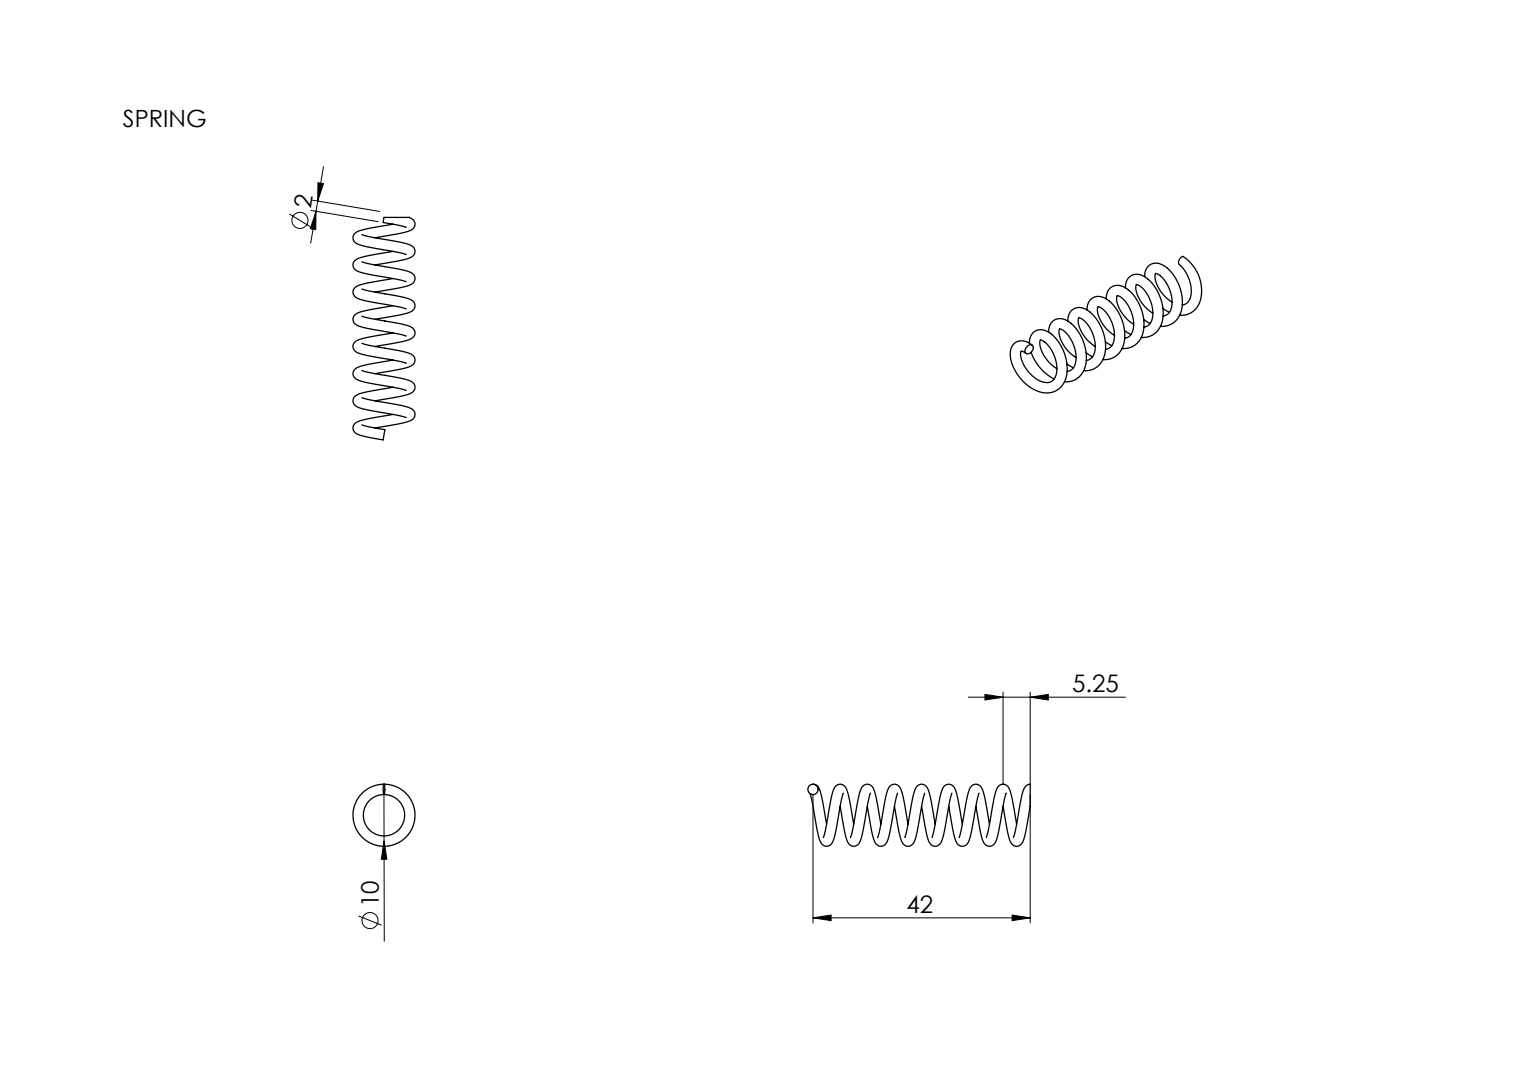
ISO-10303-21;
HEADER;
FILE_DESCRIPTION (('STEP AP214'),
    '1' );
FILE_NAME ('spring.step',
    '2026-10-08T14:41:38',
    ( '' ),
    ( '' ),
    'SwSTEP 2.0',
    'SolidWorks 2026',
    '' );
FILE_SCHEMA (( 'AUTOMOTIVE_DESIGN' ));
ENDSEC;

DATA;
#1=CARTESIAN_POINT ( 'NONE',  ( -12.68318583509882380, -26.07549068051207541, 23.95507249208304756 ) ) ;
#5=ORIENTED_EDGE ( 'NONE', *, *, #7068, .F. ) ;
#6=CARTESIAN_POINT ( 'NONE',  ( -14.83517299489738761, -20.99999999999997513, 4.263677507916960430 ) ) ;
#20=CARTESIAN_POINT ( 'NONE',  ( -16.17491895705301275, -18.95583473709189803, 14.54492750791695421 ) ) ;
#25=CARTESIAN_POINT ( 'NONE',  ( -17.64274437364858983, -19.75228648362910633, 21.54882249208304401 ) ) ;
#29=CARTESIAN_POINT ( 'NONE',  ( -17.35725562635140307, -28.41254052147349185, 40.79882249208304046 ) ) ;
#52=CARTESIAN_POINT ( 'NONE',  ( -10.75228648362910100, -26.64274437364854009, 6.013677507916958653 ) ) ;
#53=CARTESIAN_POINT ( 'NONE',  ( -19.41254052147348830, -26.35725562635142083, 18.26367750791695599 ) ) ;
#55=CARTESIAN_POINT ( 'NONE',  ( -13.49542703274174116, -28.95583473709188738, 3.392572492083040903 ) ) ;
#59=CARTESIAN_POINT ( 'NONE',  ( -13.82508104294698192, -29.04416526290806644, 1.419927507916958209 ) ) ;
#61=CARTESIAN_POINT ( 'NONE',  ( -15.16482700510259640, -28.99999999999998224, 1.638677507916958431 ) ) ;
#74=CARTESIAN_POINT ( 'NONE',  ( -7.999999999999996447, -23.83517299489733432, 23.29882249208304046 ) ) ;
#79=CARTESIAN_POINT ( 'NONE',  ( -15.63902057219076269, -20.95583473709189448, 9.294927507916961318 ) ) ;
#81=CARTESIAN_POINT ( 'NONE',  ( -21.14459132904239169, -20.64274437364858628, 5.361322492083039570 ) ) ;
#90=CARTESIAN_POINT ( 'NONE',  ( -15.00000000000001066, -19.99999999999997868, -4.814824860968089633E-32 ) ) ;
#98=CARTESIAN_POINT ( 'NONE',  ( -9.754982604823348780, -18.99630608921234654, 15.41992750791695777 ) ) ;
#103=CARTESIAN_POINT ( 'NONE',  ( -14.83517299489736985, -26.99999999999998579, 24.61132249208304756 ) ) ;
#107=CARTESIAN_POINT ( 'NONE',  ( -11.99999999999999289, -24.16482700510258752, 16.07617750791696309 ) ) ;
#119=PLANE ( 'NONE',  #7046 ) ;
#120=CARTESIAN_POINT ( 'NONE',  ( -19.95583473709191580, -22.49542703274176603, 13.66992750791695599 ) ) ;
#123=CARTESIAN_POINT ( 'NONE',  ( -16.50457296725825174, -19.04416526290807354, 16.51757249208304046 ) ) ;
#126=CARTESIAN_POINT ( 'NONE',  ( -14.83517299489736985, -26.99999999999998579, 19.36132249208304046 ) ) ;
#129=CARTESIAN_POINT ( 'NONE',  ( -11.21456601361727046, -19.57682413056721416, 1.010946030696228434E-16 ) ) ;
#144=CARTESIAN_POINT ( 'NONE',  ( -17.35725562635144215, -19.58745947852648683, 19.57617750791695954 ) ) ;
#146=CARTESIAN_POINT ( 'NONE',  ( -17.35725562635144215, -19.58745947852648683, 9.076177507916957765 ) ) ;
#149=CARTESIAN_POINT ( 'NONE',  ( -20.24501739517669563, -18.99630608921239627, 42.33007249208303335 ) ) ;
#151=CARTESIAN_POINT ( 'NONE',  ( -10.58745947852649927, -21.64274437364853654, -0.1113224920830418047 ) ) ;
#153=CARTESIAN_POINT ( 'NONE',  ( -12.35725562635143682, -19.75228648362908501, 20.45117750791695954 ) ) ;
#170=CARTESIAN_POINT ( 'NONE',  ( -22.04416526290809486, -22.28918265808477628, 15.64257249208304223 ) ) ;
#175=CARTESIAN_POINT ( 'NONE',  ( -18.04416526290808420, -24.63902057219074493, 18.48242750791695954 ) ) ;
#177=CARTESIAN_POINT ( 'NONE',  ( -7.999999999999996447, -23.83517299489733432, 7.548822492083037794 ) ) ;
#198=CARTESIAN_POINT ( 'NONE',  ( -20.97976432393977575, -20.35725562635143504, 13.88867750791695599 ) ) ;
#202=CARTESIAN_POINT ( 'NONE',  ( -13.64274437364857739, -21.31951028609534760, 11.92382249208304401 ) ) ;
#206=CARTESIAN_POINT ( 'NONE',  ( -15.96867458239597326, -26.95583473709190159, 17.60742750791696309 ) ) ;
#222=CARTESIAN_POINT ( 'NONE',  ( -10.04416526290807710, -25.50457296725819489, 21.54492750791695599 ) ) ;
#226=CARTESIAN_POINT ( 'NONE',  ( -19.95583473709190514, -25.50457296725822687, 15.20507249208304046 ) ) ;
#228=CARTESIAN_POINT ( 'NONE',  ( -17.07549068051208963, -26.31681416490115311, 25.26757249208305112 ) ) ;
#235=( BOUNDED_CURVE ( )  B_SPLINE_CURVE ( 2, ( #4277, #17906, #10238, #11607, #11805, #16129, #13075, #8674, #61, #14656, #4180, #7208, #16424, #14762, #1334, #10042, #1227, #16223, #2599, #7501, #2989, #1531, #2897, #2794, #14856, #14957, #8970, #6044, #13479, #16039, #8872, #13181, #1431, #8580, #19173, #17497, #1133, #19368, #4075, #5744, #11704, #5939, #14561, #7112, #8771, #7304, #13271, #5844, #17801, #4375, #10334, #11910, #16330, #7406, #18202, #8002, #16628, #18399, #15345, #16823, #3194, #18000, #9264, #6339, #12200, #9460, #9170, #1636, #352, #13969, #13671, #4779, #250, #10531, #6235, #18299, #7607, #12304, #1822, #4965, #10729, #542, #12001, #16524, #4867, #7801, #13772, #4574, #15251, #3386, #10827, #16725, #6140, #9355, #153, #1924, #7907, #15154, #3087, #9070, #13872, #10922, #3294, #16922, #447, #1723, #6432, #3485, #12399, #7704, #15446, #2013, #15057, #13572, #12101, #18097, #4670, #10626, #2113, #12596, #918, #14165, #17022, #6900, #17387, #6629, #11203, #15918, #2390, #3579, #9551, #5251, #14345, #2299, #5064, #17112, #8376, #3772, #12683, #18872, #12873, #18494, #17302, #3676, #3864, #15543, #8198, #8469, #8097, #5437, #3961, #18587, #14066, #8283, #9921, #14253, #638, #825, #11393, #17207, #9830, #2481, #734, #14445, #6528, #15823, #18686, #12493, #11115, #11020, #5154, #11304, #9646, #15633, #2205, #6808, #6713, #9745, #15737, #5341, #12773, #18769, #2674, #1205, #8657, #18960, #14638, #7289, #16022 ),
 .UNSPECIFIED., .F., .F. ) 
 B_SPLINE_CURVE_WITH_KNOTS ( ( 3, 2, 2, 2, 2, 2, 2, 2, 2, 2, 2, 2, 2, 2, 2, 2, 2, 2, 2, 2, 2, 2, 2, 2, 2, 2, 2, 2, 2, 2, 2, 2, 2, 2, 2, 2, 2, 2, 2, 2, 2, 2, 2, 2, 2, 2, 2, 2, 2, 2, 2, 2, 2, 2, 2, 2, 2, 2, 2, 2, 2, 2, 2, 2, 2, 2, 2, 2, 2, 2, 2, 2, 2, 2, 2, 2, 2, 2, 2, 2, 2, 2, 2, 2, 2, 2, 2, 2, 2, 2, 2, 2, 2, 2, 3 ),
 ( 0.02351720863160803449, 0.03125000000000000000, 0.04166666666666666435, 0.05208333333333333565, 0.06250000000000000000, 0.07291666666666665741, 0.08333333333333332871, 0.09375000000000000000, 0.1041666666666666574, 0.1145833333333333148, 0.1250000000000000000, 0.1354166666666666574, 0.1458333333333333426, 0.1562500000000000000, 0.1666666666666666574, 0.1770833333333333426, 0.1875000000000000000, 0.1979166666666666574, 0.2083333333333333426, 0.2187500000000000000, 0.2291666666666666574, 0.2395833333333333426, 0.2500000000000000000, 0.2604166666666666852, 0.2708333333333333148, 0.2812500000000000000, 0.2916666666666666852, 0.3020833333333333148, 0.3125000000000000000, 0.3229166666666666852, 0.3333333333333333148, 0.3437500000000000000, 0.3541666666666666852, 0.3645833333333333148, 0.3750000000000000000, 0.3854166666666666852, 0.3958333333333333148, 0.4062500000000000000, 0.4166666666666666852, 0.4270833333333333148, 0.4375000000000000000, 0.4479166666666666852, 0.4583333333333333148, 0.4687500000000000000, 0.4791666666666666852, 0.4895833333333333148, 0.5000000000000000000, 0.5104166666666666297, 0.5208333333333333703, 0.5312500000000000000, 0.5416666666666666297, 0.5520833333333333703, 0.5625000000000000000, 0.5729166666666666297, 0.5833333333333333703, 0.5937500000000000000, 0.6041666666666666297, 0.6145833333333333703, 0.6250000000000000000, 0.6354166666666666297, 0.6458333333333333703, 0.6562500000000000000, 0.6666666666666666297, 0.6770833333333333703, 0.6875000000000000000, 0.6979166666666666297, 0.7083333333333333703, 0.7187500000000000000, 0.7291666666666666297, 0.7395833333333333703, 0.7500000000000000000, 0.7604166666666666297, 0.7708333333333333703, 0.7812500000000000000, 0.7916666666666666297, 0.8020833333333333703, 0.8125000000000000000, 0.8229166666666666297, 0.8333333333333333703, 0.8437500000000000000, 0.8541666666666666297, 0.8645833333333333703, 0.8750000000000000000, 0.8854166666666666297, 0.8958333333333333703, 0.9062500000000000000, 0.9166666666666666297, 0.9270833333333333703, 0.9375000000000000000, 0.9479166666666666297, 0.9583333333333333703, 0.9687500000000000000, 0.9791666666666666297, 0.9895833333333333703, 1.000000000000000000 ),
 .UNSPECIFIED. ) 
 CURVE ( )  GEOMETRIC_REPRESENTATION_ITEM ( )  RATIONAL_B_SPLINE_CURVE ( ( 0.9869654386326103257, 0.9747051062697298374, 1.000000000000000000, 0.9659258262890683122, 1.000000000000000000, 0.9659258262890683122, 1.000000000000000000, 0.9659258262890683122, 1.000000000000000000, 0.9659258262890683122, 1.000000000000000000, 0.9659258262890683122, 1.000000000000000000, 0.9659258262890683122, 1.000000000000000000, 0.9659258262890683122, 1.000000000000000000, 0.9659258262890683122, 1.000000000000000000, 0.9659258262890683122, 1.000000000000000000, 0.9659258262890683122, 1.000000000000000000, 0.9659258262890683122, 1.000000000000000000, 0.9659258262890683122, 1.000000000000000000, 0.9659258262890683122, 1.000000000000000000, 0.9659258262890683122, 1.000000000000000000, 0.9659258262890683122, 1.000000000000000000, 0.9659258262890683122, 1.000000000000000000, 0.9659258262890683122, 1.000000000000000000, 0.9659258262890683122, 1.000000000000000000, 0.9659258262890683122, 1.000000000000000000, 0.9659258262890683122, 1.000000000000000000, 0.9659258262890683122, 1.000000000000000000, 0.9659258262890683122, 1.000000000000000000, 0.9659258262890683122, 1.000000000000000000, 0.9659258262890683122, 1.000000000000000000, 0.9659258262890683122, 1.000000000000000000, 0.9659258262890683122, 1.000000000000000000, 0.9659258262890683122, 1.000000000000000000, 0.9659258262890683122, 1.000000000000000000, 0.9659258262890683122, 1.000000000000000000, 0.9659258262890683122, 1.000000000000000000, 0.9659258262890683122, 1.000000000000000000, 0.9659258262890683122, 1.000000000000000000, 0.9659258262890683122, 1.000000000000000000, 0.9659258262890683122, 1.000000000000000000, 0.9659258262890683122, 1.000000000000000000, 0.9659258262890683122, 1.000000000000000000, 0.9659258262890683122, 1.000000000000000000, 0.9659258262890683122, 1.000000000000000000, 0.9659258262890683122, 1.000000000000000000, 0.9659258262890683122, 1.000000000000000000, 0.9659258262890683122, 1.000000000000000000, 0.9659258262890683122, 1.000000000000000000, 0.9659258262890683122, 1.000000000000000000, 0.9659258262890683122, 1.000000000000000000, 0.9659258262890683122, 1.000000000000000000, 0.9659258262890683122, 1.000000000000000000, 0.9659258262890683122, 1.000000000000000000, 0.9659258262890683122, 1.000000000000000000, 0.9659258262890683122, 1.000000000000000000, 0.9659258262890683122, 1.000000000000000000, 0.9659258262890683122, 1.000000000000000000, 0.9659258262890683122, 1.000000000000000000, 0.9659258262890683122, 1.000000000000000000, 0.9659258262890683122, 1.000000000000000000, 0.9659258262890683122, 1.000000000000000000, 0.9659258262890683122, 1.000000000000000000, 0.9659258262890683122, 1.000000000000000000, 0.9659258262890683122, 1.000000000000000000, 0.9659258262890683122, 1.000000000000000000, 0.9659258262890683122, 1.000000000000000000, 0.9659258262890683122, 1.000000000000000000, 0.9659258262890683122, 1.000000000000000000, 0.9659258262890683122, 1.000000000000000000, 0.9659258262890683122, 1.000000000000000000, 0.9659258262890683122, 1.000000000000000000, 0.9659258262890683122, 1.000000000000000000, 0.9659258262890683122, 1.000000000000000000, 0.9659258262890683122, 1.000000000000000000, 0.9659258262890683122, 1.000000000000000000, 0.9659258262890683122, 1.000000000000000000, 0.9659258262890683122, 1.000000000000000000, 0.9659258262890683122, 1.000000000000000000, 0.9659258262890683122, 1.000000000000000000, 0.9659258262890683122, 1.000000000000000000, 0.9659258262890683122, 1.000000000000000000, 0.9659258262890683122, 1.000000000000000000, 0.9659258262890683122, 1.000000000000000000, 0.9659258262890683122, 1.000000000000000000, 0.9659258262890683122, 1.000000000000000000, 0.9659258262890683122, 1.000000000000000000, 0.9659258262890683122, 1.000000000000000000, 0.9659258262890683122, 1.000000000000000000, 0.9659258262890683122, 1.000000000000000000, 0.9659258262890683122, 1.000000000000000000, 0.9659258262890683122, 1.000000000000000000, 0.9659258262890683122, 1.000000000000000000, 0.9659258262890683122, 1.000000000000000000, 0.9659258262890683122, 1.000000000000000000, 0.9659258262890683122, 1.000000000000000000, 0.9659258262890683122, 1.000000000000000000, 0.9659258262890683122, 1.000000000000000000, 0.9659258262890683122, 1.000000000000000000, 0.9659258262890683122, 1.000000000000000000 ) ) 
 REPRESENTATION_ITEM ( '' )  );
#244=CARTESIAN_POINT ( 'NONE',  ( -13.82508104294698192, -29.04416526290806644, 11.91992750791695421 ) ) ;
#246=CARTESIAN_POINT ( 'NONE',  ( -20.04416526290809131, -22.82508104294699791, 20.89257249208303691 ) ) ;
#248=CARTESIAN_POINT ( 'NONE',  ( -10.75228648362910100, -26.64274437364854009, 11.26367750791695777 ) ) ;
#250=CARTESIAN_POINT ( 'NONE',  ( -10.58745947852649927, -21.64274437364853654, 15.63867750791695777 ) ) ;
#263=CARTESIAN_POINT ( 'NONE',  ( -14.83517299489734853, -30.99999999999998224, 19.36132249208304046 ) ) ;
#264=CARTESIAN_POINT ( 'NONE',  ( -9.955834737091903364, -25.17491895705295235, 7.767572492083041347 ) ) ;
#266=CARTESIAN_POINT ( 'NONE',  ( -14.83517299489738761, -20.99999999999997513, 14.76367750791695954 ) ) ;
#268=CARTESIAN_POINT ( 'NONE',  ( -7.999999999999996447, -23.83517299489733432, 18.04882249208304046 ) ) ;
#288=CARTESIAN_POINT ( 'NONE',  ( -11.64274437364854187, -30.14459132904234195, 16.95117750791695954 ) ) ;
#293=CARTESIAN_POINT ( 'NONE',  ( -14.83517299489736985, -26.99999999999998579, 14.11132249208304223 ) ) ;
#294=CARTESIAN_POINT ( 'NONE',  ( -16.71081734191527346, -16.95583473709190159, 9.294927507916959541 ) ) ;
#298=CARTESIAN_POINT ( 'NONE',  ( -16.35725562635142794, -21.31951028609535470, 14.32617750791695777 ) ) ;
#321=CARTESIAN_POINT ( 'NONE',  ( -13.82508104294698192, -29.04416526290806644, 11.91992750791695421 ) ) ;
#325=CARTESIAN_POINT ( 'NONE',  ( -19.41254052147350961, -21.64274437364857562, 21.11132249208304401 ) ) ;
#328=CARTESIAN_POINT ( 'NONE',  ( -15.63902057219073605, -27.04416526290807710, 19.58007249208304046 ) ) ;
#337=CARTESIAN_POINT ( 'NONE',  ( -15.00000000000001421, -18.99999999999997868, 42.00000000000000000 ) ) ;
#346=CARTESIAN_POINT ( 'NONE',  ( -13.82508104294698192, -29.04416526290806644, 17.16992750791694888 ) ) ;
#348=CARTESIAN_POINT ( 'NONE',  ( -11.21908421996106320, -27.53959229564982181, 23.95507249208304401 ) ) ;
#350=CARTESIAN_POINT ( 'NONE',  ( -17.64274437364855430, -28.24771351637087236, 23.07617750791695954 ) ) ;
#352=CARTESIAN_POINT ( 'NONE',  ( -14.83517299489739649, -18.99999999999997868, 14.76367750791695777 ) ) ;
#365=CARTESIAN_POINT ( 'NONE',  ( -9.020235676060250896, -20.35725562635137820, 38.61132249208304046 ) ) ;
#367=CARTESIAN_POINT ( 'NONE',  ( -12.64274437364858628, -19.58745947852646552, 6.673822492083040459 ) ) ;
#369=CARTESIAN_POINT ( 'NONE',  ( -16.64274437364856496, -26.51566270880199738, 23.07617750791695954 ) ) ;
#371=CARTESIAN_POINT ( 'NONE',  ( -21.95583473709189803, -26.04047135212049469, 15.20507249208304046 ) ) ;
#392=CARTESIAN_POINT ( 'NONE',  ( -8.855408670957631401, -20.64274437364852943, 26.13867750791696309 ) ) ;
#396=CARTESIAN_POINT ( 'NONE',  ( -14.03132541760400009, -26.95583473709189448, 13.89257249208304401 ) ) ;
#397=CARTESIAN_POINT ( 'NONE',  ( -8.044165262908075320, -26.04047135212042718, 11.04492750791695777 ) ) ;
#402=CARTESIAN_POINT ( 'NONE',  ( -12.04416526290807887, -24.96867458239596260, 11.04492750791696132 ) ) ;
#416=CARTESIAN_POINT ( 'NONE',  ( -19.99999999999999645, -23.83517299489738051, 13.45117750791695777 ) ) ;
#422=CARTESIAN_POINT ( 'NONE',  ( -10.75228648362912232, -21.35725562635138530, 22.86132249208304401 ) ) ;
#424=CARTESIAN_POINT ( 'NONE',  ( -11.95583473709190514, -24.63902057219072361, 18.26757249208304401 ) ) ;
#441=CARTESIAN_POINT ( 'NONE',  ( -10.58745947852649927, -21.64274437364853654, 20.88867750791695954 ) ) ;
#443=CARTESIAN_POINT ( 'NONE',  ( -17.35725562635140307, -28.41254052147349185, 19.79882249208304046 ) ) ;
#445=CARTESIAN_POINT ( 'NONE',  ( -18.53959229564986799, -20.21908421996107563, 14.10742750791695777 ) ) ;
#447=CARTESIAN_POINT ( 'NONE',  ( -15.16482700510259640, -28.99999999999998224, 22.63867750791695954 ) ) ;
#449=CARTESIAN_POINT ( 'NONE',  ( -18.78091578003892792, -20.46040770435013556, 31.83007249208304046 ) ) ;
#460=CARTESIAN_POINT ( 'NONE',  ( -11.35725562635139418, -29.97976432393972601, 29.42382249208304046 ) ) ;
#461=CARTESIAN_POINT ( 'NONE',  ( -18.53959229564983247, -27.78091578003891016, 9.517572492083040459 ) ) ;
#463=CARTESIAN_POINT ( 'NONE',  ( -16.64274437364856496, -26.51566270880199738, 33.57617750791696665 ) ) ;
#465=CARTESIAN_POINT ( 'NONE',  ( -12.95952864787948755, -30.95583473709188382, 24.39257249208303691 ) ) ;
#483=CARTESIAN_POINT ( 'NONE',  ( -8.044165262908075320, -26.04047135212042718, 32.04492750791695954 ) ) ;
#488=CARTESIAN_POINT ( 'NONE',  ( -15.63902057219073605, -27.04416526290807710, 24.83007249208304046 ) ) ;
#489=CARTESIAN_POINT ( 'NONE',  ( -13.28918265808472299, -31.04416526290805933, 17.16992750791696309 ) ) ;
#493=CARTESIAN_POINT ( 'NONE',  ( -14.03132541760401786, -21.04416526290806289, 20.23242750791696309 ) ) ;
#511=CARTESIAN_POINT ( 'NONE',  ( -10.75228648362910100, -26.64274437364854009, 27.01367750791695954 ) ) ;
#514=CARTESIAN_POINT ( 'NONE',  ( -19.99999999999999645, -24.16482700510261949, 31.17382249208304046 ) ) ;
#517=CARTESIAN_POINT ( 'NONE',  ( -11.95583473709190514, -24.63902057219072361, 23.51757249208304401 ) ) ;
#518=( BOUNDED_SURFACE ( )  B_SPLINE_SURFACE ( 3, 2, ( 
 ( #10197, #8455, #1007, #8641, #5511, #1394, #8550, #16095, #7170, #18945, #11476, #16192, #7369, #4038, #13143, #17663, #4241, #14624, #5610, #1301, #10003, #13339, #19237, #13041, #2466, #2757, #16287, #17570, #11770, #14826, #4148, #16007, #19338, #10099, #2567, #14524, #10294, #11867, #9911, #1095, #14431, #14723, #17765, #17867, #7276, #13241, #5804, #2861, #15904, #18066, #15222, #7670, #9231, #7571, #4441, #6403, #13542, #16590, #18166, #321, #14925, #4838, #6304, #4741, #17965, #4641, #416, #120, #12368, #9326, #6104, #20, #1790, #1597, #16393, #18270, #10399, #12068, #12274, #13738, #3158, #10594, #3259, #9138, #13436, #15021, #10791, #3361, #7773, #16790, #2957, #12167, #6009, #15122, #8933, #7467, #13843, #16695, #7876, #1690, #15313, #13637, #1498, #222, #11971, #6207, #4539, #10699, #1891, #10495, #16492, #3056, #9032, #17174, #603, #18655, #16887, #9427, #17082, #13938, #9800, #16993, #5131, #9616, #15422, #1986, #5220, #15794, #511, #15602, #14133, #8160, #11084, #8071, #9709, #12461, #2360, #8257, #15509, #10892, #6688, #5306, #14032, #794, #3834, #6596, #6498, #8343, #2082, #18459, #5029, #12744, #14315, #18366, #10989, #3453, #3552, #6779, #882, #2171, #3736, #708, #7970, #12566, #18563, #15702, #12654, #2271, #3644, #4935, #6861, #11174, #14225, #18740, #11266, #9520, #17267, #14502, #1275, #14698, #19022, #1074, #1373, #14604, #5587, #13022, #17447, #16264, #7254, #4017, #18923, #5690, #2634 ),
 ( #13221, #4123, #17544, #5781, #7053, #11650, #8528, #9979, #11549, #2836, #14406, #10079, #16073, #8819, #14805, #12835, #19118, #8620, #5405, #17353, #8710, #19213, #1171, #11743, #2446, #7149, #15983, #17640, #17740, #13119, #18833, #4216, #8430, #10171, #4315, #10271, #16170, #983, #11360, #2739, #3924, #9892, #15885, #6959, #12929, #5492, #11455, #2545, #16763, #6185, #18136, #3130, #16371, #16564, #7645, #16668, #14993, #3032, #1570, #10762, #1671, #9109, #15099, #13612, #12044, #15287, #17841, #9009, #198, #7544, #7748, #13519, #7342, #3233, #16467, #98, #6080, #4415, #4714, #4814, #10668, #12142, #288, #19313, #15194, #3335, #1765, #10377, #9206, #18239, #7443, #5982, #13410, #10570, #13712, #6274, #18043, #4616, #12244, #9303, #13313, #11841, #5880, #2935, #8910, #14899, #1474, #6085, #11951, #17943, #4515, #10472, #9584, #16964, #10866, #12437, #17143, #764, #679, #9679, #13811, #15577, #16861, #14003, #392, #4908, #11234, #14103, #5275, #2047, #6745, #15481, #3807, #8042, #7847, #5102, #15391, #10960, #2241, #18534, #1959, #3706, #15672, #6662, #3526, #2144, #6375, #12338, #575, #3423, #12716, #483, #6564, #12533, #18336, #9396, #8131, #18713, #7945, #11056, #17052, #3615, #12627, #9492, #18622, #13905, #17239, #11148, #18433, #6470, #5187, #8232, #14197, #9773, #1860, #5002, #3895, #13194, #18900, #17328, #15860, #10143, #11716, #15768, #9862, #14287, #2419, #17613, #17710, #18995, #1146, #11518, #5378 ),
 ( #2331, #4291, #14476, #5463, #2608, #12991, #8314, #9950, #17422, #4190, #16142, #2515, #3992, #855, #17511, #11426, #8499, #10052, #11622, #6834, #2712, #8685, #16048, #8402, #15950, #12803, #1047, #18803, #1243, #7024, #11336, #13089, #12903, #14375, #14668, #951, #5560, #7223, #5659, #4090, #8592, #14573, #6933, #7123, #19089, #19187, #5754, #6154, #1346, #10641, #12116, #4586, #4389, #10445, #6247, #5953, #18216, #15169, #13386, #5856, #7621, #7419, #2808, #4683, #16235, #11924, #18110, #170, #3002, #19381, #9085, #17918, #19284, #1442, #16644, #9183, #15073, #3209, #8786, #18013, #11817, #8982, #14777, #13283, #263, #3102, #13685, #16437, #1737, #4491, #12214, #14969, #7317, #13492, #10347, #1542, #7720, #7517, #16345, #10248, #17812, #1648, #74, #10545, #2909, #8883, #6054, #14870, #12016, #16535, #13585, #15457, #1834, #7815, #11033, #2470, #6353, #2026, #554, #13982, #16936, #13884, #15555, #18312, #8460, #14078, #1937, #16738, #12506, #11127, #460, #6642, #9657, #6445, #12316, #14435, #7920, #4880, #10840, #18599, #1010, #4792, #16835, #3307, #3400, #12606, #6985, #8016, #9562, #6541, #13785, #18410, #4977, #2125, #18509, #8109, #12412, #10741, #12951, #3501, #10935, #17033, #5076, #9276, #9471, #3591, #5166, #17123, #651, #3687, #15647, #15265, #365, #9367, #15361, #17667, #8646, #5809, #16195, #5517, #13148, #1192, #7373, #1398, #5717, #7174, #7470, #1305, #2664, #11676, #13244, #14829, #10007 ),
 ( #8936, #17768, #10298, #14727, #8553, #8735, #19241, #8844, #19145, #14628, #4244, #2960, #11776, #7279, #4342, #16292, #10204, #18949, #16012, #2762, #2864, #13347, #19341, #5907, #11479, #11872, #17871, #4444, #10402, #2571, #16396, #14931, #1503, #17467, #4042, #14528, #1098, #7081, #13044, #19043, #5614, #11577, #17574, #4153, #10103, #16099, #6308, #12279, #7674, #4747, #9234, #10796, #16698, #17968, #16891, #16793, #4841, #12372, #7575, #18370, #9141, #1602, #9432, #3365, #1795, #226, #13640, #18071, #3457, #7880, #4644, #123, #18274, #3263, #7776, #6406, #6210, #3163, #12171, #15425, #13846, #10702, #18171, #4940, #15126, #9329, #1693, #10598, #15225, #1989, #15026, #13741, #325, #13440, #25, #6012, #15316, #1894, #11974, #4542, #422, #13545, #10498, #10897, #16498, #3060, #9038, #16595, #6108, #12071, #18566, #14036, #797, #17177, #2275, #886, #8164, #17085, #6691, #3927, #2363, #18658, #12658, #6866, #9620, #6782, #3649, #5134, #5223, #17358, #9524, #15606, #711, #9895, #11363, #15888, #14229, #3740, #514, #12464, #3838, #8346, #11179, #14318, #16996, #9713, #11088, #12748, #12838, #15706, #7975, #18745, #3555, #5309, #18838, #5408, #8261, #15514, #13941, #17271, #11270, #6503, #9804, #18464, #2085, #5033, #10994, #8074, #606, #15798, #6602, #12570, #2174, #14137, #2743, #11747, #10083, #17548, #16076, #5885, #16174, #4221, #10176, #8715, #7153, #10382, #12932, #4128, #14702, #2640, #2841, #8623, #2450 ),
 ( #19317, #5787, #1280, #14809, #14411, #10276, #11846, #16269, #5495, #4319, #13318, #2550, #1078, #8532, #5695, #7258, #13225, #14607, #13122, #17645, #19217, #11654, #6963, #17846, #17745, #8824, #1377, #15987, #7348, #8433, #4420, #11552, #1174, #19122, #18927, #987, #11458, #17450, #4021, #9982, #14506, #7056, #13025, #19025, #5591, #18244, #7851, #16471, #14998, #3036, #202, #9209, #15201, #10574, #7650, #12146, #13716, #6189, #1478, #396, #293, #7751, #15292, #10478, #1865, #12050, #4519, #12342, #6278, #4718, #3135, #16569, #1575, #6378, #10765, #7549, #9013, #1769, #18141, #10673, #9307, #9114, #6084, #15104, #18341, #16768, #13616, #1674, #13817, #18048, #12248, #4621, #13524, #16674, #4911, #17947, #3237, #4818, #16375, #2939, #8915, #3339, #14903, #7447, #13415, #1, #5987, #11956, #103, #488, #12631, #2053, #17148, #5279, #6666, #18809, #9685, #6474, #8236, #3812, #15772, #14109, #12441, #859, #768, #15677, #10870, #2247, #14292, #18437, #3428, #6838, #5006, #12809, #14202, #6752, #18627, #10964, #684, #11152, #12720, #18538, #6572, #5106, #16865, #5194, #3711, #18717, #11239, #15581, #9400, #1962, #12538, #17243, #11060, #9779, #17056, #2335, #8321, #16969, #15395, #7948, #13909, #3529, #9496, #15485, #8046, #14008, #579, #3621, #9589, #2148, #8136, #1151, #14382, #14580, #5664, #14674, #12999, #1052, #19000, #8793, #19094, #7128, #13094, #11628, #10057, #13288, #15864, #7029, #17618, #5565, #5759 ),
 ( #2424, #16149, #2814, #8691, #4195, #17718, #17333, #13198, #14782, #19192, #8407, #7229, #16241, #5468, #3997, #11433, #8596, #10147, #2718, #11523, #16052, #1249, #11721, #4295, #9869, #1351, #10252, #7323, #5383, #18904, #11341, #17517, #12908, #3900, #956, #6938, #4097, #2612, #9955, #17426, #15957, #2522, #8503, #14481, #9089, #13590, #12218, #79, #8987, #18018, #15268, #13690, #10551, #4593, #18219, #1548, #18116, #14974, #16442, #16540, #9282, #1450, #7523, #12022, #1837, #3311, #7821, #6161, #15078, #11821, #4395, #15175, #266, #3108, #6252, #8888, #1652, #10450, #12121, #4796, #7626, #19291, #4688, #14876, #16649, #10745, #6059, #13497, #5861, #175, #3010, #10646, #3214, #1742, #10355, #16742, #7727, #9187, #13390, #17817, #16349, #2914, #7423, #19386, #5959, #11930, #17923, #4495, #6357, #8213, #369, #9474, #2221, #3689, #6545, #3505, #12609, #15460, #3403, #4982, #9659, #12695, #18603, #14181, #12320, #2127, #9372, #12512, #18316, #16841, #3790, #6644, #17221, #13987, #18699, #8020, #15750, #557, #4884, #17036, #7924, #2029, #746, #11037, #13887, #15651, #6728, #5168, #18513, #14082, #10846, #15367, #5080, #1940, #5261, #12418, #3593, #9564, #463, #6449, #657, #11215, #18415, #15559, #8111, #11129, #17127, #9757, #2312, #10939, #13789, #16942, #5448, #838, #16034, #14650, #3976, #10126, #13174, #9933, #15839, #5739, #11407, #9843, #8385, #2692, #4270, #8296, #2403, #6819, #14358, #16123, #10232 ),
 ( #12786, #18783, #4175, #8668, #7008, #1220, #17313, #10036, #18886, #14554, #7202, #4068, #16216, #7106, #3876, #19168, #15930, #13069, #2496, #17402, #12976, #17692, #933, #8483, #1033, #14268, #11699, #5359, #1125, #2593, #11319, #6914, #12887, #14460, #18975, #5545, #11501, #8575, #17491, #19067, #5640, #11601, #17598, #17992, #5836, #16518, #146, #12093, #14952, #11800, #10620, #9062, #4566, #9162, #10523, #4663, #17794, #8765, #16621, #4367, #3188, #3081, #15050, #7494, #19267, #1525, #6037, #1628, #5930, #13370, #11901, #2787, #11994, #7598, #13565, #6131, #8962, #14755, #10327, #17899, #18091, #10422, #1329, #16417, #7299, #13266, #13470, #16324, #53, #19362, #2891, #8866, #14851, #1424, #7399, #2982, #4471, #4336, #14719, #3942, #2755, #11766, #1002, #18942, #6978, #4146, #13140, #19139, #14520, #11569, #16090, #17660, #10097, #5421, #10292, #4237, #11670, #19234, #14428, #5803, #16005, #8452, #16285, #10195, #8639, #7073, #1093, #5508, #2858, #1299, #11473, #12944, #5712, #2658, #14622, #13239, #13039, #10000, #19037, #8838, #7274, #17567, #5608, #900, #17763, #4035, #15900, #16190, #17462, #12854, #6881, #18856, #11377, #1187, #7168, #8729, #17369, #9908, #2464, #2565, #8546, #16588, #9030, #15219, #15017, #3358, #10694, #4536, #7569, #16490, #11865, #6205, #12271, #18163, #3154, #7770, #7367, #3256, #18265, #9227, #17865, #16691, #6301, #14923, #13433, #1496, #18064, #7667, #13635, #1594, #6101, #10592, #12164 ) ),
 .UNSPECIFIED., .T., .F., .F. ) 
 B_SPLINE_SURFACE_WITH_KNOTS ( ( 4, 3, 4 ),
 ( 3, 2, 2, 2, 2, 2, 2, 2, 2, 2, 2, 2, 2, 2, 2, 2, 2, 2, 2, 2, 2, 2, 2, 2, 2, 2, 2, 2, 2, 2, 2, 2, 2, 2, 2, 2, 2, 2, 2, 2, 2, 2, 2, 2, 2, 2, 2, 2, 2, 2, 2, 2, 2, 2, 2, 2, 2, 2, 2, 2, 2, 2, 2, 2, 2, 2, 2, 2, 2, 2, 2, 2, 2, 2, 2, 2, 2, 2, 2, 2, 2, 2, 2, 2, 2, 2, 2, 2, 2, 2, 2, 2, 2, 2, 2, 2, 3 ),
 ( 0.000000000000000000, 0.5000000000000000000, 1.000000000000000000 ),
 ( 0.000000000000000000, 0.01041666666666666609, 0.02083333333333333218, 0.03125000000000000000, 0.04166666666666666435, 0.05208333333333333565, 0.06250000000000000000, 0.07291666666666667129, 0.08333333333333332871, 0.09375000000000000000, 0.1041666666666666713, 0.1145833333333333287, 0.1250000000000000000, 0.1354166666666666574, 0.1458333333333333426, 0.1562500000000000000, 0.1666666666666666574, 0.1770833333333333426, 0.1875000000000000000, 0.1979166666666666574, 0.2083333333333333426, 0.2187500000000000000, 0.2291666666666666574, 0.2395833333333333426, 0.2500000000000000000, 0.2604166666666666852, 0.2708333333333333148, 0.2812500000000000000, 0.2916666666666666852, 0.3020833333333333148, 0.3125000000000000000, 0.3229166666666666852, 0.3333333333333333148, 0.3437500000000000000, 0.3541666666666666852, 0.3645833333333333148, 0.3750000000000000000, 0.3854166666666666852, 0.3958333333333333148, 0.4062500000000000000, 0.4166666666666666852, 0.4270833333333333148, 0.4375000000000000000, 0.4479166666666666852, 0.4583333333333333148, 0.4687500000000000000, 0.4791666666666666852, 0.4895833333333333148, 0.5000000000000000000, 0.5104166666666666297, 0.5208333333333333703, 0.5312500000000000000, 0.5416666666666666297, 0.5520833333333333703, 0.5625000000000000000, 0.5729166666666666297, 0.5833333333333333703, 0.5937500000000000000, 0.6041666666666666297, 0.6145833333333333703, 0.6250000000000000000, 0.6354166666666666297, 0.6458333333333333703, 0.6562500000000000000, 0.6666666666666666297, 0.6770833333333333703, 0.6875000000000000000, 0.6979166666666666297, 0.7083333333333333703, 0.7187500000000000000, 0.7291666666666666297, 0.7395833333333333703, 0.7500000000000000000, 0.7604166666666666297, 0.7708333333333333703, 0.7812500000000000000, 0.7916666666666666297, 0.8020833333333333703, 0.8125000000000000000, 0.8229166666666666297, 0.8333333333333333703, 0.8437500000000000000, 0.8541666666666666297, 0.8645833333333333703, 0.8750000000000000000, 0.8854166666666666297, 0.8958333333333333703, 0.9062500000000000000, 0.9166666666666666297, 0.9270833333333333703, 0.9375000000000000000, 0.9479166666666666297, 0.9583333333333333703, 0.9687500000000000000, 0.9791666666666666297, 0.9895833333333333703, 1.000000000000000000 ),
 .UNSPECIFIED. ) 
 GEOMETRIC_REPRESENTATION_ITEM ( )  RATIONAL_B_SPLINE_SURFACE ( (
 ( 1.000000000000000000, 0.9659258262890683122, 1.000000000000000000, 0.9659258262890683122, 1.000000000000000000, 0.9659258262890683122, 1.000000000000000000, 0.9659258262890683122, 1.000000000000000000, 0.9659258262890683122, 1.000000000000000000, 0.9659258262890683122, 1.000000000000000000, 0.9659258262890683122, 1.000000000000000000, 0.9659258262890683122, 1.000000000000000000, 0.9659258262890683122, 1.000000000000000000, 0.9659258262890683122, 1.000000000000000000, 0.9659258262890683122, 1.000000000000000000, 0.9659258262890683122, 1.000000000000000000, 0.9659258262890683122, 1.000000000000000000, 0.9659258262890683122, 1.000000000000000000, 0.9659258262890683122, 1.000000000000000000, 0.9659258262890683122, 1.000000000000000000, 0.9659258262890683122, 1.000000000000000000, 0.9659258262890683122, 1.000000000000000000, 0.9659258262890683122, 1.000000000000000000, 0.9659258262890683122, 1.000000000000000000, 0.9659258262890683122, 1.000000000000000000, 0.9659258262890683122, 1.000000000000000000, 0.9659258262890683122, 1.000000000000000000, 0.9659258262890683122, 1.000000000000000000, 0.9659258262890683122, 1.000000000000000000, 0.9659258262890683122, 1.000000000000000000, 0.9659258262890683122, 1.000000000000000000, 0.9659258262890683122, 1.000000000000000000, 0.9659258262890683122, 1.000000000000000000, 0.9659258262890683122, 1.000000000000000000, 0.9659258262890683122, 1.000000000000000000, 0.9659258262890683122, 1.000000000000000000, 0.9659258262890683122, 1.000000000000000000, 0.9659258262890683122, 1.000000000000000000, 0.9659258262890683122, 1.000000000000000000, 0.9659258262890683122, 1.000000000000000000, 0.9659258262890683122, 1.000000000000000000, 0.9659258262890683122, 1.000000000000000000, 0.9659258262890683122, 1.000000000000000000, 0.9659258262890683122, 1.000000000000000000, 0.9659258262890683122, 1.000000000000000000, 0.9659258262890683122, 1.000000000000000000, 0.9659258262890683122, 1.000000000000000000, 0.9659258262890683122, 1.000000000000000000, 0.9659258262890683122, 1.000000000000000000, 0.9659258262890683122, 1.000000000000000000, 0.9659258262890683122, 1.000000000000000000, 0.9659258262890683122, 1.000000000000000000, 0.9659258262890683122, 1.000000000000000000, 0.9659258262890683122, 1.000000000000000000, 0.9659258262890683122, 1.000000000000000000, 0.9659258262890683122, 1.000000000000000000, 0.9659258262890683122, 1.000000000000000000, 0.9659258262890683122, 1.000000000000000000, 0.9659258262890683122, 1.000000000000000000, 0.9659258262890683122, 1.000000000000000000, 0.9659258262890683122, 1.000000000000000000, 0.9659258262890683122, 1.000000000000000000, 0.9659258262890683122, 1.000000000000000000, 0.9659258262890683122, 1.000000000000000000, 0.9659258262890683122, 1.000000000000000000, 0.9659258262890683122, 1.000000000000000000, 0.9659258262890683122, 1.000000000000000000, 0.9659258262890683122, 1.000000000000000000, 0.9659258262890683122, 1.000000000000000000, 0.9659258262890683122, 1.000000000000000000, 0.9659258262890683122, 1.000000000000000000, 0.9659258262890683122, 1.000000000000000000, 0.9659258262890683122, 1.000000000000000000, 0.9659258262890683122, 1.000000000000000000, 0.9659258262890683122, 1.000000000000000000, 0.9659258262890683122, 1.000000000000000000, 0.9659258262890683122, 1.000000000000000000, 0.9659258262890683122, 1.000000000000000000, 0.9659258262890683122, 1.000000000000000000, 0.9659258262890683122, 1.000000000000000000, 0.9659258262890683122, 1.000000000000000000, 0.9659258262890683122, 1.000000000000000000, 0.9659258262890683122, 1.000000000000000000, 0.9659258262890683122, 1.000000000000000000, 0.9659258262890683122, 1.000000000000000000, 0.9659258262890683122, 1.000000000000000000, 0.9659258262890683122, 1.000000000000000000, 0.9659258262890683122, 1.000000000000000000, 0.9659258262890683122, 1.000000000000000000, 0.9659258262890683122, 1.000000000000000000, 0.9659258262890683122, 1.000000000000000000, 0.9659258262890683122, 1.000000000000000000, 0.9659258262890683122, 1.000000000000000000, 0.9659258262890683122, 1.000000000000000000, 0.9659258262890683122, 1.000000000000000000, 0.9659258262890683122, 1.000000000000000000, 0.9659258262890683122, 1.000000000000000000, 0.9659258262890683122, 1.000000000000000000, 0.9659258262890683122, 1.000000000000000000, 0.9659258262890683122, 1.000000000000000000),
 ( 0.3333333333333333703, 0.3219752754296894559, 0.3333333333333333703, 0.3219752754296894559, 0.3333333333333333703, 0.3219752754296894559, 0.3333333333333333703, 0.3219752754296894559, 0.3333333333333333703, 0.3219752754296894559, 0.3333333333333333703, 0.3219752754296894559, 0.3333333333333333703, 0.3219752754296894559, 0.3333333333333333703, 0.3219752754296894559, 0.3333333333333333703, 0.3219752754296894559, 0.3333333333333333703, 0.3219752754296894559, 0.3333333333333333703, 0.3219752754296894559, 0.3333333333333333703, 0.3219752754296894559, 0.3333333333333333703, 0.3219752754296894559, 0.3333333333333333703, 0.3219752754296894559, 0.3333333333333333703, 0.3219752754296894559, 0.3333333333333333703, 0.3219752754296894559, 0.3333333333333333703, 0.3219752754296894559, 0.3333333333333333703, 0.3219752754296894559, 0.3333333333333333703, 0.3219752754296894559, 0.3333333333333333703, 0.3219752754296894559, 0.3333333333333333703, 0.3219752754296894559, 0.3333333333333333703, 0.3219752754296894559, 0.3333333333333333703, 0.3219752754296894559, 0.3333333333333333703, 0.3219752754296894559, 0.3333333333333333703, 0.3219752754296894559, 0.3333333333333333703, 0.3219752754296894559, 0.3333333333333333703, 0.3219752754296894559, 0.3333333333333333703, 0.3219752754296894559, 0.3333333333333333703, 0.3219752754296894559, 0.3333333333333333703, 0.3219752754296894559, 0.3333333333333333703, 0.3219752754296894559, 0.3333333333333333703, 0.3219752754296894559, 0.3333333333333333703, 0.3219752754296894559, 0.3333333333333333703, 0.3219752754296894559, 0.3333333333333333703, 0.3219752754296894559, 0.3333333333333333703, 0.3219752754296894559, 0.3333333333333333703, 0.3219752754296894559, 0.3333333333333333703, 0.3219752754296894559, 0.3333333333333333703, 0.3219752754296894559, 0.3333333333333333703, 0.3219752754296894559, 0.3333333333333333703, 0.3219752754296894559, 0.3333333333333333703, 0.3219752754296894559, 0.3333333333333333703, 0.3219752754296894559, 0.3333333333333333703, 0.3219752754296894559, 0.3333333333333333703, 0.3219752754296894559, 0.3333333333333333703, 0.3219752754296894559, 0.3333333333333333703, 0.3219752754296894559, 0.3333333333333333703, 0.3219752754296894559, 0.3333333333333333703, 0.3219752754296894559, 0.3333333333333333703, 0.3219752754296894559, 0.3333333333333333703, 0.3219752754296894559, 0.3333333333333333703, 0.3219752754296894559, 0.3333333333333333703, 0.3219752754296894559, 0.3333333333333333703, 0.3219752754296894559, 0.3333333333333333703, 0.3219752754296894559, 0.3333333333333333703, 0.3219752754296894559, 0.3333333333333333703, 0.3219752754296894559, 0.3333333333333333703, 0.3219752754296894559, 0.3333333333333333703, 0.3219752754296894559, 0.3333333333333333703, 0.3219752754296894559, 0.3333333333333333703, 0.3219752754296894559, 0.3333333333333333703, 0.3219752754296894559, 0.3333333333333333703, 0.3219752754296894559, 0.3333333333333333703, 0.3219752754296894559, 0.3333333333333333703, 0.3219752754296894559, 0.3333333333333333703, 0.3219752754296894559, 0.3333333333333333703, 0.3219752754296894559, 0.3333333333333333703, 0.3219752754296894559, 0.3333333333333333703, 0.3219752754296894559, 0.3333333333333333703, 0.3219752754296894559, 0.3333333333333333703, 0.3219752754296894559, 0.3333333333333333703, 0.3219752754296894559, 0.3333333333333333703, 0.3219752754296894559, 0.3333333333333333703, 0.3219752754296894559, 0.3333333333333333703, 0.3219752754296894559, 0.3333333333333333703, 0.3219752754296894559, 0.3333333333333333703, 0.3219752754296894559, 0.3333333333333333703, 0.3219752754296894559, 0.3333333333333333703, 0.3219752754296894559, 0.3333333333333333703, 0.3219752754296894559, 0.3333333333333333703, 0.3219752754296894559, 0.3333333333333333703, 0.3219752754296894559, 0.3333333333333333703, 0.3219752754296894559, 0.3333333333333333703, 0.3219752754296894559, 0.3333333333333333703, 0.3219752754296894559, 0.3333333333333333703, 0.3219752754296894559, 0.3333333333333333703, 0.3219752754296894559, 0.3333333333333333703, 0.3219752754296894559, 0.3333333333333333703, 0.3219752754296894559, 0.3333333333333333703, 0.3219752754296894559, 0.3333333333333333703, 0.3219752754296894559, 0.3333333333333333703, 0.3219752754296894559, 0.3333333333333333703, 0.3219752754296894559, 0.3333333333333333703, 0.3219752754296894559, 0.3333333333333333703, 0.3219752754296894559, 0.3333333333333333703, 0.3219752754296894559, 0.3333333333333333703),
 ( 0.3333333333333333703, 0.3219752754296894559, 0.3333333333333333703, 0.3219752754296894559, 0.3333333333333333703, 0.3219752754296894559, 0.3333333333333333703, 0.3219752754296894559, 0.3333333333333333703, 0.3219752754296894559, 0.3333333333333333703, 0.3219752754296894559, 0.3333333333333333703, 0.3219752754296894559, 0.3333333333333333703, 0.3219752754296894559, 0.3333333333333333703, 0.3219752754296894559, 0.3333333333333333703, 0.3219752754296894559, 0.3333333333333333703, 0.3219752754296894559, 0.3333333333333333703, 0.3219752754296894559, 0.3333333333333333703, 0.3219752754296894559, 0.3333333333333333703, 0.3219752754296894559, 0.3333333333333333703, 0.3219752754296894559, 0.3333333333333333703, 0.3219752754296894559, 0.3333333333333333703, 0.3219752754296894559, 0.3333333333333333703, 0.3219752754296894559, 0.3333333333333333703, 0.3219752754296894559, 0.3333333333333333703, 0.3219752754296894559, 0.3333333333333333703, 0.3219752754296894559, 0.3333333333333333703, 0.3219752754296894559, 0.3333333333333333703, 0.3219752754296894559, 0.3333333333333333703, 0.3219752754296894559, 0.3333333333333333703, 0.3219752754296894559, 0.3333333333333333703, 0.3219752754296894559, 0.3333333333333333703, 0.3219752754296894559, 0.3333333333333333703, 0.3219752754296894559, 0.3333333333333333703, 0.3219752754296894559, 0.3333333333333333703, 0.3219752754296894559, 0.3333333333333333703, 0.3219752754296894559, 0.3333333333333333703, 0.3219752754296894559, 0.3333333333333333703, 0.3219752754296894559, 0.3333333333333333703, 0.3219752754296894559, 0.3333333333333333703, 0.3219752754296894559, 0.3333333333333333703, 0.3219752754296894559, 0.3333333333333333703, 0.3219752754296894559, 0.3333333333333333703, 0.3219752754296894559, 0.3333333333333333703, 0.3219752754296894559, 0.3333333333333333703, 0.3219752754296894559, 0.3333333333333333703, 0.3219752754296894559, 0.3333333333333333703, 0.3219752754296894559, 0.3333333333333333703, 0.3219752754296894559, 0.3333333333333333703, 0.3219752754296894559, 0.3333333333333333703, 0.3219752754296894559, 0.3333333333333333703, 0.3219752754296894559, 0.3333333333333333703, 0.3219752754296894559, 0.3333333333333333703, 0.3219752754296894559, 0.3333333333333333703, 0.3219752754296894559, 0.3333333333333333703, 0.3219752754296894559, 0.3333333333333333703, 0.3219752754296894559, 0.3333333333333333703, 0.3219752754296894559, 0.3333333333333333703, 0.3219752754296894559, 0.3333333333333333703, 0.3219752754296894559, 0.3333333333333333703, 0.3219752754296894559, 0.3333333333333333703, 0.3219752754296894559, 0.3333333333333333703, 0.3219752754296894559, 0.3333333333333333703, 0.3219752754296894559, 0.3333333333333333703, 0.3219752754296894559, 0.3333333333333333703, 0.3219752754296894559, 0.3333333333333333703, 0.3219752754296894559, 0.3333333333333333703, 0.3219752754296894559, 0.3333333333333333703, 0.3219752754296894559, 0.3333333333333333703, 0.3219752754296894559, 0.3333333333333333703, 0.3219752754296894559, 0.3333333333333333703, 0.3219752754296894559, 0.3333333333333333703, 0.3219752754296894559, 0.3333333333333333703, 0.3219752754296894559, 0.3333333333333333703, 0.3219752754296894559, 0.3333333333333333703, 0.3219752754296894559, 0.3333333333333333703, 0.3219752754296894559, 0.3333333333333333703, 0.3219752754296894559, 0.3333333333333333703, 0.3219752754296894559, 0.3333333333333333703, 0.3219752754296894559, 0.3333333333333333703, 0.3219752754296894559, 0.3333333333333333703, 0.3219752754296894559, 0.3333333333333333703, 0.3219752754296894559, 0.3333333333333333703, 0.3219752754296894559, 0.3333333333333333703, 0.3219752754296894559, 0.3333333333333333703, 0.3219752754296894559, 0.3333333333333333703, 0.3219752754296894559, 0.3333333333333333703, 0.3219752754296894559, 0.3333333333333333703, 0.3219752754296894559, 0.3333333333333333703, 0.3219752754296894559, 0.3333333333333333703, 0.3219752754296894559, 0.3333333333333333703, 0.3219752754296894559, 0.3333333333333333703, 0.3219752754296894559, 0.3333333333333333703, 0.3219752754296894559, 0.3333333333333333703, 0.3219752754296894559, 0.3333333333333333703, 0.3219752754296894559, 0.3333333333333333703, 0.3219752754296894559, 0.3333333333333333703, 0.3219752754296894559, 0.3333333333333333703, 0.3219752754296894559, 0.3333333333333333703, 0.3219752754296894559, 0.3333333333333333703, 0.3219752754296894559, 0.3333333333333333703, 0.3219752754296894559, 0.3333333333333333703),
 ( 1.000000000000000000, 0.9659258262890683122, 1.000000000000000000, 0.9659258262890683122, 1.000000000000000000, 0.9659258262890683122, 1.000000000000000000, 0.9659258262890683122, 1.000000000000000000, 0.9659258262890683122, 1.000000000000000000, 0.9659258262890683122, 1.000000000000000000, 0.9659258262890683122, 1.000000000000000000, 0.9659258262890683122, 1.000000000000000000, 0.9659258262890683122, 1.000000000000000000, 0.9659258262890683122, 1.000000000000000000, 0.9659258262890683122, 1.000000000000000000, 0.9659258262890683122, 1.000000000000000000, 0.9659258262890683122, 1.000000000000000000, 0.9659258262890683122, 1.000000000000000000, 0.9659258262890683122, 1.000000000000000000, 0.9659258262890683122, 1.000000000000000000, 0.9659258262890683122, 1.000000000000000000, 0.9659258262890683122, 1.000000000000000000, 0.9659258262890683122, 1.000000000000000000, 0.9659258262890683122, 1.000000000000000000, 0.9659258262890683122, 1.000000000000000000, 0.9659258262890683122, 1.000000000000000000, 0.9659258262890683122, 1.000000000000000000, 0.9659258262890683122, 1.000000000000000000, 0.9659258262890683122, 1.000000000000000000, 0.9659258262890683122, 1.000000000000000000, 0.9659258262890683122, 1.000000000000000000, 0.9659258262890683122, 1.000000000000000000, 0.9659258262890683122, 1.000000000000000000, 0.9659258262890683122, 1.000000000000000000, 0.9659258262890683122, 1.000000000000000000, 0.9659258262890683122, 1.000000000000000000, 0.9659258262890683122, 1.000000000000000000, 0.9659258262890683122, 1.000000000000000000, 0.9659258262890683122, 1.000000000000000000, 0.9659258262890683122, 1.000000000000000000, 0.9659258262890683122, 1.000000000000000000, 0.9659258262890683122, 1.000000000000000000, 0.9659258262890683122, 1.000000000000000000, 0.9659258262890683122, 1.000000000000000000, 0.9659258262890683122, 1.000000000000000000, 0.9659258262890683122, 1.000000000000000000, 0.9659258262890683122, 1.000000000000000000, 0.9659258262890683122, 1.000000000000000000, 0.9659258262890683122, 1.000000000000000000, 0.9659258262890683122, 1.000000000000000000, 0.9659258262890683122, 1.000000000000000000, 0.9659258262890683122, 1.000000000000000000, 0.9659258262890683122, 1.000000000000000000, 0.9659258262890683122, 1.000000000000000000, 0.9659258262890683122, 1.000000000000000000, 0.9659258262890683122, 1.000000000000000000, 0.9659258262890683122, 1.000000000000000000, 0.9659258262890683122, 1.000000000000000000, 0.9659258262890683122, 1.000000000000000000, 0.9659258262890683122, 1.000000000000000000, 0.9659258262890683122, 1.000000000000000000, 0.9659258262890683122, 1.000000000000000000, 0.9659258262890683122, 1.000000000000000000, 0.9659258262890683122, 1.000000000000000000, 0.9659258262890683122, 1.000000000000000000, 0.9659258262890683122, 1.000000000000000000, 0.9659258262890683122, 1.000000000000000000, 0.9659258262890683122, 1.000000000000000000, 0.9659258262890683122, 1.000000000000000000, 0.9659258262890683122, 1.000000000000000000, 0.9659258262890683122, 1.000000000000000000, 0.9659258262890683122, 1.000000000000000000, 0.9659258262890683122, 1.000000000000000000, 0.9659258262890683122, 1.000000000000000000, 0.9659258262890683122, 1.000000000000000000, 0.9659258262890683122, 1.000000000000000000, 0.9659258262890683122, 1.000000000000000000, 0.9659258262890683122, 1.000000000000000000, 0.9659258262890683122, 1.000000000000000000, 0.9659258262890683122, 1.000000000000000000, 0.9659258262890683122, 1.000000000000000000, 0.9659258262890683122, 1.000000000000000000, 0.9659258262890683122, 1.000000000000000000, 0.9659258262890683122, 1.000000000000000000, 0.9659258262890683122, 1.000000000000000000, 0.9659258262890683122, 1.000000000000000000, 0.9659258262890683122, 1.000000000000000000, 0.9659258262890683122, 1.000000000000000000, 0.9659258262890683122, 1.000000000000000000, 0.9659258262890683122, 1.000000000000000000, 0.9659258262890683122, 1.000000000000000000, 0.9659258262890683122, 1.000000000000000000, 0.9659258262890683122, 1.000000000000000000, 0.9659258262890683122, 1.000000000000000000, 0.9659258262890683122, 1.000000000000000000, 0.9659258262890683122, 1.000000000000000000, 0.9659258262890683122, 1.000000000000000000, 0.9659258262890683122, 1.000000000000000000, 0.9659258262890683122, 1.000000000000000000, 0.9659258262890683122, 1.000000000000000000),
 ( 0.3333333333333333703, 0.3219752754296894559, 0.3333333333333333703, 0.3219752754296894559, 0.3333333333333333703, 0.3219752754296894559, 0.3333333333333333703, 0.3219752754296894559, 0.3333333333333333703, 0.3219752754296894559, 0.3333333333333333703, 0.3219752754296894559, 0.3333333333333333703, 0.3219752754296894559, 0.3333333333333333703, 0.3219752754296894559, 0.3333333333333333703, 0.3219752754296894559, 0.3333333333333333703, 0.3219752754296894559, 0.3333333333333333703, 0.3219752754296894559, 0.3333333333333333703, 0.3219752754296894559, 0.3333333333333333703, 0.3219752754296894559, 0.3333333333333333703, 0.3219752754296894559, 0.3333333333333333703, 0.3219752754296894559, 0.3333333333333333703, 0.3219752754296894559, 0.3333333333333333703, 0.3219752754296894559, 0.3333333333333333703, 0.3219752754296894559, 0.3333333333333333703, 0.3219752754296894559, 0.3333333333333333703, 0.3219752754296894559, 0.3333333333333333703, 0.3219752754296894559, 0.3333333333333333703, 0.3219752754296894559, 0.3333333333333333703, 0.3219752754296894559, 0.3333333333333333703, 0.3219752754296894559, 0.3333333333333333703, 0.3219752754296894559, 0.3333333333333333703, 0.3219752754296894559, 0.3333333333333333703, 0.3219752754296894559, 0.3333333333333333703, 0.3219752754296894559, 0.3333333333333333703, 0.3219752754296894559, 0.3333333333333333703, 0.3219752754296894559, 0.3333333333333333703, 0.3219752754296894559, 0.3333333333333333703, 0.3219752754296894559, 0.3333333333333333703, 0.3219752754296894559, 0.3333333333333333703, 0.3219752754296894559, 0.3333333333333333703, 0.3219752754296894559, 0.3333333333333333703, 0.3219752754296894559, 0.3333333333333333703, 0.3219752754296894559, 0.3333333333333333703, 0.3219752754296894559, 0.3333333333333333703, 0.3219752754296894559, 0.3333333333333333703, 0.3219752754296894559, 0.3333333333333333703, 0.3219752754296894559, 0.3333333333333333703, 0.3219752754296894559, 0.3333333333333333703, 0.3219752754296894559, 0.3333333333333333703, 0.3219752754296894559, 0.3333333333333333703, 0.3219752754296894559, 0.3333333333333333703, 0.3219752754296894559, 0.3333333333333333703, 0.3219752754296894559, 0.3333333333333333703, 0.3219752754296894559, 0.3333333333333333703, 0.3219752754296894559, 0.3333333333333333703, 0.3219752754296894559, 0.3333333333333333703, 0.3219752754296894559, 0.3333333333333333703, 0.3219752754296894559, 0.3333333333333333703, 0.3219752754296894559, 0.3333333333333333703, 0.3219752754296894559, 0.3333333333333333703, 0.3219752754296894559, 0.3333333333333333703, 0.3219752754296894559, 0.3333333333333333703, 0.3219752754296894559, 0.3333333333333333703, 0.3219752754296894559, 0.3333333333333333703, 0.3219752754296894559, 0.3333333333333333703, 0.3219752754296894559, 0.3333333333333333703, 0.3219752754296894559, 0.3333333333333333703, 0.3219752754296894559, 0.3333333333333333703, 0.3219752754296894559, 0.3333333333333333703, 0.3219752754296894559, 0.3333333333333333703, 0.3219752754296894559, 0.3333333333333333703, 0.3219752754296894559, 0.3333333333333333703, 0.3219752754296894559, 0.3333333333333333703, 0.3219752754296894559, 0.3333333333333333703, 0.3219752754296894559, 0.3333333333333333703, 0.3219752754296894559, 0.3333333333333333703, 0.3219752754296894559, 0.3333333333333333703, 0.3219752754296894559, 0.3333333333333333703, 0.3219752754296894559, 0.3333333333333333703, 0.3219752754296894559, 0.3333333333333333703, 0.3219752754296894559, 0.3333333333333333703, 0.3219752754296894559, 0.3333333333333333703, 0.3219752754296894559, 0.3333333333333333703, 0.3219752754296894559, 0.3333333333333333703, 0.3219752754296894559, 0.3333333333333333703, 0.3219752754296894559, 0.3333333333333333703, 0.3219752754296894559, 0.3333333333333333703, 0.3219752754296894559, 0.3333333333333333703, 0.3219752754296894559, 0.3333333333333333703, 0.3219752754296894559, 0.3333333333333333703, 0.3219752754296894559, 0.3333333333333333703, 0.3219752754296894559, 0.3333333333333333703, 0.3219752754296894559, 0.3333333333333333703, 0.3219752754296894559, 0.3333333333333333703, 0.3219752754296894559, 0.3333333333333333703, 0.3219752754296894559, 0.3333333333333333703, 0.3219752754296894559, 0.3333333333333333703, 0.3219752754296894559, 0.3333333333333333703, 0.3219752754296894559, 0.3333333333333333703, 0.3219752754296894559, 0.3333333333333333703, 0.3219752754296894559, 0.3333333333333333703, 0.3219752754296894559, 0.3333333333333333703),
 ( 0.3333333333333333703, 0.3219752754296894559, 0.3333333333333333703, 0.3219752754296894559, 0.3333333333333333703, 0.3219752754296894559, 0.3333333333333333703, 0.3219752754296894559, 0.3333333333333333703, 0.3219752754296894559, 0.3333333333333333703, 0.3219752754296894559, 0.3333333333333333703, 0.3219752754296894559, 0.3333333333333333703, 0.3219752754296894559, 0.3333333333333333703, 0.3219752754296894559, 0.3333333333333333703, 0.3219752754296894559, 0.3333333333333333703, 0.3219752754296894559, 0.3333333333333333703, 0.3219752754296894559, 0.3333333333333333703, 0.3219752754296894559, 0.3333333333333333703, 0.3219752754296894559, 0.3333333333333333703, 0.3219752754296894559, 0.3333333333333333703, 0.3219752754296894559, 0.3333333333333333703, 0.3219752754296894559, 0.3333333333333333703, 0.3219752754296894559, 0.3333333333333333703, 0.3219752754296894559, 0.3333333333333333703, 0.3219752754296894559, 0.3333333333333333703, 0.3219752754296894559, 0.3333333333333333703, 0.3219752754296894559, 0.3333333333333333703, 0.3219752754296894559, 0.3333333333333333703, 0.3219752754296894559, 0.3333333333333333703, 0.3219752754296894559, 0.3333333333333333703, 0.3219752754296894559, 0.3333333333333333703, 0.3219752754296894559, 0.3333333333333333703, 0.3219752754296894559, 0.3333333333333333703, 0.3219752754296894559, 0.3333333333333333703, 0.3219752754296894559, 0.3333333333333333703, 0.3219752754296894559, 0.3333333333333333703, 0.3219752754296894559, 0.3333333333333333703, 0.3219752754296894559, 0.3333333333333333703, 0.3219752754296894559, 0.3333333333333333703, 0.3219752754296894559, 0.3333333333333333703, 0.3219752754296894559, 0.3333333333333333703, 0.3219752754296894559, 0.3333333333333333703, 0.3219752754296894559, 0.3333333333333333703, 0.3219752754296894559, 0.3333333333333333703, 0.3219752754296894559, 0.3333333333333333703, 0.3219752754296894559, 0.3333333333333333703, 0.3219752754296894559, 0.3333333333333333703, 0.3219752754296894559, 0.3333333333333333703, 0.3219752754296894559, 0.3333333333333333703, 0.3219752754296894559, 0.3333333333333333703, 0.3219752754296894559, 0.3333333333333333703, 0.3219752754296894559, 0.3333333333333333703, 0.3219752754296894559, 0.3333333333333333703, 0.3219752754296894559, 0.3333333333333333703, 0.3219752754296894559, 0.3333333333333333703, 0.3219752754296894559, 0.3333333333333333703, 0.3219752754296894559, 0.3333333333333333703, 0.3219752754296894559, 0.3333333333333333703, 0.3219752754296894559, 0.3333333333333333703, 0.3219752754296894559, 0.3333333333333333703, 0.3219752754296894559, 0.3333333333333333703, 0.3219752754296894559, 0.3333333333333333703, 0.3219752754296894559, 0.3333333333333333703, 0.3219752754296894559, 0.3333333333333333703, 0.3219752754296894559, 0.3333333333333333703, 0.3219752754296894559, 0.3333333333333333703, 0.3219752754296894559, 0.3333333333333333703, 0.3219752754296894559, 0.3333333333333333703, 0.3219752754296894559, 0.3333333333333333703, 0.3219752754296894559, 0.3333333333333333703, 0.3219752754296894559, 0.3333333333333333703, 0.3219752754296894559, 0.3333333333333333703, 0.3219752754296894559, 0.3333333333333333703, 0.3219752754296894559, 0.3333333333333333703, 0.3219752754296894559, 0.3333333333333333703, 0.3219752754296894559, 0.3333333333333333703, 0.3219752754296894559, 0.3333333333333333703, 0.3219752754296894559, 0.3333333333333333703, 0.3219752754296894559, 0.3333333333333333703, 0.3219752754296894559, 0.3333333333333333703, 0.3219752754296894559, 0.3333333333333333703, 0.3219752754296894559, 0.3333333333333333703, 0.3219752754296894559, 0.3333333333333333703, 0.3219752754296894559, 0.3333333333333333703, 0.3219752754296894559, 0.3333333333333333703, 0.3219752754296894559, 0.3333333333333333703, 0.3219752754296894559, 0.3333333333333333703, 0.3219752754296894559, 0.3333333333333333703, 0.3219752754296894559, 0.3333333333333333703, 0.3219752754296894559, 0.3333333333333333703, 0.3219752754296894559, 0.3333333333333333703, 0.3219752754296894559, 0.3333333333333333703, 0.3219752754296894559, 0.3333333333333333703, 0.3219752754296894559, 0.3333333333333333703, 0.3219752754296894559, 0.3333333333333333703, 0.3219752754296894559, 0.3333333333333333703, 0.3219752754296894559, 0.3333333333333333703, 0.3219752754296894559, 0.3333333333333333703, 0.3219752754296894559, 0.3333333333333333703, 0.3219752754296894559, 0.3333333333333333703, 0.3219752754296894559, 0.3333333333333333703),
 ( 1.000000000000000000, 0.9659258262890683122, 1.000000000000000000, 0.9659258262890683122, 1.000000000000000000, 0.9659258262890683122, 1.000000000000000000, 0.9659258262890683122, 1.000000000000000000, 0.9659258262890683122, 1.000000000000000000, 0.9659258262890683122, 1.000000000000000000, 0.9659258262890683122, 1.000000000000000000, 0.9659258262890683122, 1.000000000000000000, 0.9659258262890683122, 1.000000000000000000, 0.9659258262890683122, 1.000000000000000000, 0.9659258262890683122, 1.000000000000000000, 0.9659258262890683122, 1.000000000000000000, 0.9659258262890683122, 1.000000000000000000, 0.9659258262890683122, 1.000000000000000000, 0.9659258262890683122, 1.000000000000000000, 0.9659258262890683122, 1.000000000000000000, 0.9659258262890683122, 1.000000000000000000, 0.9659258262890683122, 1.000000000000000000, 0.9659258262890683122, 1.000000000000000000, 0.9659258262890683122, 1.000000000000000000, 0.9659258262890683122, 1.000000000000000000, 0.9659258262890683122, 1.000000000000000000, 0.9659258262890683122, 1.000000000000000000, 0.9659258262890683122, 1.000000000000000000, 0.9659258262890683122, 1.000000000000000000, 0.9659258262890683122, 1.000000000000000000, 0.9659258262890683122, 1.000000000000000000, 0.9659258262890683122, 1.000000000000000000, 0.9659258262890683122, 1.000000000000000000, 0.9659258262890683122, 1.000000000000000000, 0.9659258262890683122, 1.000000000000000000, 0.9659258262890683122, 1.000000000000000000, 0.9659258262890683122, 1.000000000000000000, 0.9659258262890683122, 1.000000000000000000, 0.9659258262890683122, 1.000000000000000000, 0.9659258262890683122, 1.000000000000000000, 0.9659258262890683122, 1.000000000000000000, 0.9659258262890683122, 1.000000000000000000, 0.9659258262890683122, 1.000000000000000000, 0.9659258262890683122, 1.000000000000000000, 0.9659258262890683122, 1.000000000000000000, 0.9659258262890683122, 1.000000000000000000, 0.9659258262890683122, 1.000000000000000000, 0.9659258262890683122, 1.000000000000000000, 0.9659258262890683122, 1.000000000000000000, 0.9659258262890683122, 1.000000000000000000, 0.9659258262890683122, 1.000000000000000000, 0.9659258262890683122, 1.000000000000000000, 0.9659258262890683122, 1.000000000000000000, 0.9659258262890683122, 1.000000000000000000, 0.9659258262890683122, 1.000000000000000000, 0.9659258262890683122, 1.000000000000000000, 0.9659258262890683122, 1.000000000000000000, 0.9659258262890683122, 1.000000000000000000, 0.9659258262890683122, 1.000000000000000000, 0.9659258262890683122, 1.000000000000000000, 0.9659258262890683122, 1.000000000000000000, 0.9659258262890683122, 1.000000000000000000, 0.9659258262890683122, 1.000000000000000000, 0.9659258262890683122, 1.000000000000000000, 0.9659258262890683122, 1.000000000000000000, 0.9659258262890683122, 1.000000000000000000, 0.9659258262890683122, 1.000000000000000000, 0.9659258262890683122, 1.000000000000000000, 0.9659258262890683122, 1.000000000000000000, 0.9659258262890683122, 1.000000000000000000, 0.9659258262890683122, 1.000000000000000000, 0.9659258262890683122, 1.000000000000000000, 0.9659258262890683122, 1.000000000000000000, 0.9659258262890683122, 1.000000000000000000, 0.9659258262890683122, 1.000000000000000000, 0.9659258262890683122, 1.000000000000000000, 0.9659258262890683122, 1.000000000000000000, 0.9659258262890683122, 1.000000000000000000, 0.9659258262890683122, 1.000000000000000000, 0.9659258262890683122, 1.000000000000000000, 0.9659258262890683122, 1.000000000000000000, 0.9659258262890683122, 1.000000000000000000, 0.9659258262890683122, 1.000000000000000000, 0.9659258262890683122, 1.000000000000000000, 0.9659258262890683122, 1.000000000000000000, 0.9659258262890683122, 1.000000000000000000, 0.9659258262890683122, 1.000000000000000000, 0.9659258262890683122, 1.000000000000000000, 0.9659258262890683122, 1.000000000000000000, 0.9659258262890683122, 1.000000000000000000, 0.9659258262890683122, 1.000000000000000000, 0.9659258262890683122, 1.000000000000000000, 0.9659258262890683122, 1.000000000000000000, 0.9659258262890683122, 1.000000000000000000, 0.9659258262890683122, 1.000000000000000000, 0.9659258262890683122, 1.000000000000000000, 0.9659258262890683122, 1.000000000000000000, 0.9659258262890683122, 1.000000000000000000, 0.9659258262890683122, 1.000000000000000000, 0.9659258262890683122, 1.000000000000000000) ) ) 
 REPRESENTATION_ITEM ( '' )  SURFACE ( )  );
#536=CARTESIAN_POINT ( 'NONE',  ( -19.99999999999999645, -23.83517299489738051, 18.70117750791695954 ) ) ;
#538=CARTESIAN_POINT ( 'NONE',  ( -13.82508104294702100, -18.95583473709188382, 22.20507249208304401 ) ) ;
#540=CARTESIAN_POINT ( 'NONE',  ( -14.83517299489739649, -18.99999999999997868, 20.01367750791695954 ) ) ;
#542=CARTESIAN_POINT ( 'NONE',  ( -16.50457296725820555, -28.95583473709189803, 17.60742750791695599 ) ) ;
#544=CARTESIAN_POINT ( 'NONE',  ( -13.82508104294702100, -18.95583473709188382, 27.45507249208304046 ) ) ;
#554=CARTESIAN_POINT ( 'NONE',  ( -18.64274437364860049, -18.02023567606023491, 26.79882249208304401 ) ) ;
#555=CARTESIAN_POINT ( 'NONE',  ( -19.41254052147350961, -21.64274437364857562, 15.86132249208304223 ) ) ;
#557=CARTESIAN_POINT ( 'NONE',  ( -18.04416526290808420, -24.63902057219074493, 28.98242750791696309 ) ) ;
#559=CARTESIAN_POINT ( 'NONE',  ( -21.99999999999999289, -24.16482700510262305, 20.67382249208304046 ) ) ;
#575=CARTESIAN_POINT ( 'NONE',  ( -8.855408670957631401, -20.64274437364852943, 31.38867750791695599 ) ) ;
#579=CARTESIAN_POINT ( 'NONE',  ( -15.16482700510262482, -20.99999999999997513, 37.73632249208304756 ) ) ;
#580=CARTESIAN_POINT ( 'NONE',  ( -9.754982604823348780, -18.99630608921234654, 20.66992750791695954 ) ) ;
#586=CARTESIAN_POINT ( 'NONE',  ( -14.36097942780923731, -27.04416526290806999, 27.66992750791696665 ) ) ;
#603=CARTESIAN_POINT ( 'NONE',  ( -19.99999999999999645, -23.83517299489738051, 23.95117750791695954 ) ) ;
#606=CARTESIAN_POINT ( 'NONE',  ( -15.16482700510263371, -18.99999999999997868, 37.73632249208303335 ) ) ;
#608=CARTESIAN_POINT ( 'NONE',  ( -12.48433729119799196, -22.35725562635139596, 33.36132249208304756 ) ) ;
#629=CARTESIAN_POINT ( 'NONE',  ( -14.83517299489739649, -18.99999999999997868, 35.76367750791695954 ) ) ;
#633=CARTESIAN_POINT ( 'NONE',  ( -9.955834737091903364, -25.17491895705294880, 23.51757249208304401 ) ) ;
#636=CARTESIAN_POINT ( 'NONE',  ( -12.35725562635143682, -19.75228648362908501, 15.20117750791695777 ) ) ;
#638=CARTESIAN_POINT ( 'NONE',  ( -19.41254052147348830, -26.35725562635142083, 34.01367750791696665 ) ) ;
#640=CARTESIAN_POINT ( 'NONE',  ( -10.75228648362912232, -21.35725562635138530, 22.86132249208304401 ) ) ;
#651=CARTESIAN_POINT ( 'NONE',  ( -15.16482700510264436, -16.99999999999997868, 37.73632249208302625 ) ) ;
#657=CARTESIAN_POINT ( 'NONE',  ( -17.68048971390461688, -25.35725562635141372, 34.01367750791696665 ) ) ;
#660=CARTESIAN_POINT ( 'NONE',  ( -18.64274437364860049, -18.02023567606023491, 21.54882249208304046 ) ) ;
#679=CARTESIAN_POINT ( 'NONE',  ( -18.35725562635144925, -17.85540867095761186, 24.82617750791695599 ) ) ;
#684=CARTESIAN_POINT ( 'NONE',  ( -17.99999999999999645, -24.16482700510260173, 31.17382249208304046 ) ) ;
#685=CARTESIAN_POINT ( 'NONE',  ( -18.35725562635144925, -17.85540867095761186, 19.57617750791695954 ) ) ;
#690=CARTESIAN_POINT ( 'NONE',  ( -16.64274437364856496, -26.51566270880199738, 28.32617750791696665 ) ) ;
#708=CARTESIAN_POINT ( 'NONE',  ( -20.04416526290808065, -25.17491895705300209, 34.23242750791695954 ) ) ;
#711=CARTESIAN_POINT ( 'NONE',  ( -14.83517299489735741, -28.99999999999998224, 29.86132249208304401 ) ) ;
#713=CARTESIAN_POINT ( 'NONE',  ( -17.31681416490117087, -21.92450931948788551, 26.58007249208304756 ) ) ;
#727=CARTESIAN_POINT ( 'NONE',  ( -18.53959229564986799, -20.21908421996107563, 29.85742750791695599 ) ) ;
#729=CARTESIAN_POINT ( 'NONE',  ( -17.64274437364858983, -19.75228648362910633, 26.79882249208304401 ) ) ;
#731=CARTESIAN_POINT ( 'NONE',  ( -10.04416526290807710, -25.50457296725819489, 26.79492750791695954 ) ) ;
#734=CARTESIAN_POINT ( 'NONE',  ( -17.35725562635144215, -19.58745947852648683, 35.32617750791695954 ) ) ;
#736=CARTESIAN_POINT ( 'NONE',  ( -12.35725562635140307, -28.24771351637085459, 24.17382249208304046 ) ) ;
#746=CARTESIAN_POINT ( 'NONE',  ( -16.35725562635142794, -21.31951028609535470, 30.07617750791696309 ) ) ;
#748=CARTESIAN_POINT ( 'NONE',  ( -9.996306089212408708, -18.75498260482328661, 38.39257249208304756 ) ) ;
#764=CARTESIAN_POINT ( 'NONE',  ( -20.00369391078762860, -18.75498260482333279, 24.60742750791696309 ) ) ;
#768=CARTESIAN_POINT ( 'NONE',  ( -12.48433729119799196, -22.35725562635139596, 28.11132249208304401 ) ) ;
#769=CARTESIAN_POINT ( 'NONE',  ( -9.020235676060220698, -27.64274437364852588, 16.51367750791695954 ) ) ;
#775=CARTESIAN_POINT ( 'NONE',  ( -13.64274437364856141, -26.68048971390460622, 32.70117750791696665 ) ) ;
#794=CARTESIAN_POINT ( 'NONE',  ( -16.17491895705301275, -18.95583473709189803, 30.29492750791695244 ) ) ;
#797=CARTESIAN_POINT ( 'NONE',  ( -19.24771351637086880, -26.64274437364857206, 25.48632249208304401 ) ) ;
#799=CARTESIAN_POINT ( 'NONE',  ( -17.95583473709190869, -24.96867458239598037, 36.20507249208304756 ) ) ;
#817=CARTESIAN_POINT ( 'NONE',  ( -18.53959229564986799, -20.21908421996107563, 35.10742750791694533 ) ) ;
#819=CARTESIAN_POINT ( 'NONE',  ( -16.17491895705296656, -29.04416526290807710, 30.08007249208304401 ) ) ;
#822=CARTESIAN_POINT ( 'NONE',  ( -16.17491895705301275, -18.95583473709189803, 35.54492750791695954 ) ) ;
#825=CARTESIAN_POINT ( 'NONE',  ( -20.04416526290808065, -25.17491895705300209, 34.23242750791696665 ) ) ;
#827=CARTESIAN_POINT ( 'NONE',  ( -20.04416526290809131, -22.82508104294700502, 31.39257249208304046 ) ) ;
#838=CARTESIAN_POINT ( 'NONE',  ( -11.95583473709191047, -23.36097942780921954, 36.85742750791697375 ) ) ;
#840=CARTESIAN_POINT ( 'NONE',  ( -18.64274437364860049, -18.02023567606023491, 26.79882249208304401 ) ) ;
#855=CARTESIAN_POINT ( 'NONE',  ( -16.71081734191520596, -31.04416526290808065, 3.830072492083039126 ) ) ;
#859=CARTESIAN_POINT ( 'NONE',  ( -12.92450931948790149, -21.68318583509881137, 27.89257249208304401 ) ) ;
#860=CARTESIAN_POINT ( 'NONE',  ( -8.855408670957631401, -20.64274437364852943, 26.13867750791696309 ) ) ;
#882=CARTESIAN_POINT ( 'NONE',  ( -17.64274437364855430, -28.24771351637087236, 33.57617750791696665 ) ) ;
#886=CARTESIAN_POINT ( 'NONE',  ( -20.04416526290809131, -22.82508104294699791, 26.14257249208303691 ) ) ;
#891=CARTESIAN_POINT ( 'NONE',  ( -17.51566270880199738, -25.64274437364856496, 35.98632249208304756 ) ) ;
#900=CARTESIAN_POINT ( 'NONE',  ( -16.17491895705301275, -18.95583473709189803, 30.29492750791695244 ) ) ;
#910=CARTESIAN_POINT ( 'NONE',  ( -20.04416526290808065, -25.17491895705300209, 28.98242750791695244 ) ) ;
#912=CARTESIAN_POINT ( 'NONE',  ( -10.58745947852648328, -26.35725562635138530, 28.98632249208304401 ) ) ;
#915=CARTESIAN_POINT ( 'NONE',  ( -13.49542703274178379, -19.04416526290806289, 30.73242750791695599 ) ) ;
#918=CARTESIAN_POINT ( 'NONE',  ( -10.58745947852649927, -21.64274437364853654, 26.13867750791695599 ) ) ;
#933=CARTESIAN_POINT ( 'NONE',  ( -17.35725562635144215, -19.58745947852648683, 3.826177507916958209 ) ) ;
#935=CARTESIAN_POINT ( 'NONE',  ( -9.754982604823302594, -29.00369391078756465, 34.45507249208304046 ) ) ;
#951=CARTESIAN_POINT ( 'NONE',  ( -12.95952864787948755, -30.95583473709188382, 8.642572492083038682 ) ) ;
#953=ORIENTED_EDGE ( 'NONE', *, *, #2641, .T. ) ;
#956=CARTESIAN_POINT ( 'NONE',  ( -13.64274437364856141, -26.68048971390460622, 6.451177507916961318 ) ) ;
#959=CARTESIAN_POINT ( 'NONE',  ( -7.999999999999996447, -24.16482700510256976, 31.82617750791695954 ) ) ;
#975=EDGE_CURVE ( 'NONE', #12569, #15887, #9043, .T. ) ;
#983=CARTESIAN_POINT ( 'NONE',  ( -17.04047135212043784, -30.95583473709190159, 7.107427507916957765 ) ) ;
#987=CARTESIAN_POINT ( 'NONE',  ( -14.03132541760400009, -26.95583473709189448, 8.642572492083042235 ) ) ;
#991=CARTESIAN_POINT ( 'NONE',  ( -18.04416526290808775, -23.36097942780924441, 36.64257249208304756 ) ) ;
#1002=CARTESIAN_POINT ( 'NONE',  ( -9.999999999999994671, -24.16482700510257686, 21.32617750791695599 ) ) ;
#1007=CARTESIAN_POINT ( 'NONE',  ( -12.35725562635143682, -19.75228648362908501, -0.5488224920830419018 ) ) ;
#1010=CARTESIAN_POINT ( 'NONE',  ( -21.14459132904239169, -20.64274437364858628, 31.61132249208303691 ) ) ;
#1011=CARTESIAN_POINT ( 'NONE',  ( -12.64274437364855252, -28.41254052147347053, 37.95117750791695954 ) ) ;
#1013=CARTESIAN_POINT ( 'NONE',  ( -9.955834737091903364, -25.17491895705294880, 39.26757249208304046 ) ) ;
#1018=CARTESIAN_POINT ( 'NONE',  ( -13.49542703274178379, -19.04416526290806289, 35.98242750791696665 ) ) ;
#1022=CARTESIAN_POINT ( 'NONE',  ( -13.49542703274174116, -28.95583473709188738, 34.89257249208303335 ) ) ;
#1033=CARTESIAN_POINT ( 'NONE',  ( -14.83517299489739649, -18.99999999999997868, 4.263677507916958653 ) ) ;
#1035=CARTESIAN_POINT ( 'NONE',  ( -17.04047135212050890, -17.04416526290807710, 37.51757249208304046 ) ) ;
#1047=CARTESIAN_POINT ( 'NONE',  ( -11.64274437364859693, -17.85540867095757989, 6.673822492083038682 ) ) ;
#1052=CARTESIAN_POINT ( 'NONE',  ( -14.03132541760400009, -26.95583473709189448, 40.14257249208306177 ) ) ;
#1053=CARTESIAN_POINT ( 'NONE',  ( -18.35725562635144925, -17.85540867095761186, 24.82617750791695599 ) ) ;
#1074=CARTESIAN_POINT ( 'NONE',  ( -16.50457296725820555, -28.95583473709189448, 38.60742750791694533 ) ) ;
#1078=CARTESIAN_POINT ( 'NONE',  ( -14.83517299489736985, -26.99999999999998579, 3.611322492083043123 ) ) ;
#1081=CARTESIAN_POINT ( 'NONE',  ( -15.63902057219076269, -20.95583473709189448, 9.294927507916961318 ) ) ;
#1093=CARTESIAN_POINT ( 'NONE',  ( -9.999999999999994671, -24.16482700510257686, 26.57617750791695954 ) ) ;
#1095=CARTESIAN_POINT ( 'NONE',  ( -18.78091578003889950, -27.53959229564985378, 7.544927507916956877 ) ) ;
#1098=CARTESIAN_POINT ( 'NONE',  ( -14.83517299489735741, -28.99999999999998224, 8.861322492083040459 ) ) ;
#1100=CARTESIAN_POINT ( 'NONE',  ( -11.35725562635144925, -18.02023567606020293, -0.5488224920830435671 ) ) ;
#1103=CARTESIAN_POINT ( 'NONE',  ( -19.95583473709190514, -25.50457296725822687, 36.20507249208303335 ) ) ;
#1108=CARTESIAN_POINT ( 'NONE',  ( -11.21908421996108629, -20.46040770435011069, 31.16992750791695599 ) ) ;
#1114=CARTESIAN_POINT ( 'NONE',  ( -19.95583473709190514, -25.50457296725823042, 41.45507249208304046 ) ) ;
#1124=CARTESIAN_POINT ( 'NONE',  ( -12.35725562635143682, -19.75228648362908501, 4.701177507916957765 ) ) ;
#1125=CARTESIAN_POINT ( 'NONE',  ( -10.58745947852649927, -21.64274437364853654, 5.138677507916957765 ) ) ;
#1127=CARTESIAN_POINT ( 'NONE',  ( -20.97976432393974022, -27.64274437364858628, 35.98632249208303335 ) ) ;
#1132=CARTESIAN_POINT ( 'NONE',  ( -17.95583473709191580, -23.03132541760400898, 34.66992750791696665 ) ) ;
#1133=CARTESIAN_POINT ( 'NONE',  ( -19.41254052147348830, -26.35725562635142083, 7.763677507916958653 ) ) ;
#1142=CIRCLE ( 'NONE', #15856, 0.9999999999999974465 ) ;
#1146=CARTESIAN_POINT ( 'NONE',  ( -18.35725562635144925, -17.85540867095761186, 40.57617750791695244 ) ) ;
#1147=ORIENTED_EDGE ( 'NONE', *, *, #4748, .T. ) ;
#1151=CARTESIAN_POINT ( 'NONE',  ( -12.04416526290808420, -23.03132541760398766, 38.83007249208304756 ) ) ;
#1152=CARTESIAN_POINT ( 'NONE',  ( -7.955834737091916686, -22.28918265808470522, 36.85742750791695244 ) ) ;
#1158=VERTEX_POINT ( 'NONE', #1514 ) ;
#1171=CARTESIAN_POINT ( 'NONE',  ( -18.35725562635144925, -17.85540867095761186, 3.826177507916956433 ) ) ;
#1174=CARTESIAN_POINT ( 'NONE',  ( -12.31951028609536536, -25.35725562635139596, 7.986322492083044011 ) ) ;
#1177=CARTESIAN_POINT ( 'NONE',  ( -12.48433729119798130, -25.64274437364855075, 0.7636775079169598746 ) ) ;
#1187=CARTESIAN_POINT ( 'NONE',  ( -11.46040770435012668, -27.78091578003887463, 32.48242750791695954 ) ) ;
#1192=CARTESIAN_POINT ( 'NONE',  ( -16.71081734191520596, -31.04416526290808065, 40.58007249208304756 ) ) ;
#1193=CARTESIAN_POINT ( 'NONE',  ( -20.97976432393977575, -20.35725562635143504, 3.388677507916956877 ) ) ;
#1197=CARTESIAN_POINT ( 'NONE',  ( -11.99999999999999289, -23.83517299489735564, 2.298822492083042235 ) ) ;
#1205=CARTESIAN_POINT ( 'NONE',  ( -19.95583473709191225, -22.49542703274176603, 39.91992750791695954 ) ) ;
#1207=CARTESIAN_POINT ( 'NONE',  ( -13.82508104294702100, -18.95583473709188382, 32.70507249208304046 ) ) ;
#1219=CARTESIAN_POINT ( 'NONE',  ( -11.46040770435012668, -27.78091578003887463, 0.9824275079169582092 ) ) ;
#1220=CARTESIAN_POINT ( 'NONE',  ( -9.955834737091912245, -22.82508104294696594, 0.1074275079169582509 ) ) ;
#1222=CARTESIAN_POINT ( 'NONE',  ( -17.64274437364858983, -19.75228648362910633, 11.04882249208304046 ) ) ;
#1226=CARTESIAN_POINT ( 'NONE',  ( -15.96867458239597326, -26.95583473709190159, 28.10742750791695954 ) ) ;
#1227=CARTESIAN_POINT ( 'NONE',  ( -19.24771351637089367, -21.35725562635142438, 3.388677507916958653 ) ) ;
#1243=CARTESIAN_POINT ( 'NONE',  ( -9.020235676060250896, -20.35725562635137820, 7.111322492083040459 ) ) ;
#1245=( NAMED_UNIT ( * ) SI_UNIT ( $, .STERADIAN. ) SOLID_ANGLE_UNIT ( ) );
#1249=CARTESIAN_POINT ( 'NONE',  ( -17.07549068051210739, -21.68318583509881847, 3.607427507916959097 ) ) ;
#1251=CARTESIAN_POINT ( 'NONE',  ( -18.64274437364860049, -18.02023567606023491, 11.04882249208303868 ) ) ;
#1275=CARTESIAN_POINT ( 'NONE',  ( -12.64274437364855252, -28.41254052147347053, 37.95117750791695954 ) ) ;
#1280=CARTESIAN_POINT ( 'NONE',  ( -13.64274437364857739, -21.31951028609534760, 1.423822492083042901 ) ) ;
#1284=CARTESIAN_POINT ( 'NONE',  ( -14.83517299489736985, -26.99999999999998579, 40.36132249208304756 ) ) ;
#1299=CARTESIAN_POINT ( 'NONE',  ( -11.46040770435012668, -27.78091578003887463, 27.23242750791694888 ) ) ;
#1301=CARTESIAN_POINT ( 'NONE',  ( -19.95583473709191580, -22.49542703274176603, 3.169927507916957321 ) ) ;
#1305=CARTESIAN_POINT ( 'NONE',  ( -22.04416526290809486, -22.28918265808477628, 41.89257249208304046 ) ) ;
#1307=CARTESIAN_POINT ( 'NONE',  ( -14.83517299489740715, -16.99999999999997868, -0.9863224920830435671 ) ) ;
#1309=CARTESIAN_POINT ( 'NONE',  ( -16.35725562635141372, -26.68048971390461332, 4.048822492083043123 ) ) ;
#1315=CARTESIAN_POINT ( 'NONE',  ( -17.64274437364855430, -28.24771351637087236, 38.82617750791695954 ) ) ;
#1319=CARTESIAN_POINT ( 'NONE',  ( -16.17491895705296656, -29.04416526290807354, 40.58007249208304046 ) ) ;
#1328=CARTESIAN_POINT ( 'NONE',  ( -10.04416526290807710, -25.50457296725819489, 0.5449275079169579872 ) ) ;
#1329=CARTESIAN_POINT ( 'NONE',  ( -12.64274437364855252, -28.41254052147347053, 16.95117750791695954 ) ) ;
#1331=CARTESIAN_POINT ( 'NONE',  ( -14.83517299489735741, -28.99999999999998224, 3.611322492083041347 ) ) ;
#1333=CARTESIAN_POINT ( 'NONE',  ( -11.46040770435012668, -27.78091578003887463, 0.9824275079169582092 ) ) ;
#1334=CARTESIAN_POINT ( 'NONE',  ( -19.99999999999999645, -23.83517299489738051, 2.951177507916958209 ) ) ;
#1346=CARTESIAN_POINT ( 'NONE',  ( -15.16482700510264436, -16.99999999999997868, 11.48632249208304046 ) ) ;
#1351=CARTESIAN_POINT ( 'NONE',  ( -14.03132541760401786, -21.04416526290806289, 4.482427507916961318 ) ) ;
#1353=CARTESIAN_POINT ( 'NONE',  ( -9.020235676060250896, -20.35725562635137820, 7.111322492083040459 ) ) ;
#1364=CARTESIAN_POINT ( 'NONE',  ( -10.52874183968111765, -22.23000804518926543, 4.401948939463559618E-14 ) ) ;
#1373=CARTESIAN_POINT ( 'NONE',  ( -17.64274437364855430, -28.24771351637087236, 38.82617750791695954 ) ) ;
#1377=CARTESIAN_POINT ( 'NONE',  ( -13.64274437364857739, -21.31951028609534760, 6.673822492083044011 ) ) ;
#1381=CARTESIAN_POINT ( 'NONE',  ( -16.35725562635141372, -26.68048971390461332, 40.79882249208304756 ) ) ;
#1393=AXIS2_PLACEMENT_3D ( 'NONE', #337, #13652, #7987 ) ;
#1394=CARTESIAN_POINT ( 'NONE',  ( -9.955834737091912245, -22.82508104294696594, 0.1074275079169582509 ) ) ;
#1397=PRODUCT_DEFINITION_CONTEXT ( 'detailed design', #10429, 'design' ) ;
#1398=CARTESIAN_POINT ( 'NONE',  ( -20.00369391078757886, -29.24501739517668142, 41.01757249208304046 ) ) ;
#1399=CARTESIAN_POINT ( 'NONE',  ( -19.41254052147348830, -26.35725562635142083, 39.26367750791695954 ) ) ;
#1402=CARTESIAN_POINT ( 'NONE',  ( -15.16482700510262482, -20.99999999999997513, 0.9863224920830429010 ) ) ;
#1416=SURFACE_SIDE_STYLE ('',( #7294 ) ) ;
#1422=CARTESIAN_POINT ( 'NONE',  ( -12.64274437364855252, -28.41254052147347053, 6.451177507916959541 ) ) ;
#1424=CARTESIAN_POINT ( 'NONE',  ( -18.53959229564986799, -20.21908421996107563, 19.35742750791695599 ) ) ;
#1426=CARTESIAN_POINT ( 'NONE',  ( -12.35725562635140307, -28.24771351637085459, 3.173822492083041347 ) ) ;
#1428=CARTESIAN_POINT ( 'NONE',  ( -15.63902057219076269, -20.95583473709189448, 40.79492750791695244 ) ) ;
#1431=CARTESIAN_POINT ( 'NONE',  ( -15.16482700510259640, -28.99999999999998224, 6.888677507916957765 ) ) ;
#1442=CARTESIAN_POINT ( 'NONE',  ( -13.28918265808478694, -16.95583473709189093, 16.95507249208304046 ) ) ;
#1444=SURFACE_STYLE_USAGE ( .BOTH. , #14872 ) ;
#1448=ORIENTED_EDGE ( 'NONE', *, *, #11863, .T. ) ;
#1450=CARTESIAN_POINT ( 'NONE',  ( -15.96867458239597326, -26.95583473709190159, 12.35742750791696132 ) ) ;
#1452=CARTESIAN_POINT ( 'NONE',  ( -9.020235676060250896, -20.35725562635137820, 1.861322492083039126 ) ) ;
#1474=CARTESIAN_POINT ( 'NONE',  ( -11.64274437364854187, -30.14459132904234195, 22.20117750791695599 ) ) ;
#1478=CARTESIAN_POINT ( 'NONE',  ( -13.35725562635141195, -26.51566270880198672, 13.67382249208304401 ) ) ;
#1484=CARTESIAN_POINT ( 'NONE',  ( -17.95583473709191580, -23.03132541760400898, 8.419927507916959541 ) ) ;
#1496=CARTESIAN_POINT ( 'NONE',  ( -20.04416526290808065, -25.17491895705300209, 39.48242750791695244 ) ) ;
#1498=CARTESIAN_POINT ( 'NONE',  ( -9.999999999999994671, -24.16482700510257686, 21.32617750791695599 ) ) ;
#1503=CARTESIAN_POINT ( 'NONE',  ( -10.58745947852648328, -26.35725562635138530, 7.986322492083041347 ) ) ;
#1506=CARTESIAN_POINT ( 'NONE',  ( -17.51566270880199738, -25.64274437364856496, 9.736322492083042235 ) ) ;
#1509=CARTESIAN_POINT ( 'NONE',  ( -12.94483980383665589, -18.39989183304783538, -8.139499971890162088E-17 ) ) ;
#1514=CARTESIAN_POINT ( 'NONE',  ( -15.00000000000001066, -19.99999999999997868, -4.814824860968089633E-32 ) ) ;
#1524=CARTESIAN_POINT ( 'NONE',  ( -16.50457296725820555, -28.95583473709189448, 7.107427507916955989 ) ) ;
#1525=CARTESIAN_POINT ( 'NONE',  ( -20.04416526290808065, -25.17491895705300209, 13.23242750791695777 ) ) ;
#1527=CARTESIAN_POINT ( 'NONE',  ( -9.955834737091903364, -25.17491895705294880, 7.767572492083041347 ) ) ;
#1529=CARTESIAN_POINT ( 'NONE',  ( -17.99999999999999645, -23.83517299489736985, 39.70117750791695954 ) ) ;
#1531=CARTESIAN_POINT ( 'NONE',  ( -13.49542703274178201, -19.04416526290806289, 4.482427507916958653 ) ) ;
#1542=CARTESIAN_POINT ( 'NONE',  ( -17.04047135212050890, -17.04416526290807710, 21.76757249208304401 ) ) ;
#1544=FILL_AREA_STYLE ('',( #13284 ) ) ;
#1548=CARTESIAN_POINT ( 'NONE',  ( -12.04416526290807887, -24.96867458239596260, 11.04492750791696132 ) ) ;
#1549=CARTESIAN_POINT ( 'NONE',  ( -8.855408670957602979, -27.35725562635137820, 2.736322492083039126 ) ) ;
#1570=CARTESIAN_POINT ( 'NONE',  ( -11.64274437364854187, -30.14459132904234195, 11.70117750791695777 ) ) ;
#1571=PLANE ( 'NONE',  #8360 ) ;
#1575=CARTESIAN_POINT ( 'NONE',  ( -15.16482700510262482, -20.99999999999997513, 16.73632249208304046 ) ) ;
#1581=CARTESIAN_POINT ( 'NONE',  ( -14.36097942780923731, -27.04416526290806999, 22.41992750791696309 ) ) ;
#1594=CARTESIAN_POINT ( 'NONE',  ( -18.53959229564986799, -20.21908421996107563, 40.35742750791696665 ) ) ;
#1597=CARTESIAN_POINT ( 'NONE',  ( -13.49542703274178379, -19.04416526290806289, 14.98242750791695777 ) ) ;
#1602=CARTESIAN_POINT ( 'NONE',  ( -16.17491895705296656, -29.04416526290807710, 14.33007249208304046 ) ) ;
#1605=CARTESIAN_POINT ( 'NONE',  ( -12.04416526290808420, -23.03132541760398766, 23.08007249208304401 ) ) ;
#1627=CARTESIAN_POINT ( 'NONE',  ( -15.16482700510259640, -28.99999999999998224, 22.63867750791695954 ) ) ;
#1628=CARTESIAN_POINT ( 'NONE',  ( -19.95583473709191580, -22.49542703274176603, 13.66992750791695599 ) ) ;
#1630=CARTESIAN_POINT ( 'NONE',  ( -10.75228648362912232, -21.35725562635138530, 1.861322492083040903 ) ) ;
#1633=CARTESIAN_POINT ( 'NONE',  ( -10.04416526290807710, -25.50457296725819489, 5.794927507916955989 ) ) ;
#1636=CARTESIAN_POINT ( 'NONE',  ( -16.17491895705301275, -18.95583473709189448, 14.54492750791695599 ) ) ;
#1648=CARTESIAN_POINT ( 'NONE',  ( -8.044165262908093084, -21.95952864787946979, 23.08007249208303691 ) ) ;
#1652=CARTESIAN_POINT ( 'NONE',  ( -12.31951028609537602, -22.64274437364854364, 15.63867750791696309 ) ) ;
#1654=CARTESIAN_POINT ( 'NONE',  ( -21.99999999999999289, -24.16482700510262305, 4.923822492083038682 ) ) ;
#1671=CARTESIAN_POINT ( 'NONE',  ( -15.16482700510258574, -30.99999999999998224, 12.13867750791695421 ) ) ;
#1674=CARTESIAN_POINT ( 'NONE',  ( -17.07549068051208963, -26.31681416490115311, 20.01757249208304401 ) ) ;
#1678=CARTESIAN_POINT ( 'NONE',  ( -14.36097942780923731, -27.04416526290806999, 17.16992750791696309 ) ) ;
#1681=CARTESIAN_POINT ( 'NONE',  ( -15.00000000000001954, -17.99999999999997868, -4.814824860968089633E-32 ) ) ;
#1690=CARTESIAN_POINT ( 'NONE',  ( -11.21908421996108629, -20.46040770435011069, 20.66992750791695244 ) ) ;
#1693=CARTESIAN_POINT ( 'NONE',  ( -17.35725562635140307, -28.41254052147349185, 19.79882249208304046 ) ) ;
#1695=CARTESIAN_POINT ( 'NONE',  ( -17.07549068051208963, -26.31681416490115311, 20.01757249208304401 ) ) ;
#1713=CARTESIAN_POINT ( 'NONE',  ( -19.24771351637089367, -21.35725562635142438, 24.38867750791695954 ) ) ;
#1718=CARTESIAN_POINT ( 'NONE',  ( -12.64274437364858628, -19.58745947852646552, 22.42382249208304401 ) ) ;
#1721=CARTESIAN_POINT ( 'NONE',  ( -19.24771351637089367, -21.35725562635142438, 3.388677507916958653 ) ) ;
#1723=CARTESIAN_POINT ( 'NONE',  ( -16.50457296725820555, -28.95583473709189803, 22.85742750791695954 ) ) ;
#1737=CARTESIAN_POINT ( 'NONE',  ( -20.97976432393974022, -27.64274437364858628, 20.23632249208303691 ) ) ;
#1739=CARTESIAN_POINT ( 'NONE',  ( -9.999999999999994671, -23.83517299489734143, 18.04882249208304401 ) ) ;
#1742=CARTESIAN_POINT ( 'NONE',  ( -17.07549068051210739, -21.68318583509881847, 19.35742750791695954 ) ) ;
#1744=CARTESIAN_POINT ( 'NONE',  ( -22.04416526290809486, -22.28918265808477628, 26.14257249208303691 ) ) ;
#1765=CARTESIAN_POINT ( 'NONE',  ( -18.64274437364853654, -29.97976432393976509, 17.82617750791695954 ) ) ;
#1769=CARTESIAN_POINT ( 'NONE',  ( -12.04416526290808420, -23.03132541760398766, 17.83007249208304046 ) ) ;
#1770=CARTESIAN_POINT ( 'NONE',  ( -9.996306089212364299, -29.24501739517662813, 0.9824275079169565439 ) ) ;
#1774=CARTESIAN_POINT ( 'NONE',  ( -16.64274437364856496, -26.51566270880199738, 23.07617750791695954 ) ) ;
#1790=CARTESIAN_POINT ( 'NONE',  ( -14.83517299489739649, -18.99999999999997868, 14.76367750791695777 ) ) ;
#1791=AXIS2_PLACEMENT_3D ( 'NONE', #13713, #4815, #7646 ) ;
#1795=CARTESIAN_POINT ( 'NONE',  ( -19.24771351637086880, -26.64274437364857206, 14.98632249208304046 ) ) ;
#1796=CARTESIAN_POINT ( 'NONE',  ( -12.92450931948790149, -21.68318583509881137, 17.39257249208304046 ) ) ;
#1814=CARTESIAN_POINT ( 'NONE',  ( -12.64274437364855252, -28.41254052147347053, 11.70117750791695777 ) ) ;
#1817=CARTESIAN_POINT ( 'NONE',  ( -11.46040770435014977, -20.21908421996103655, 17.39257249208304401 ) ) ;
#1819=CARTESIAN_POINT ( 'NONE',  ( -15.16482700510259640, -28.99999999999998224, 22.63867750791695954 ) ) ;
#1822=CARTESIAN_POINT ( 'NONE',  ( -12.64274437364855252, -28.41254052147347053, 16.95117750791695954 ) ) ;
#1834=CARTESIAN_POINT ( 'NONE',  ( -20.97976432393974022, -27.64274437364858628, 25.48632249208304401 ) ) ;
#1835=CARTESIAN_POINT ( 'NONE',  ( -14.83517299489735741, -28.99999999999998224, 14.11132249208304046 ) ) ;
#1837=CARTESIAN_POINT ( 'NONE',  ( -17.68048971390461688, -25.35725562635141372, 13.01367750791696132 ) ) ;
#1839=CARTESIAN_POINT ( 'NONE',  ( -16.71081734191520596, -31.04416526290808065, 14.33007249208304046 ) ) ;
#1860=CARTESIAN_POINT ( 'NONE',  ( -7.999999999999996447, -24.16482700510256976, 37.07617750791694533 ) ) ;
#1865=CARTESIAN_POINT ( 'NONE',  ( -17.51566270880199738, -25.64274437364856496, 14.98632249208304046 ) ) ;
#1866=CARTESIAN_POINT ( 'NONE',  ( -20.97976432393977575, -20.35725562635143504, 19.13867750791695954 ) ) ;
#1870=CARTESIAN_POINT ( 'NONE',  ( -11.95583473709191047, -23.36097942780921954, 21.10742750791696309 ) ) ;
#1891=CARTESIAN_POINT ( 'NONE',  ( -15.16482700510259640, -28.99999999999998224, 22.63867750791695954 ) ) ;
#1894=CARTESIAN_POINT ( 'NONE',  ( -13.82508104294702100, -18.95583473709188382, 22.20507249208304401 ) ) ;
#1896=CARTESIAN_POINT ( 'NONE',  ( -17.95583473709190869, -24.96867458239598037, 15.20507249208304579 ) ) ;
#1915=CARTESIAN_POINT ( 'NONE',  ( -11.21908421996108629, -20.46040770435011069, 20.66992750791695244 ) ) ;
#1917=CARTESIAN_POINT ( 'NONE',  ( -18.53959229564982536, -27.78091578003890660, 14.76757249208303691 ) ) ;
#1922=CARTESIAN_POINT ( 'NONE',  ( -19.95583473709191580, -22.49542703274176603, 13.66992750791695599 ) ) ;
#1924=CARTESIAN_POINT ( 'NONE',  ( -11.21908421996108984, -20.46040770435011069, 20.66992750791695599 ) ) ;
#1937=CARTESIAN_POINT ( 'NONE',  ( -7.999999999999996447, -23.83517299489733432, 28.54882249208303691 ) ) ;
#1938=CARTESIAN_POINT ( 'NONE',  ( -12.35725562635140307, -28.24771351637085459, 13.67382249208304223 ) ) ;
#1940=CARTESIAN_POINT ( 'NONE',  ( -12.92450931948788906, -26.31681416490114245, 32.48242750791695954 ) ) ;
#1943=CARTESIAN_POINT ( 'NONE',  ( -14.83517299489734853, -30.99999999999998224, 19.36132249208304046 ) ) ;
#1959=CARTESIAN_POINT ( 'NONE',  ( -20.97976432393977575, -20.35725562635143504, 29.63867750791695954 ) ) ;
#1962=CARTESIAN_POINT ( 'NONE',  ( -11.95583473709190514, -24.63902057219072361, 34.01757249208304046 ) ) ;
#1963=CARTESIAN_POINT ( 'NONE',  ( -8.855408670957631401, -20.64274437364852943, 15.63867750791696132 ) ) ;
#1970=CARTESIAN_POINT ( 'NONE',  ( -17.95583473709191580, -23.03132541760400898, 13.66992750791696309 ) ) ;
#1986=CARTESIAN_POINT ( 'NONE',  ( -9.955834737091912245, -22.82508104294696594, 26.35742750791695954 ) ) ;
#1989=CARTESIAN_POINT ( 'NONE',  ( -19.95583473709190514, -25.50457296725822687, 20.45507249208304401 ) ) ;
#1991=CARTESIAN_POINT ( 'NONE',  ( -12.92450931948790149, -21.68318583509881137, 22.64257249208304401 ) ) ;
#2005=CARTESIAN_POINT ( 'NONE',  ( -9.999999999999994671, -24.16482700510257686, 16.07617750791695954 ) ) ;
#2007=CARTESIAN_POINT ( 'NONE',  ( -9.955834737091903364, -25.17491895705294880, 13.01757249208304223 ) ) ;
#2011=CARTESIAN_POINT ( 'NONE',  ( -12.64274437364855252, -28.41254052147347053, 11.70117750791695777 ) ) ;
#2013=CARTESIAN_POINT ( 'NONE',  ( -19.95583473709191225, -22.49542703274176603, 24.16992750791695599 ) ) ;
#2015=CARTESIAN_POINT ( 'NONE',  ( -9.955834737091903364, -25.17491895705295235, 28.76757249208304401 ) ) ;
#2026=CARTESIAN_POINT ( 'NONE',  ( -20.24501739517669563, -18.99630608921239627, 26.58007249208304046 ) ) ;
#2027=CARTESIAN_POINT ( 'NONE',  ( -19.99999999999999645, -24.16482700510261949, 15.42382249208304046 ) ) ;
#2029=CARTESIAN_POINT ( 'NONE',  ( -17.07549068051210739, -21.68318583509881847, 29.85742750791696309 ) ) ;
#2031=CARTESIAN_POINT ( 'NONE',  ( -11.64274437364859693, -17.85540867095757989, 17.17382249208304046 ) ) ;
#2047=CARTESIAN_POINT ( 'NONE',  ( -9.996306089212364299, -29.24501739517662813, 27.23242750791696309 ) ) ;
#2053=CARTESIAN_POINT ( 'NONE',  ( -17.07549068051208963, -26.31681416490115311, 25.26757249208305112 ) ) ;
#2056=CARTESIAN_POINT ( 'NONE',  ( -9.754982604823348780, -18.99630608921234654, 15.41992750791695777 ) ) ;
#2061=CARTESIAN_POINT ( 'NONE',  ( -17.68048971390461688, -25.35725562635141372, 34.01367750791696665 ) ) ;
#2072=DIRECTION ( 'NONE',  ( 0.000000000000000000, 0.000000000000000000, -1.000000000000000000 ) ) ;
#2082=CARTESIAN_POINT ( 'NONE',  ( -10.58745947852649927, -21.64274437364853654, 31.38867750791696309 ) ) ;
#2085=CARTESIAN_POINT ( 'NONE',  ( -19.41254052147350961, -21.64274437364857562, 36.86132249208304046 ) ) ;
#2089=CARTESIAN_POINT ( 'NONE',  ( -12.31951028609536536, -25.35725562635139596, 39.48632249208304756 ) ) ;
#2107=CARTESIAN_POINT ( 'NONE',  ( -13.82508104294698192, -29.04416526290806644, 27.66992750791695244 ) ) ;
#2109=CARTESIAN_POINT ( 'NONE',  ( -10.04416526290808953, -22.49542703274172695, 12.58007249208304046 ) ) ;
#2111=CARTESIAN_POINT ( 'NONE',  ( -10.58745947852649927, -21.64274437364853654, 10.38867750791695777 ) ) ;
#2113=CARTESIAN_POINT ( 'NONE',  ( -12.35725562635143682, -19.75228648362908501, 25.70117750791695599 ) ) ;
#2115=CARTESIAN_POINT ( 'NONE',  ( -11.46040770435015332, -20.21908421996104011, 27.89257249208303691 ) ) ;
#2125=CARTESIAN_POINT ( 'NONE',  ( -9.754982604823302594, -29.00369391078756465, 34.45507249208304046 ) ) ;
#2126=CARTESIAN_POINT ( 'NONE',  ( -10.04416526290808598, -22.49542703274172695, 12.58007249208304046 ) ) ;
#2127=CARTESIAN_POINT ( 'NONE',  ( -11.95583473709191047, -23.36097942780921954, 26.35742750791696309 ) ) ;
#2129=CARTESIAN_POINT ( 'NONE',  ( -9.754982604823302594, -29.00369391078756465, 23.95507249208304046 ) ) ;
#2144=CARTESIAN_POINT ( 'NONE',  ( -12.95952864787955150, -17.04416526290805933, 30.73242750791696309 ) ) ;
#2148=CARTESIAN_POINT ( 'NONE',  ( -12.92450931948790149, -21.68318583509881137, 38.39257249208304756 ) ) ;
#2149=CARTESIAN_POINT ( 'NONE',  ( -21.99999999999999289, -23.83517299489739116, 18.70117750791695599 ) ) ;
#2155=CARTESIAN_POINT ( 'NONE',  ( -15.63902057219076269, -20.95583473709189448, 25.04492750791696309 ) ) ;
#2171=CARTESIAN_POINT ( 'NONE',  ( -18.78091578003889950, -27.53959229564985378, 33.79492750791696665 ) ) ;
#2174=CARTESIAN_POINT ( 'NONE',  ( -10.75228648362912232, -21.35725562635138530, 38.61132249208304046 ) ) ;
#2177=CARTESIAN_POINT ( 'NONE',  ( -14.03132541760400009, -26.95583473709189448, 29.64257249208304401 ) ) ;
#2194=CARTESIAN_POINT ( 'NONE',  ( -16.50457296725820555, -28.95583473709189448, 33.35742750791695954 ) ) ;
#2197=CARTESIAN_POINT ( 'NONE',  ( -18.78091578003892081, -20.46040770435013556, 37.08007249208304046 ) ) ;
#2202=CARTESIAN_POINT ( 'NONE',  ( -9.999999999999994671, -24.16482700510257686, 37.07617750791695954 ) ) ;
#2205=CARTESIAN_POINT ( 'NONE',  ( -12.64274437364855252, -28.41254052147347053, 37.95117750791695954 ) ) ;
#2208=CARTESIAN_POINT ( 'NONE',  ( -16.17491895705296656, -29.04416526290807354, 19.58007249208303691 ) ) ;
#2221=CARTESIAN_POINT ( 'NONE',  ( -17.68048971390461688, -25.35725562635141372, 23.51367750791696309 ) ) ;
#2224=CARTESIAN_POINT ( 'NONE',  ( -11.35725562635139418, -29.97976432393972601, 29.42382249208304046 ) ) ;
#2241=CARTESIAN_POINT ( 'NONE',  ( -21.99999999999999289, -23.83517299489739116, 29.20117750791695244 ) ) ;
#2247=CARTESIAN_POINT ( 'NONE',  ( -11.95583473709190514, -24.63902057219072361, 28.76757249208304401 ) ) ;
#2248=CARTESIAN_POINT ( 'NONE',  ( -17.04047135212043784, -30.95583473709190159, 17.60742750791695954 ) ) ;
#2254=CARTESIAN_POINT ( 'NONE',  ( -17.95583473709191580, -23.03132541760400898, 29.41992750791696665 ) ) ;
#2271=CARTESIAN_POINT ( 'NONE',  ( -16.17491895705301275, -18.95583473709189803, 35.54492750791695954 ) ) ;
#2275=CARTESIAN_POINT ( 'NONE',  ( -19.99999999999999645, -24.16482700510261949, 25.92382249208304401 ) ) ;
#2277=CARTESIAN_POINT ( 'NONE',  ( -15.63902057219073605, -27.04416526290807710, 30.08007249208304401 ) ) ;
#2290=CARTESIAN_POINT ( 'NONE',  ( -9.955834737091912245, -22.82508104294696594, 31.60742750791695954 ) ) ;
#2294=CARTESIAN_POINT ( 'NONE',  ( -16.17491895705296656, -29.04416526290807710, 35.33007249208301914 ) ) ;
#2296=CARTESIAN_POINT ( 'NONE',  ( -12.35725562635143682, -19.75228648362908501, 30.95117750791695954 ) ) ;
#2299=CARTESIAN_POINT ( 'NONE',  ( -20.04416526290808065, -25.17491895705300209, 28.98242750791695599 ) ) ;
#2301=CARTESIAN_POINT ( 'NONE',  ( -17.35725562635140307, -28.41254052147349185, 30.29882249208304401 ) ) ;
#2312=CARTESIAN_POINT ( 'NONE',  ( -14.83517299489738761, -20.99999999999997513, 35.76367750791695954 ) ) ;
#2313=APPLICATION_CONTEXT ( 'automotive_design' ) ;
#2315=CARTESIAN_POINT ( 'NONE',  ( -9.754982604823302594, -29.00369391078756465, 39.70507249208304046 ) ) ;
#2331=CARTESIAN_POINT ( 'NONE',  ( -15.16482700510264436, -16.99999999999997868, 0.9863224920830391262 ) ) ;
#2335=CARTESIAN_POINT ( 'NONE',  ( -15.63902057219073605, -27.04416526290807710, 35.33007249208304046 ) ) ;
#2337=CARTESIAN_POINT ( 'NONE',  ( -14.83517299489740715, -16.99999999999997868, 25.26367750791695954 ) ) ;
#2360=CARTESIAN_POINT ( 'NONE',  ( -19.41254052147348830, -26.35725562635142083, 28.76367750791695954 ) ) ;
#2363=CARTESIAN_POINT ( 'NONE',  ( -15.16482700510263371, -18.99999999999997868, 27.23632249208304046 ) ) ;
#2366=CARTESIAN_POINT ( 'NONE',  ( -17.31681416490117087, -21.92450931948788551, 31.83007249208304046 ) ) ;
#2383=CARTESIAN_POINT ( 'NONE',  ( -11.21908421996108629, -20.46040770435011069, 36.41992750791695954 ) ) ;
#2385=CARTESIAN_POINT ( 'NONE',  ( -19.95583473709190514, -25.50457296725822687, 30.95507249208303691 ) ) ;
#2387=CARTESIAN_POINT ( 'NONE',  ( -18.53959229564986799, -20.21908421996107563, 24.60742750791695954 ) ) ;
#2390=CARTESIAN_POINT ( 'NONE',  ( -15.16482700510259640, -28.99999999999998224, 27.88867750791695954 ) ) ;
#2392=CARTESIAN_POINT ( 'NONE',  ( -19.41254052147350961, -21.64274437364857562, 31.61132249208303691 ) ) ;
#2403=CARTESIAN_POINT ( 'NONE',  ( -17.51566270880201159, -22.35725562635141728, 40.13867750791696665 ) ) ;
#2405=CARTESIAN_POINT ( 'NONE',  ( -17.04047135212050890, -17.04416526290807710, 32.26757249208304046 ) ) ;
#2419=CARTESIAN_POINT ( 'NONE',  ( -21.99999999999999289, -23.83517299489739116, 39.70117750791695954 ) ) ;
#2424=CARTESIAN_POINT ( 'NONE',  ( -14.83517299489738761, -20.99999999999997513, -0.9863224920830401254 ) ) ;
#2425=CARTESIAN_POINT ( 'NONE',  ( -15.16482700510258574, -30.99999999999998224, 27.88867750791695954 ) ) ;
#2446=CARTESIAN_POINT ( 'NONE',  ( -14.83517299489740715, -16.99999999999997868, 4.263677507916957765 ) ) ;
#2450=CARTESIAN_POINT ( 'NONE',  ( -15.16482700510263371, -18.99999999999997868, 42.98632249208304046 ) ) ;
#2455=CARTESIAN_POINT ( 'NONE',  ( -18.04416526290808775, -23.36097942780924441, 26.14257249208303691 ) ) ;
#2464=CARTESIAN_POINT ( 'NONE',  ( -17.64274437364855430, -28.24771351637087236, 33.57617750791696665 ) ) ;
#2466=CARTESIAN_POINT ( 'NONE',  ( -14.83517299489739649, -18.99999999999997868, 4.263677507916958653 ) ) ;
#2470=CARTESIAN_POINT ( 'NONE',  ( -22.04416526290809486, -22.28918265808477628, 26.14257249208303691 ) ) ;
#2471=CARTESIAN_POINT ( 'NONE',  ( -9.999999999999994671, -24.16482700510257686, 37.07617750791695954 ) ) ;
#2475=CARTESIAN_POINT ( 'NONE',  ( -11.46040770435014977, -20.21908421996103655, 38.39257249208301914 ) ) ;
#2478=CARTESIAN_POINT ( 'NONE',  ( -9.955834737091912245, -22.82508104294696594, 26.35742750791695954 ) ) ;
#2481=CARTESIAN_POINT ( 'NONE',  ( -18.53959229564986799, -20.21908421996107563, 35.10742750791695244 ) ) ;
#2483=CARTESIAN_POINT ( 'NONE',  ( -10.75228648362912232, -21.35725562635138530, 38.61132249208304046 ) ) ;
#2496=CARTESIAN_POINT ( 'NONE',  ( -19.99999999999999645, -23.83517299489738051, 2.951177507916958209 ) ) ;
#2498=CARTESIAN_POINT ( 'NONE',  ( -8.855408670957602979, -27.35725562635137820, 34.23632249208304046 ) ) ;
#2515=CARTESIAN_POINT ( 'NONE',  ( -12.95952864787948755, -30.95583473709188382, 3.392572492083039570 ) ) ;
#2522=CARTESIAN_POINT ( 'NONE',  ( -18.04416526290808420, -24.63902057219074493, 7.982427507916962206 ) ) ;
#2523=CARTESIAN_POINT ( 'NONE',  ( -20.97976432393977575, -20.35725562635143504, 34.88867750791695954 ) ) ;
#2545=CARTESIAN_POINT ( 'NONE',  ( -16.71081734191527346, -16.95583473709190159, 9.294927507916959541 ) ) ;
#2550=CARTESIAN_POINT ( 'NONE',  ( -14.03132541760400009, -26.95583473709189448, 3.392572492083043567 ) ) ;
#2554=CARTESIAN_POINT ( 'NONE',  ( -17.51566270880201159, -22.35725562635141728, 3.388677507916959986 ) ) ;
#2565=CARTESIAN_POINT ( 'NONE',  ( -18.78091578003889950, -27.53959229564985378, 33.79492750791696665 ) ) ;
#2567=CARTESIAN_POINT ( 'NONE',  ( -12.64274437364855252, -28.41254052147347053, 6.451177507916959541 ) ) ;
#2571=CARTESIAN_POINT ( 'NONE',  ( -10.04416526290808953, -22.49542703274172695, 7.330072492083041347 ) ) ;
#2572=CARTESIAN_POINT ( 'NONE',  ( -20.97976432393977575, -20.35725562635143504, 8.638677507916955989 ) ) ;
#2575=CARTESIAN_POINT ( 'NONE',  ( -20.04416526290809131, -22.82508104294699791, 36.64257249208304046 ) ) ;
#2579=CARTESIAN_POINT ( 'NONE',  ( -13.82508104294698192, -29.04416526290806644, 32.91992750791695954 ) ) ;
#2583=CARTESIAN_POINT ( 'NONE',  ( -13.82508104294702100, -18.95583473709188382, 37.95507249208304046 ) ) ;
#2593=CARTESIAN_POINT ( 'NONE',  ( -9.955834737091912245, -22.82508104294696594, 5.357427507916956877 ) ) ;
#2596=CARTESIAN_POINT ( 'NONE',  ( -9.020235676060250896, -20.35725562635137820, 33.36132249208304046 ) ) ;
#2598=CARTESIAN_POINT ( 'NONE',  ( -15.96867458239597326, -26.95583473709190159, 33.35742750791695954 ) ) ;
#2599=CARTESIAN_POINT ( 'NONE',  ( -17.35725562635144215, -19.58745947852648683, 3.826177507916958209 ) ) ;
#2608=CARTESIAN_POINT ( 'NONE',  ( -9.020235676060250896, -20.35725562635137820, 1.861322492083039126 ) ) ;
#2612=CARTESIAN_POINT ( 'NONE',  ( -15.96867458239597326, -26.95583473709190159, 7.107427507916960430 ) ) ;
#2613=CARTESIAN_POINT ( 'NONE',  ( -21.14459132904236327, -27.35725562635143149, 28.76367750791696309 ) ) ;
#2634=CARTESIAN_POINT ( 'NONE',  ( -14.83517299489739649, -18.99999999999997868, 41.01367750791696665 ) ) ;
#2640=CARTESIAN_POINT ( 'NONE',  ( -18.78091578003892081, -20.46040770435013556, 42.33007249208301914 ) ) ;
#2641=EDGE_CURVE ( 'NONE', #13312, #18550, #10633, .T. ) ;
#2644=CARTESIAN_POINT ( 'NONE',  ( -17.51566270880201159, -22.35725562635141728, 8.638677507916959541 ) ) ;
#2658=CARTESIAN_POINT ( 'NONE',  ( -16.50457296725820555, -28.95583473709189448, 28.10742750791695954 ) ) ;
#2664=CARTESIAN_POINT ( 'NONE',  ( -21.14459132904239169, -20.64274437364858628, 42.11132249208304046 ) ) ;
#2666=CARTESIAN_POINT ( 'NONE',  ( -17.64274437364855430, -28.24771351637087236, 38.82617750791695954 ) ) ;
#2669=CARTESIAN_POINT ( 'NONE',  ( -13.64274437364857739, -21.31951028609534760, 1.423822492083042901 ) ) ;
#2674=CARTESIAN_POINT ( 'NONE',  ( -19.99999999999999645, -23.83517299489738051, 39.70117750791695954 ) ) ;
#2676=CARTESIAN_POINT ( 'NONE',  ( -11.21908421996106142, -27.53959229564982181, 34.45507249208304046 ) ) ;
#2691=CARTESIAN_POINT ( 'NONE',  ( -16.17491895705301275, -18.95583473709189803, 9.294927507916954212 ) ) ;
#2692=CARTESIAN_POINT ( 'NONE',  ( -18.04416526290808420, -24.63902057219074493, 39.48242750791696665 ) ) ;
#2694=CARTESIAN_POINT ( 'NONE',  ( -15.16482700510263371, -18.99999999999997868, 6.236322492083041347 ) ) ;
#2699=CARTESIAN_POINT ( 'NONE',  ( -12.31951028609537602, -22.64274437364854364, 31.38867750791696309 ) ) ;
#2712=CARTESIAN_POINT ( 'NONE',  ( -21.14459132904239169, -20.64274437364858628, 5.361322492083039570 ) ) ;
#2713=( LENGTH_UNIT ( ) NAMED_UNIT ( * ) SI_UNIT ( .MILLI., .METRE. ) );
#2715=CARTESIAN_POINT ( 'NONE',  ( -11.46040770435015332, -20.21908421996104011, 1.642572492083041125 ) ) ;
#2718=CARTESIAN_POINT ( 'NONE',  ( -17.99999999999999645, -23.83517299489736985, 2.951177507916960430 ) ) ;
#2719=CARTESIAN_POINT ( 'NONE',  ( -9.996306089212364299, -29.24501739517662813, 37.73242750791695244 ) ) ;
#2725=( GEOMETRIC_REPRESENTATION_CONTEXT ( 3 ) GLOBAL_UNCERTAINTY_ASSIGNED_CONTEXT ( ( #5516 ) ) GLOBAL_UNIT_ASSIGNED_CONTEXT ( ( #2713, #5857, #7224 ) ) REPRESENTATION_CONTEXT ( 'NONE', 'WORKASPACE' ) );
#2739=CARTESIAN_POINT ( 'NONE',  ( -20.24501739517664234, -29.00369391078761439, 7.544927507916956877 ) ) ;
#2743=CARTESIAN_POINT ( 'NONE',  ( -9.999999999999994671, -23.83517299489734143, 39.04882249208304046 ) ) ;
#2746=CARTESIAN_POINT ( 'NONE',  ( -12.68318583509884157, -21.92450931948787485, -0.3300724920830400699 ) ) ;
#2755=CARTESIAN_POINT ( 'NONE',  ( -10.58745947852649927, -21.64274437364853654, 20.88867750791695954 ) ) ;
#2757=CARTESIAN_POINT ( 'NONE',  ( -13.49542703274178379, -19.04416526290806289, 4.482427507916957765 ) ) ;
#2762=CARTESIAN_POINT ( 'NONE',  ( -20.04416526290809131, -22.82508104294699791, 5.142572492083038682 ) ) ;
#2763=CARTESIAN_POINT ( 'NONE',  ( -11.35725562635144925, -18.02023567606020293, 9.951177507916955989 ) ) ;
#2765=CARTESIAN_POINT ( 'NONE',  ( -18.53959229564982536, -27.78091578003890660, 41.01757249208304046 ) ) ;
#2775=CARTESIAN_POINT ( 'NONE',  ( -14.83517299489735741, -28.99999999999998224, 40.36132249208304046 ) ) ;
#2785=CARTESIAN_POINT ( 'NONE',  ( -11.21908421996108629, -20.46040770435011069, -0.3300724920830416798 ) ) ;
#2787=CARTESIAN_POINT ( 'NONE',  ( -16.17491895705301275, -18.95583473709189803, 14.54492750791695421 ) ) ;
#2790=CARTESIAN_POINT ( 'NONE',  ( -13.82508104294702100, -18.95583473709188382, 11.70507249208303868 ) ) ;
#2793=CARTESIAN_POINT ( 'NONE',  ( -11.21908421996108629, -20.46040770435011069, 4.919927507916955989 ) ) ;
#2794=CARTESIAN_POINT ( 'NONE',  ( -11.21908421996108984, -20.46040770435011069, 4.919927507916956877 ) ) ;
#2808=CARTESIAN_POINT ( 'NONE',  ( -18.35725562635138886, -30.14459132904237393, 14.54882249208303868 ) ) ;
#2814=CARTESIAN_POINT ( 'NONE',  ( -13.35725562635142794, -21.48433729119796709, -0.5488224920830401254 ) ) ;
#2815=CARTESIAN_POINT ( 'NONE',  ( -13.28918265808478694, -16.95583473709189093, 6.455072492083038682 ) ) ;
#2836=CARTESIAN_POINT ( 'NONE',  ( -9.996306089212364299, -29.24501739517662813, 0.9824275079169565439 ) ) ;
#2841=CARTESIAN_POINT ( 'NONE',  ( -17.64274437364858983, -19.75228648362910633, 42.54882249208304046 ) ) ;
#2846=CARTESIAN_POINT ( 'NONE',  ( -13.35725562635142794, -21.48433729119796709, -0.5488224920830401254 ) ) ;
#2858=CARTESIAN_POINT ( 'NONE',  ( -10.75228648362910100, -26.64274437364854009, 27.01367750791695954 ) ) ;
#2861=CARTESIAN_POINT ( 'NONE',  ( -16.17491895705301275, -18.95583473709189803, 9.294927507916954212 ) ) ;
#2864=CARTESIAN_POINT ( 'NONE',  ( -19.41254052147350961, -21.64274437364857562, 5.361322492083041347 ) ) ;
#2866=CARTESIAN_POINT ( 'NONE',  ( -20.04416526290808065, -25.17491895705300209, 39.48242750791695244 ) ) ;
#2868=CARTESIAN_POINT ( 'NONE',  ( -17.99999999999999645, -24.16482700510260173, 4.923822492083043123 ) ) ;
#2872=CARTESIAN_POINT ( 'NONE',  ( -11.89515593330241749, -18.98492275559260989, 1.100789300500590883E-12 ) ) ;
#2874=CARTESIAN_POINT ( 'NONE',  ( -11.46040770435012668, -27.78091578003887463, 37.73242750791694533 ) ) ;
#2878=CARTESIAN_POINT ( 'NONE',  ( -11.21908421996106142, -27.53959229564982181, 39.70507249208304046 ) ) ;
#2889=CARTESIAN_POINT ( 'NONE',  ( -13.49542703274178379, -19.04416526290806289, -0.7675724920830416798 ) ) ;
#2891=CARTESIAN_POINT ( 'NONE',  ( -19.99999999999999645, -23.83517299489738051, 18.70117750791695954 ) ) ;
#2894=CARTESIAN_POINT ( 'NONE',  ( -11.21908421996106320, -27.53959229564982181, 8.205072492083036906 ) ) ;
#2896=CARTESIAN_POINT ( 'NONE',  ( -19.95583473709191580, -22.49542703274176603, 8.419927507916955989 ) ) ;
#2897=CARTESIAN_POINT ( 'NONE',  ( -12.35725562635143682, -19.75228648362908501, 4.701177507916957765 ) ) ;
#2909=CARTESIAN_POINT ( 'NONE',  ( -8.855408670957602979, -27.35725562635137820, 23.73632249208303691 ) ) ;
#2914=CARTESIAN_POINT ( 'NONE',  ( -11.95583473709191047, -23.36097942780921954, 21.10742750791696309 ) ) ;
#2916=CARTESIAN_POINT ( 'NONE',  ( -20.00369391078757886, -29.24501739517668142, 9.517572492083038682 ) ) ;
#2924=CARTESIAN_POINT ( 'NONE',  ( -14.11162457711532703, -20.06223238837476330, 1.106825084037506213E-14 ) ) ;
#2935=CARTESIAN_POINT ( 'NONE',  ( -8.044165262908075320, -26.04047135212042718, 21.54492750791695599 ) ) ;
#2936=FACE_OUTER_BOUND ( 'NONE', #12656, .T. ) ;
#2939=CARTESIAN_POINT ( 'NONE',  ( -12.92450931948790149, -21.68318583509881137, 22.64257249208304401 ) ) ;
#2943=CARTESIAN_POINT ( 'NONE',  ( -16.64274437364856496, -26.51566270880199738, 7.326177507916959541 ) ) ;
#2957=CARTESIAN_POINT ( 'NONE',  ( -19.99999999999999645, -23.83517299489738051, 18.70117750791695954 ) ) ;
#2960=CARTESIAN_POINT ( 'NONE',  ( -13.49542703274174116, -28.95583473709188738, 3.392572492083040903 ) ) ;
#2962=CARTESIAN_POINT ( 'NONE',  ( -13.49542703274174116, -28.95583473709188738, 40.14257249208304756 ) ) ;
#2975=SURFACE_STYLE_USAGE ( .BOTH. , #1416 ) ;
#2981=CARTESIAN_POINT ( 'NONE',  ( -13.49542703274178379, -19.04416526290806289, 9.732427507916959541 ) ) ;
#2982=CARTESIAN_POINT ( 'NONE',  ( -16.17491895705301275, -18.95583473709189803, 19.79492750791695954 ) ) ;
#2984=CARTESIAN_POINT ( 'NONE',  ( -12.64274437364858628, -19.58745947852646552, 6.673822492083040459 ) ) ;
#2986=CARTESIAN_POINT ( 'NONE',  ( -18.78091578003889950, -27.53959229564985378, 2.294927507916958209 ) ) ;
#2989=CARTESIAN_POINT ( 'NONE',  ( -14.83517299489739649, -18.99999999999997868, 4.263677507916958653 ) ) ;
#3002=CARTESIAN_POINT ( 'NONE',  ( -21.14459132904239169, -20.64274437364858628, 15.86132249208304223 ) ) ;
#3006=CARTESIAN_POINT ( 'NONE',  ( -9.999999999999994671, -23.83517299489734143, 2.298822492083040903 ) ) ;
#3010=CARTESIAN_POINT ( 'NONE',  ( -17.99999999999999645, -23.83517299489736985, 18.70117750791695599 ) ) ;
#3012=CARTESIAN_POINT ( 'NONE',  ( -18.64274437364853654, -29.97976432393976509, 38.82617750791695244 ) ) ;
#3032=CARTESIAN_POINT ( 'NONE',  ( -9.996306089212364299, -29.24501739517662813, 11.48242750791695777 ) ) ;
#3036=CARTESIAN_POINT ( 'NONE',  ( -14.36097942780925685, -20.95583473709189093, 11.70507249208304223 ) ) ;
#3044=CARTESIAN_POINT ( 'NONE',  ( -17.95583473709191580, -23.03132541760400898, 18.91992750791695954 ) ) ;
#3056=CARTESIAN_POINT ( 'NONE',  ( -18.78091578003889950, -27.53959229564985378, 23.29492750791695954 ) ) ;
#3060=CARTESIAN_POINT ( 'NONE',  ( -11.21908421996106320, -27.53959229564982181, 23.95507249208304401 ) ) ;
#3064=CARTESIAN_POINT ( 'NONE',  ( -16.64274437364858272, -21.48433729119797420, 11.04882249208304223 ) ) ;
#3067=CARTESIAN_POINT ( 'NONE',  ( -14.39797529960427269, -18.02527416137649396, 9.743381756881009494E-15 ) ) ;
#3080=CARTESIAN_POINT ( 'NONE',  ( -17.35725562635144215, -19.58745947852648683, 3.826177507916958209 ) ) ;
#3081=CARTESIAN_POINT ( 'NONE',  ( -16.50457296725820555, -28.95583473709189448, 12.35742750791695954 ) ) ;
#3083=CARTESIAN_POINT ( 'NONE',  ( -21.99999999999999289, -24.16482700510262305, 41.67382249208304756 ) ) ;
#3085=CARTESIAN_POINT ( 'NONE',  ( -20.04416526290808065, -25.17491895705300209, 7.982427507916958653 ) ) ;
#3087=CARTESIAN_POINT ( 'NONE',  ( -9.999999999999994671, -24.16482700510257686, 21.32617750791695599 ) ) ;
#3102=CARTESIAN_POINT ( 'NONE',  ( -16.71081734191520596, -31.04416526290808065, 19.58007249208303691 ) ) ;
#3105=CARTESIAN_POINT ( 'NONE',  ( -10.58745947852648328, -26.35725562635138530, 2.736322492083041347 ) ) ;
#3108=CARTESIAN_POINT ( 'NONE',  ( -14.03132541760401786, -21.04416526290806289, 14.98242750791695954 ) ) ;
#3110=CARTESIAN_POINT ( 'NONE',  ( -11.64274437364859693, -17.85540867095757989, 6.673822492083038682 ) ) ;
#3120=CARTESIAN_POINT ( 'NONE',  ( -13.46816481875853277, -20.24306461418997216, 1.106825084037506055E-14 ) ) ;
#3130=CARTESIAN_POINT ( 'NONE',  ( -9.754982604823348780, -18.99630608921234654, 10.16992750791695777 ) ) ;
#3135=CARTESIAN_POINT ( 'NONE',  ( -16.64274437364858272, -21.48433729119797420, 16.29882249208304401 ) ) ;
#3141=CARTESIAN_POINT ( 'NONE',  ( -17.68048971390461688, -25.35725562635141372, 23.51367750791696309 ) ) ;
#3144=ORIENTED_EDGE ( 'NONE', *, *, #7068, .T. ) ;
#3154=CARTESIAN_POINT ( 'NONE',  ( -9.999999999999994671, -24.16482700510257686, 37.07617750791695954 ) ) ;
#3158=CARTESIAN_POINT ( 'NONE',  ( -10.75228648362910100, -26.64274437364854009, 16.51367750791695954 ) ) ;
#3163=CARTESIAN_POINT ( 'NONE',  ( -10.04416526290808953, -22.49542703274172695, 17.83007249208303691 ) ) ;
#3166=CARTESIAN_POINT ( 'NONE',  ( -13.64274437364857739, -21.31951028609534760, 11.92382249208304401 ) ) ;
#3187=CARTESIAN_POINT ( 'NONE',  ( -19.99999999999999645, -23.83517299489738051, 23.95117750791695954 ) ) ;
#3188=CARTESIAN_POINT ( 'NONE',  ( -15.16482700510259640, -28.99999999999998224, 12.13867750791695777 ) ) ;
#3190=CARTESIAN_POINT ( 'NONE',  ( -12.35725562635140307, -28.24771351637085459, 13.67382249208304223 ) ) ;
#3192=CARTESIAN_POINT ( 'NONE',  ( -13.49542703274178379, -19.04416526290806289, 4.482427507916957765 ) ) ;
#3194=CARTESIAN_POINT ( 'NONE',  ( -19.41254052147348830, -26.35725562635142083, 13.01367750791695777 ) ) ;
#3209=CARTESIAN_POINT ( 'NONE',  ( -8.044165262908093084, -21.95952864787946979, 17.83007249208304046 ) ) ;
#3211=CARTESIAN_POINT ( 'NONE',  ( -10.04416526290808598, -22.49542703274172695, 17.83007249208304046 ) ) ;
#3214=CARTESIAN_POINT ( 'NONE',  ( -17.51566270880201159, -22.35725562635141728, 19.13867750791695954 ) ) ;
#3217=CARTESIAN_POINT ( 'NONE',  ( -20.24501739517664234, -29.00369391078761439, 39.04492750791695954 ) ) ;
#3233=CARTESIAN_POINT ( 'NONE',  ( -12.95952864787955150, -17.04416526290805933, 14.98242750791695777 ) ) ;
#3237=CARTESIAN_POINT ( 'NONE',  ( -15.16482700510262482, -20.99999999999997513, 21.98632249208304046 ) ) ;
#3238=CARTESIAN_POINT ( 'NONE',  ( -15.16482700510258574, -30.99999999999998224, 6.888677507916956877 ) ) ;
#3242=CARTESIAN_POINT ( 'NONE',  ( -12.92450931948788906, -26.31681416490114245, 11.48242750791695954 ) ) ;
#3256=CARTESIAN_POINT ( 'NONE',  ( -11.46040770435012668, -27.78091578003887463, 37.73242750791694533 ) ) ;
#3259=CARTESIAN_POINT ( 'NONE',  ( -12.64274437364855252, -28.41254052147347053, 16.95117750791695954 ) ) ;
#3263=CARTESIAN_POINT ( 'NONE',  ( -13.82508104294702100, -18.95583473709188382, 16.95507249208304046 ) ) ;
#3266=CARTESIAN_POINT ( 'NONE',  ( -17.51566270880199738, -25.64274437364856496, 14.98632249208304046 ) ) ;
#3284=CARTESIAN_POINT ( 'NONE',  ( -13.49542703274178379, -19.04416526290806289, 14.98242750791695777 ) ) ;
#3287=CARTESIAN_POINT ( 'NONE',  ( -18.78091578003892081, -20.46040770435013556, 16.08007249208304401 ) ) ;
#3291=CARTESIAN_POINT ( 'NONE',  ( -10.75228648362910100, -26.64274437364854009, 16.51367750791695954 ) ) ;
#3294=CARTESIAN_POINT ( 'NONE',  ( -12.64274437364855252, -28.41254052147347053, 22.20117750791695599 ) ) ;
#3307=CARTESIAN_POINT ( 'NONE',  ( -17.04047135212050890, -17.04416526290807710, 32.26757249208304046 ) ) ;
#3308=CARTESIAN_POINT ( 'NONE',  ( -20.04416526290809131, -22.82508104294700502, 5.142572492083039570 ) ) ;
#3311=CARTESIAN_POINT ( 'NONE',  ( -18.04416526290808420, -24.63902057219074493, 13.23242750791696132 ) ) ;
#3314=CARTESIAN_POINT ( 'NONE',  ( -15.16482700510264436, -16.99999999999997868, 16.73632249208304046 ) ) ;
#3335=CARTESIAN_POINT ( 'NONE',  ( -17.04047135212043784, -30.95583473709190159, 17.60742750791695954 ) ) ;
#3339=CARTESIAN_POINT ( 'NONE',  ( -12.04416526290808420, -23.03132541760398766, 23.08007249208304401 ) ) ;
#3340=CARTESIAN_POINT ( 'NONE',  ( -15.16482700510258574, -30.99999999999998224, 17.38867750791695599 ) ) ;
#3344=CARTESIAN_POINT ( 'NONE',  ( -18.04416526290808420, -24.63902057219074493, 18.48242750791695954 ) ) ;
#3358=CARTESIAN_POINT ( 'NONE',  ( -18.53959229564986799, -20.21908421996107563, 35.10742750791694533 ) ) ;
#3361=CARTESIAN_POINT ( 'NONE',  ( -18.78091578003889950, -27.53959229564985378, 18.04492750791695954 ) ) ;
#3365=CARTESIAN_POINT ( 'NONE',  ( -18.53959229564982536, -27.78091578003890660, 14.76757249208303691 ) ) ;
#3366=CARTESIAN_POINT ( 'NONE',  ( -12.92450931948790149, -21.68318583509881137, 12.14257249208304223 ) ) ;
#3379=CARTESIAN_POINT ( 'NONE',  ( -19.99999999999999645, -23.83517299489738051, 13.45117750791695777 ) ) ;
#3382=CARTESIAN_POINT ( 'NONE',  ( -19.24771351637086880, -26.64274437364857206, 20.23632249208304046 ) ) ;
#3384=CARTESIAN_POINT ( 'NONE',  ( -9.955834737091912245, -22.82508104294696594, 15.85742750791695777 ) ) ;
#3386=CARTESIAN_POINT ( 'NONE',  ( -18.53959229564986799, -20.21908421996107563, 19.35742750791695954 ) ) ;
#3400=CARTESIAN_POINT ( 'NONE',  ( -15.16482700510264436, -16.99999999999997868, 32.48632249208304046 ) ) ;
#3401=CARTESIAN_POINT ( 'NONE',  ( -13.82508104294702100, -18.95583473709188382, 11.70507249208304046 ) ) ;
#3403=CARTESIAN_POINT ( 'NONE',  ( -16.35725562635142794, -21.31951028609535470, 24.82617750791696309 ) ) ;
#3405=CARTESIAN_POINT ( 'NONE',  ( -7.999999999999996447, -23.83517299489733432, 23.29882249208304046 ) ) ;
#3423=CARTESIAN_POINT ( 'NONE',  ( -7.955834737091916686, -22.28918265808470522, 31.60742750791695244 ) ) ;
#3428=CARTESIAN_POINT ( 'NONE',  ( -13.35725562635141195, -26.51566270880198672, 29.42382249208304401 ) ) ;
#3429=CARTESIAN_POINT ( 'NONE',  ( -12.95952864787955150, -17.04416526290805933, 20.23242750791695954 ) ) ;
#3433=CARTESIAN_POINT ( 'NONE',  ( -13.64274437364856141, -26.68048971390460622, 11.70117750791696132 ) ) ;
#3453=CARTESIAN_POINT ( 'NONE',  ( -13.82508104294698192, -29.04416526290806644, 32.91992750791695954 ) ) ;
#3457=CARTESIAN_POINT ( 'NONE',  ( -19.41254052147350961, -21.64274437364857562, 15.86132249208304223 ) ) ;
#3460=CARTESIAN_POINT ( 'NONE',  ( -14.36097942780925685, -20.95583473709189093, 22.20507249208304401 ) ) ;
#3478=CARTESIAN_POINT ( 'NONE',  ( -9.999999999999994671, -24.16482700510257686, 10.82617750791695777 ) ) ;
#3480=CARTESIAN_POINT ( 'NONE',  ( -15.16482700510263371, -18.99999999999997868, 21.98632249208304401 ) ) ;
#3483=CARTESIAN_POINT ( 'NONE',  ( -18.53959229564986799, -20.21908421996107563, 19.35742750791695599 ) ) ;
#3485=CARTESIAN_POINT ( 'NONE',  ( -18.78091578003889595, -27.53959229564985023, 23.29492750791695954 ) ) ;
#3487=CARTESIAN_POINT ( 'NONE',  ( -17.64274437364858983, -19.75228648362910633, 32.04882249208304046 ) ) ;
#3501=CARTESIAN_POINT ( 'NONE',  ( -20.00369391078757886, -29.24501739517668142, 35.76757249208303335 ) ) ;
#3503=CARTESIAN_POINT ( 'NONE',  ( -9.955834737091903364, -25.17491895705295235, 13.01757249208304223 ) ) ;
#3505=CARTESIAN_POINT ( 'NONE',  ( -17.95583473709191580, -23.03132541760400898, 24.16992750791696309 ) ) ;
#3508=CARTESIAN_POINT ( 'NONE',  ( -16.71081734191520596, -31.04416526290808065, 24.83007249208304046 ) ) ;
#3526=CARTESIAN_POINT ( 'NONE',  ( -14.83517299489740715, -16.99999999999997868, 30.51367750791695954 ) ) ;
#3529=CARTESIAN_POINT ( 'NONE',  ( -18.04416526290808775, -23.36097942780924441, 36.64257249208304756 ) ) ;
#3530=CARTESIAN_POINT ( 'NONE',  ( -17.04047135212043784, -30.95583473709190159, 22.85742750791695599 ) ) ;
#3534=CARTESIAN_POINT ( 'NONE',  ( -12.48433729119798130, -25.64274437364855075, 37.51367750791695954 ) ) ;
#3552=CARTESIAN_POINT ( 'NONE',  ( -15.16482700510259640, -28.99999999999998224, 33.13867750791696665 ) ) ;
#3555=CARTESIAN_POINT ( 'NONE',  ( -10.58745947852648328, -26.35725562635138530, 34.23632249208304046 ) ) ;
#3557=CARTESIAN_POINT ( 'NONE',  ( -12.31951028609536536, -25.35725562635139596, 18.48632249208304401 ) ) ;
#3570=CARTESIAN_POINT ( 'NONE',  ( -15.16482700510259640, -28.99999999999998224, 38.38867750791695954 ) ) ;
#3573=CARTESIAN_POINT ( 'NONE',  ( -19.95583473709190514, -25.50457296725822687, 15.20507249208304046 ) ) ;
#3577=CARTESIAN_POINT ( 'NONE',  ( -19.95583473709191580, -22.49542703274176603, 18.91992750791694888 ) ) ;
#3579=CARTESIAN_POINT ( 'NONE',  ( -16.50457296725820555, -28.95583473709189803, 28.10742750791695954 ) ) ;
#3581=CARTESIAN_POINT ( 'NONE',  ( -19.41254052147350961, -21.64274437364857562, 21.11132249208304401 ) ) ;
#3591=CARTESIAN_POINT ( 'NONE',  ( -20.24501739517669563, -18.99630608921239627, 37.08007249208304046 ) ) ;
#3592=CARTESIAN_POINT ( 'NONE',  ( -20.04416526290809131, -22.82508104294700502, 10.39257249208303868 ) ) ;
#3593=CARTESIAN_POINT ( 'NONE',  ( -15.16482700510260706, -26.99999999999998579, 33.13867750791695954 ) ) ;
#3595=CARTESIAN_POINT ( 'NONE',  ( -11.64274437364859693, -17.85540867095757989, 22.42382249208304046 ) ) ;
#3615=CARTESIAN_POINT ( 'NONE',  ( -22.04416526290807710, -25.71081734191525925, 34.23242750791695244 ) ) ;
#3621=CARTESIAN_POINT ( 'NONE',  ( -14.36097942780925685, -20.95583473709189093, 37.95507249208304046 ) ) ;
#3622=CARTESIAN_POINT ( 'NONE',  ( -22.04416526290807710, -25.71081734191525925, 23.73242750791695954 ) ) ;
#3627=CARTESIAN_POINT ( 'NONE',  ( -17.95583473709191580, -23.03132541760400898, 24.16992750791696309 ) ) ;
#3644=CARTESIAN_POINT ( 'NONE',  ( -14.83517299489739649, -18.99999999999997868, 35.76367750791695954 ) ) ;
#3649=CARTESIAN_POINT ( 'NONE',  ( -9.999999999999994671, -23.83517299489734143, 28.54882249208304401 ) ) ;
#3653=CARTESIAN_POINT ( 'NONE',  ( -16.64274437364858272, -21.48433729119797420, 32.04882249208304756 ) ) ;
#3669=CARTESIAN_POINT ( 'NONE',  ( -17.64274437364855430, -28.24771351637087236, 33.57617750791696665 ) ) ;
#3671=CARTESIAN_POINT ( 'NONE',  ( -18.53959229564982536, -27.78091578003890660, 35.76757249208302625 ) ) ;
#3674=CARTESIAN_POINT ( 'NONE',  ( -17.35725562635144215, -19.58745947852648683, 14.32617750791695777 ) ) ;
#3676=CARTESIAN_POINT ( 'NONE',  ( -11.21908421996108984, -20.46040770435011069, 31.16992750791695599 ) ) ;
#3678=CARTESIAN_POINT ( 'NONE',  ( -9.999999999999994671, -23.83517299489734143, 28.54882249208304401 ) ) ;
#3687=CARTESIAN_POINT ( 'NONE',  ( -13.28918265808478694, -16.95583473709189093, 37.95507249208304046 ) ) ;
#3689=CARTESIAN_POINT ( 'NONE',  ( -18.04416526290808420, -24.63902057219074493, 23.73242750791696665 ) ) ;
#3692=CARTESIAN_POINT ( 'NONE',  ( -7.955834737091903364, -25.71081734191518464, 23.51757249208304401 ) ) ;
#3706=CARTESIAN_POINT ( 'NONE',  ( -20.00369391078762860, -18.75498260482333279, 29.85742750791695599 ) ) ;
#3711=CARTESIAN_POINT ( 'NONE',  ( -13.64274437364857739, -21.31951028609534760, 32.92382249208304046 ) ) ;
#3712=CARTESIAN_POINT ( 'NONE',  ( -8.044165262908075320, -26.04047135212042718, 16.29492750791696309 ) ) ;
#3718=CARTESIAN_POINT ( 'NONE',  ( -12.04416526290807887, -24.96867458239596260, 32.04492750791695954 ) ) ;
#3736=CARTESIAN_POINT ( 'NONE',  ( -19.41254052147348830, -26.35725562635142083, 34.01367750791696665 ) ) ;
#3740=CARTESIAN_POINT ( 'NONE',  ( -19.95583473709190514, -25.50457296725822687, 30.95507249208303691 ) ) ;
#3744=CARTESIAN_POINT ( 'NONE',  ( -17.99999999999999645, -24.16482700510260173, 25.92382249208304756 ) ) ;
#3764=CARTESIAN_POINT ( 'NONE',  ( -13.49542703274178379, -19.04416526290806289, 25.48242750791694888 ) ) ;
#3767=CARTESIAN_POINT ( 'NONE',  ( -15.16482700510263371, -18.99999999999997868, 37.73632249208303335 ) ) ;
#3770=CARTESIAN_POINT ( 'NONE',  ( -9.999999999999994671, -24.16482700510257686, 26.57617750791695954 ) ) ;
#3772=CARTESIAN_POINT ( 'NONE',  ( -18.53959229564986799, -20.21908421996107563, 29.85742750791695599 ) ) ;
#3775=CARTESIAN_POINT ( 'NONE',  ( -13.82508104294702100, -18.95583473709188382, 22.20507249208304401 ) ) ;
#3790=CARTESIAN_POINT ( 'NONE',  ( -13.64274437364856141, -26.68048971390460622, 27.45117750791696309 ) ) ;
#3792=CARTESIAN_POINT ( 'NONE',  ( -7.999999999999996447, -23.83517299489733432, 39.04882249208302625 ) ) ;
#3807=CARTESIAN_POINT ( 'NONE',  ( -15.16482700510258574, -30.99999999999998224, 27.88867750791695954 ) ) ;
#3812=CARTESIAN_POINT ( 'NONE',  ( -15.96867458239599635, -21.04416526290806999, 27.01757249208303691 ) ) ;
#3813=CARTESIAN_POINT ( 'NONE',  ( -22.04416526290807710, -25.71081734191525925, 28.98242750791695599 ) ) ;
#3834=CARTESIAN_POINT ( 'NONE',  ( -14.83517299489739649, -18.99999999999997868, 30.51367750791695954 ) ) ;
#3838=CARTESIAN_POINT ( 'NONE',  ( -19.41254052147350961, -21.64274437364857562, 31.61132249208303691 ) ) ;
#3840=CARTESIAN_POINT ( 'NONE',  ( -17.99999999999999645, -24.16482700510260173, 31.17382249208304046 ) ) ;
#3858=CARTESIAN_POINT ( 'NONE',  ( -11.46040770435012668, -27.78091578003887463, 27.23242750791694888 ) ) ;
#3860=CARTESIAN_POINT ( 'NONE',  ( -12.35725562635140307, -28.24771351637085459, 39.92382249208304046 ) ) ;
#3862=CARTESIAN_POINT ( 'NONE',  ( -17.64274437364855430, -28.24771351637087236, 33.57617750791696665 ) ) ;
#3864=CARTESIAN_POINT ( 'NONE',  ( -10.58745947852649927, -21.64274437364853654, 31.38867750791696309 ) ) ;
#3866=CARTESIAN_POINT ( 'NONE',  ( -19.95583473709190514, -25.50457296725823042, 20.45507249208304046 ) ) ;
#3876=CARTESIAN_POINT ( 'NONE',  ( -17.64274437364855430, -28.24771351637087236, 2.076177507916958209 ) ) ;
#3879=CARTESIAN_POINT ( 'NONE',  ( -20.24501739517669563, -18.99630608921239627, 31.83007249208304046 ) ) ;
#3894=EDGE_CURVE ( 'NONE', #15887, #1158, #16294, .T. ) ;
#3895=CARTESIAN_POINT ( 'NONE',  ( -9.020235676060220698, -27.64274437364852588, 37.51367750791695244 ) ) ;
#3900=CARTESIAN_POINT ( 'NONE',  ( -12.92450931948788906, -26.31681416490114245, 6.232427507916960430 ) ) ;
#3901=CARTESIAN_POINT ( 'NONE',  ( -9.754982604823348780, -18.99630608921234654, 25.91992750791695599 ) ) ;
#3924=CARTESIAN_POINT ( 'NONE',  ( -21.14459132904236327, -27.35725562635143149, 7.763677507916957765 ) ) ;
#3927=CARTESIAN_POINT ( 'NONE',  ( -16.50457296725825174, -19.04416526290807354, 27.01757249208304046 ) ) ;
#3930=CARTESIAN_POINT ( 'NONE',  ( -12.92450931948790149, -21.68318583509881137, 38.39257249208304756 ) ) ;
#3942=CARTESIAN_POINT ( 'NONE',  ( -11.21908421996108629, -20.46040770435011069, 20.66992750791695244 ) ) ;
#3952=CARTESIAN_POINT ( 'NONE',  ( -19.24771351637089367, -21.35725562635142438, 34.88867750791696665 ) ) ;
#3954=CARTESIAN_POINT ( 'NONE',  ( -19.99999999999999645, -24.16482700510261949, 31.17382249208304046 ) ) ;
#3957=CARTESIAN_POINT ( 'NONE',  ( -17.35725562635144215, -19.58745947852648683, 24.82617750791695954 ) ) ;
#3961=CARTESIAN_POINT ( 'NONE',  ( -12.64274437364855252, -28.41254052147347053, 32.70117750791696665 ) ) ;
#3963=CARTESIAN_POINT ( 'NONE',  ( -20.04416526290809131, -22.82508104294700502, 36.64257249208304046 ) ) ;
#3976=CARTESIAN_POINT ( 'NONE',  ( -12.48433729119798130, -25.64274437364855075, 37.51367750791695954 ) ) ;
#3978=CARTESIAN_POINT ( 'NONE',  ( -14.83517299489734853, -30.99999999999998224, 29.86132249208304046 ) ) ;
#3992=CARTESIAN_POINT ( 'NONE',  ( -14.83517299489734853, -30.99999999999998224, 3.611322492083039570 ) ) ;
#3997=CARTESIAN_POINT ( 'NONE',  ( -16.64274437364856496, -26.51566270880199738, 2.076177507916959986 ) ) ;
#3998=CARTESIAN_POINT ( 'NONE',  ( -18.64274437364853654, -29.97976432393976509, 28.32617750791695954 ) ) ;
#4017=CARTESIAN_POINT ( 'NONE',  ( -18.53959229564986799, -20.21908421996107563, 40.35742750791696665 ) ) ;
#4021=CARTESIAN_POINT ( 'NONE',  ( -16.35725562635141372, -26.68048971390461332, 9.298822492083044011 ) ) ;
#4024=CARTESIAN_POINT ( 'NONE',  ( -12.04416526290808420, -23.03132541760398766, 38.83007249208304756 ) ) ;
#4035=CARTESIAN_POINT ( 'NONE',  ( -13.49542703274178379, -19.04416526290806289, 30.73242750791695599 ) ) ;
#4038=CARTESIAN_POINT ( 'NONE',  ( -16.50457296725820555, -28.95583473709189448, 1.857427507916957765 ) ) ;
#4042=CARTESIAN_POINT ( 'NONE',  ( -12.35725562635140307, -28.24771351637085459, 8.423822492083042235 ) ) ;
#4043=CARTESIAN_POINT ( 'NONE',  ( -21.95583473709191580, -21.95952864787954084, 8.419927507916955989 ) ) ;
#4046=CARTESIAN_POINT ( 'NONE',  ( -11.21908421996106320, -27.53959229564982181, 34.45507249208304046 ) ) ;
#4050=CARTESIAN_POINT ( 'NONE',  ( -13.82508104294698192, -29.04416526290806644, 27.66992750791695244 ) ) ;
#4056=CARTESIAN_POINT ( 'NONE',  ( -14.83517299489735741, -28.99999999999998224, 35.11132249208304046 ) ) ;
#4068=CARTESIAN_POINT ( 'NONE',  ( -13.82508104294698192, -29.04416526290806644, 1.419927507916958209 ) ) ;
#4070=CARTESIAN_POINT ( 'NONE',  ( -7.999999999999996447, -23.83517299489733432, 28.54882249208303691 ) ) ;
#4074=CARTESIAN_POINT ( 'NONE',  ( -16.64274437364856496, -26.51566270880199738, 33.57617750791696665 ) ) ;
#4075=CARTESIAN_POINT ( 'NONE',  ( -19.99999999999999645, -23.83517299489738051, 8.201177507916957765 ) ) ;
#4090=CARTESIAN_POINT ( 'NONE',  ( -20.00369391078757886, -29.24501739517668142, 9.517572492083038682 ) ) ;
#4097=CARTESIAN_POINT ( 'NONE',  ( -15.16482700510260706, -26.99999999999998579, 6.888677507916960430 ) ) ;
#4098=CARTESIAN_POINT ( 'NONE',  ( -21.99999999999999289, -23.83517299489739116, 34.45117750791695954 ) ) ;
#4123=CARTESIAN_POINT ( 'NONE',  ( -12.95952864787955150, -17.04416526290805933, -0.7675724920830436782 ) ) ;
#4128=CARTESIAN_POINT ( 'NONE',  ( -20.04416526290809131, -22.82508104294699791, 41.89257249208301914 ) ) ;
#4134=CARTESIAN_POINT ( 'NONE',  ( -17.99999999999999645, -24.16482700510260173, 41.67382249208304756 ) ) ;
#4146=CARTESIAN_POINT ( 'NONE',  ( -11.46040770435012668, -27.78091578003887463, 21.98242750791695244 ) ) ;
#4148=CARTESIAN_POINT ( 'NONE',  ( -9.999999999999994671, -24.16482700510257686, 5.576177507916958653 ) ) ;
#4153=CARTESIAN_POINT ( 'NONE',  ( -20.04416526290809131, -22.82508104294699791, 10.39257249208304223 ) ) ;
#4154=CARTESIAN_POINT ( 'NONE',  ( -20.00369391078762860, -18.75498260482333279, 3.607427507916956433 ) ) ;
#4156=CARTESIAN_POINT ( 'NONE',  ( -14.83517299489736985, -26.99999999999998579, 3.611322492083043123 ) ) ;
#4160=CARTESIAN_POINT ( 'NONE',  ( -10.58745947852649927, -21.64274437364853654, 36.63867750791695954 ) ) ;
#4164=CARTESIAN_POINT ( 'NONE',  ( -10.04416526290808598, -22.49542703274172695, 38.83007249208303335 ) ) ;
#4174=CARTESIAN_POINT ( 'NONE',  ( -14.83517299489739649, -18.99999999999997868, -0.9863224920830417908 ) ) ;
#4175=CARTESIAN_POINT ( 'NONE',  ( -12.35725562635143682, -19.75228648362908501, -0.5488224920830419018 ) ) ;
#4177=CARTESIAN_POINT ( 'NONE',  ( -17.35725562635140307, -28.41254052147349185, 9.298822492083040459 ) ) ;
#4179=CARTESIAN_POINT ( 'NONE',  ( -14.03132541760401786, -21.04416526290806289, 35.98242750791695954 ) ) ;
#4180=CARTESIAN_POINT ( 'NONE',  ( -17.64274437364855430, -28.24771351637087236, 2.076177507916958209 ) ) ;
#4190=CARTESIAN_POINT ( 'NONE',  ( -9.754982604823302594, -29.00369391078756465, 2.955072492083039126 ) ) ;
#4195=CARTESIAN_POINT ( 'NONE',  ( -12.31951028609537602, -22.64274437364854364, -0.1113224920830400977 ) ) ;
#4196=CARTESIAN_POINT ( 'NONE',  ( -9.020235676060220698, -27.64274437364852588, 37.51367750791695244 ) ) ;
#4216=CARTESIAN_POINT ( 'NONE',  ( -8.044165262908075320, -26.04047135212042718, 5.794927507916956877 ) ) ;
#4221=CARTESIAN_POINT ( 'NONE',  ( -16.17491895705296656, -29.04416526290807710, 40.58007249208304046 ) ) ;
#4225=CARTESIAN_POINT ( 'NONE',  ( -17.51566270880199738, -25.64274437364856496, 41.23632249208304756 ) ) ;
#4237=CARTESIAN_POINT ( 'NONE',  ( -19.95583473709191580, -22.49542703274176603, 24.16992750791694888 ) ) ;
#4241=CARTESIAN_POINT ( 'NONE',  ( -19.41254052147348830, -26.35725562635142083, 2.513677507916958209 ) ) ;
#4244=CARTESIAN_POINT ( 'NONE',  ( -12.35725562635140307, -28.24771351637085459, 3.173822492083041347 ) ) ;
#4246=CARTESIAN_POINT ( 'NONE',  ( -13.28918265808472299, -31.04416526290805933, 1.419927507916956433 ) ) ;
#4249=CARTESIAN_POINT ( 'NONE',  ( -19.24771351637086880, -26.64274437364857206, 41.23632249208304046 ) ) ;
#4253=CARTESIAN_POINT ( 'NONE',  ( -12.64274437364855252, -28.41254052147347053, 37.95117750791695954 ) ) ;
#4257=CARTESIAN_POINT ( 'NONE',  ( -11.46040770435015332, -20.21908421996104011, 38.39257249208303335 ) ) ;
#4264=( NAMED_UNIT ( * ) PLANE_ANGLE_UNIT ( ) SI_UNIT ( $, .RADIAN. ) );
#4269=CARTESIAN_POINT ( 'NONE',  ( -18.53959229564986799, -20.21908421996107563, 8.857427507916957765 ) ) ;
#4270=CARTESIAN_POINT ( 'NONE',  ( -17.99999999999999645, -23.83517299489736985, 39.70117750791695954 ) ) ;
#4272=CARTESIAN_POINT ( 'NONE',  ( -21.95583473709189803, -26.04047135212049469, 41.45507249208303335 ) ) ;
#4276=CARTESIAN_POINT ( 'NONE',  ( -14.83517299489739649, -18.99999999999997868, 4.263677507916958653 ) ) ;
#4277=CARTESIAN_POINT ( 'NONE',  ( -10.31147837279037738, -22.25502639194775512, -4.119453415160654225E-17 ) ) ;
#4291=CARTESIAN_POINT ( 'NONE',  ( -13.28918265808478694, -16.95583473709189093, 1.205072492083039126 ) ) ;
#4292=CARTESIAN_POINT ( 'NONE',  ( -16.17491895705296656, -29.04416526290807354, 3.830072492083040903 ) ) ;
#4295=CARTESIAN_POINT ( 'NONE',  ( -15.63902057219076269, -20.95583473709189448, 4.044927507916962206 ) ) ;
#4296=CARTESIAN_POINT ( 'NONE',  ( -8.855408670957602979, -27.35725562635137820, 7.986322492083039570 ) ) ;
#4315=CARTESIAN_POINT ( 'NONE',  ( -11.64274437364854187, -30.14459132904234195, 6.451177507916957765 ) ) ;
#4319=CARTESIAN_POINT ( 'NONE',  ( -12.68318583509882380, -26.07549068051207541, 2.955072492083043123 ) ) ;
#4323=CARTESIAN_POINT ( 'NONE',  ( -18.04416526290808775, -23.36097942780924441, 41.89257249208304046 ) ) ;
#4336=CARTESIAN_POINT ( 'NONE',  ( -13.49542703274178379, -19.04416526290806289, 20.23242750791696309 ) ) ;
#4342=CARTESIAN_POINT ( 'NONE',  ( -17.35725562635140307, -28.41254052147349185, 4.048822492083041347 ) ) ;
#4343=CARTESIAN_POINT ( 'NONE',  ( -7.955834737091916686, -22.28918265808470522, 0.1074275079169565300 ) ) ;
#4345=CARTESIAN_POINT ( 'NONE',  ( -14.83517299489735741, -28.99999999999998224, 40.36132249208304046 ) ) ;
#4358=CARTESIAN_POINT ( 'NONE',  ( -19.99999999999999645, -24.16482700510261949, 41.67382249208304046 ) ) ;
#4366=CARTESIAN_POINT ( 'NONE',  ( -11.46040770435012668, -27.78091578003887463, 6.232427507916956877 ) ) ;
#4367=CARTESIAN_POINT ( 'NONE',  ( -13.82508104294698192, -29.04416526290806644, 11.91992750791695421 ) ) ;
#4369=CARTESIAN_POINT ( 'NONE',  ( -11.46040770435014977, -20.21908421996103655, 6.892572492083040459 ) ) ;
#4374=CARTESIAN_POINT ( 'NONE',  ( -15.16482700510259640, -28.99999999999998224, 6.888677507916957765 ) ) ;
#4375=CARTESIAN_POINT ( 'NONE',  ( -9.955834737091912245, -22.82508104294696238, 10.60742750791695777 ) ) ;
#4389=CARTESIAN_POINT ( 'NONE',  ( -9.020235676060250896, -20.35725562635137820, 12.36132249208304046 ) ) ;
#4395=CARTESIAN_POINT ( 'NONE',  ( -16.35725562635142794, -21.31951028609535470, 14.32617750791695777 ) ) ;
#4397=CARTESIAN_POINT ( 'NONE',  ( -9.754982604823302594, -29.00369391078756465, 2.955072492083039126 ) ) ;
#4405=CARTESIAN_POINT ( 'NONE',  ( -10.80184671977677091, -22.03375095468977207, 1.107186296610940968E-15 ) ) ;
#4415=CARTESIAN_POINT ( 'NONE',  ( -7.955834737091916686, -22.28918265808470522, 15.85742750791695954 ) ) ;
#4420=CARTESIAN_POINT ( 'NONE',  ( -11.99999999999999289, -23.83517299489735564, 7.548822492083043123 ) ) ;
#4425=CARTESIAN_POINT ( 'NONE',  ( -17.68048971390461688, -25.35725562635141372, 2.513677507916959986 ) ) ;
#4441=CARTESIAN_POINT ( 'NONE',  ( -9.999999999999994671, -24.16482700510257686, 10.82617750791695777 ) ) ;
#4444=CARTESIAN_POINT ( 'NONE',  ( -11.46040770435014977, -20.21908421996103655, 6.892572492083040459 ) ) ;
#4450=CARTESIAN_POINT ( 'NONE',  ( -16.50457296725825174, -19.04416526290807354, 42.76757249208303335 ) ) ;
#4454=CARTESIAN_POINT ( 'NONE',  ( -15.00000000000001954, -17.99999999999997868, -4.814824860968089633E-32 ) ) ;
#4467=ORIENTED_EDGE ( 'NONE', *, *, #975, .F. ) ;
#4469=CARTESIAN_POINT ( 'NONE',  ( -13.49542703274178379, -19.04416526290806289, 4.482427507916957765 ) ) ;
#4471=CARTESIAN_POINT ( 'NONE',  ( -14.83517299489739649, -18.99999999999997868, 20.01367750791695954 ) ) ;
#4474=CARTESIAN_POINT ( 'NONE',  ( -16.17491895705296656, -29.04416526290807710, 3.830072492083041347 ) ) ;
#4476=CARTESIAN_POINT ( 'NONE',  ( -19.41254052147348830, -26.35725562635142083, 7.763677507916958653 ) ) ;
#4491=CARTESIAN_POINT ( 'NONE',  ( -21.95583473709189803, -26.04047135212049469, 20.45507249208304046 ) ) ;
#4492=CARTESIAN_POINT ( 'NONE',  ( -12.64274437364858628, -19.58745947852646552, 1.423822492083040903 ) ) ;
#4495=CARTESIAN_POINT ( 'NONE',  ( -14.36097942780923731, -27.04416526290806999, 22.41992750791696309 ) ) ;
#4497=CARTESIAN_POINT ( 'NONE',  ( -21.14459132904236327, -27.35725562635143149, 39.26367750791695244 ) ) ;
#4515=CARTESIAN_POINT ( 'NONE',  ( -18.64274437364853654, -29.97976432393976509, 23.07617750791695954 ) ) ;
#4519=CARTESIAN_POINT ( 'NONE',  ( -17.99999999999999645, -24.16482700510260173, 15.42382249208304223 ) ) ;
#4520=STYLED_ITEM ( 'NONE', ( #8956 ), #16836 ) ;
#4524=CARTESIAN_POINT ( 'NONE',  ( -12.31951028609537602, -22.64274437364854364, 10.38867750791695954 ) ) ;
#4536=CARTESIAN_POINT ( 'NONE',  ( -16.17491895705301275, -18.95583473709189803, 35.54492750791695954 ) ) ;
#4539=CARTESIAN_POINT ( 'NONE',  ( -12.64274437364855252, -28.41254052147347053, 22.20117750791695599 ) ) ;
#4541=EDGE_LOOP ( 'NONE', ( #6860, #3144, #17161, #6078, #1448 ) ) ;
#4542=CARTESIAN_POINT ( 'NONE',  ( -11.46040770435014977, -20.21908421996103655, 22.64257249208303335 ) ) ;
#4544=CARTESIAN_POINT ( 'NONE',  ( -18.04416526290808775, -23.36097942780924441, 10.39257249208304223 ) ) ;
#4565=CARTESIAN_POINT ( 'NONE',  ( -16.17491895705301275, -18.95583473709189803, 4.044927507916959541 ) ) ;
#4566=CARTESIAN_POINT ( 'NONE',  ( -10.58745947852649927, -21.64274437364853654, 10.38867750791695777 ) ) ;
#4568=CARTESIAN_POINT ( 'NONE',  ( -19.41254052147350961, -21.64274437364857562, 10.61132249208304046 ) ) ;
#4570=CARTESIAN_POINT ( 'NONE',  ( -17.64274437364855430, -28.24771351637087236, 7.326177507916957765 ) ) ;
#4574=CARTESIAN_POINT ( 'NONE',  ( -19.95583473709191225, -22.49542703274176603, 18.91992750791695599 ) ) ;
#4586=CARTESIAN_POINT ( 'NONE',  ( -9.996306089212408708, -18.75498260482328661, 12.14257249208303691 ) ) ;
#4593=CARTESIAN_POINT ( 'NONE',  ( -11.95583473709191047, -23.36097942780921954, 10.60742750791695954 ) ) ;
#4595=CARTESIAN_POINT ( 'NONE',  ( -18.35725562635138886, -30.14459132904237393, 4.048822492083038682 ) ) ;
#4604=CARTESIAN_POINT ( 'NONE',  ( -14.55051906578255938, -19.99999999999997158, 5.135813185032623395E-31 ) ) ;
#4616=CARTESIAN_POINT ( 'NONE',  ( -12.95952864787955150, -17.04416526290805933, 20.23242750791695954 ) ) ;
#4621=CARTESIAN_POINT ( 'NONE',  ( -18.04416526290808775, -23.36097942780924441, 20.89257249208304046 ) ) ;
#4626=CARTESIAN_POINT ( 'NONE',  ( -13.35725562635142794, -21.48433729119796709, 20.45117750791696309 ) ) ;
#4641=CARTESIAN_POINT ( 'NONE',  ( -20.04416526290808065, -25.17491895705300209, 13.23242750791695777 ) ) ;
#4644=CARTESIAN_POINT ( 'NONE',  ( -17.64274437364858983, -19.75228648362910633, 16.29882249208304046 ) ) ;
#4647=CARTESIAN_POINT ( 'NONE',  ( -17.99999999999999645, -24.16482700510260173, 15.42382249208304223 ) ) ;
#4650=CARTESIAN_POINT ( 'NONE',  ( -12.67132176431211832, -18.52296496192205311, 5.414424919715126740E-14 ) ) ;
#4662=CARTESIAN_POINT ( 'NONE',  ( -15.16482700510259640, -28.99999999999998224, 17.38867750791695599 ) ) ;
#4663=CARTESIAN_POINT ( 'NONE',  ( -10.04416526290807710, -25.50457296725819489, 11.04492750791695421 ) ) ;
#4665=CARTESIAN_POINT ( 'NONE',  ( -16.17491895705296656, -29.04416526290807710, 24.83007249208304046 ) ) ;
#4667=CARTESIAN_POINT ( 'NONE',  ( -19.95583473709191580, -22.49542703274176603, 3.169927507916957321 ) ) ;
#4670=CARTESIAN_POINT ( 'NONE',  ( -14.83517299489739649, -18.99999999999997868, 25.26367750791695599 ) ) ;
#4683=CARTESIAN_POINT ( 'NONE',  ( -20.00369391078757886, -29.24501739517668142, 14.76757249208304046 ) ) ;
#4685=CARTESIAN_POINT ( 'NONE',  ( -11.46040770435015332, -20.21908421996104011, 12.14257249208304046 ) ) ;
#4688=CARTESIAN_POINT ( 'NONE',  ( -13.64274437364856141, -26.68048971390460622, 16.95117750791696309 ) ) ;
#4690=CARTESIAN_POINT ( 'NONE',  ( -16.71081734191520596, -31.04416526290808065, 9.080072492083038682 ) ) ;
#4714=CARTESIAN_POINT ( 'NONE',  ( -7.999999999999996447, -24.16482700510256976, 16.07617750791695599 ) ) ;
#4718=CARTESIAN_POINT ( 'NONE',  ( -17.31681416490117087, -21.92450931948788551, 16.08007249208304401 ) ) ;
#4720=CARTESIAN_POINT ( 'NONE',  ( -18.78091578003889950, -27.53959229564985378, 39.04492750791695954 ) ) ;
#4724=CARTESIAN_POINT ( 'NONE',  ( -17.99999999999999645, -23.83517299489736985, 13.45117750791696309 ) ) ;
#4741=CARTESIAN_POINT ( 'NONE',  ( -18.78091578003889950, -27.53959229564985378, 12.79492750791695421 ) ) ;
#4747=CARTESIAN_POINT ( 'NONE',  ( -13.82508104294702100, -18.95583473709188382, 11.70507249208303868 ) ) ;
#4748=EDGE_CURVE ( 'NONE', #14224, #13312, #235, .T. ) ;
#4752=CARTESIAN_POINT ( 'NONE',  ( -12.04416526290808420, -23.03132541760398766, 17.83007249208304046 ) ) ;
#4773=CARTESIAN_POINT ( 'NONE',  ( -11.46040770435012668, -27.78091578003887463, 16.73242750791695954 ) ) ;
#4775=CARTESIAN_POINT ( 'NONE',  ( -13.49542703274174116, -28.95583473709188738, 19.14257249208304401 ) ) ;
#4777=CARTESIAN_POINT ( 'NONE',  ( -10.04416526290807710, -25.50457296725819489, 21.54492750791695599 ) ) ;
#4779=CARTESIAN_POINT ( 'NONE',  ( -11.21908421996108984, -20.46040770435011069, 15.41992750791695777 ) ) ;
#4792=CARTESIAN_POINT ( 'NONE',  ( -20.24501739517669563, -18.99630608921239627, 31.83007249208304046 ) ) ;
#4794=CARTESIAN_POINT ( 'NONE',  ( -17.64274437364858983, -19.75228648362910633, 16.29882249208304046 ) ) ;
#4796=CARTESIAN_POINT ( 'NONE',  ( -12.04416526290807887, -24.96867458239596260, 16.29492750791696665 ) ) ;
#4798=CARTESIAN_POINT ( 'NONE',  ( -7.955834737091903364, -25.71081734191518464, 13.01757249208304046 ) ) ;
#4814=CARTESIAN_POINT ( 'NONE',  ( -8.044165262908075320, -26.04047135212042718, 16.29492750791696309 ) ) ;
#4815=DIRECTION ( 'NONE',  ( 0.000000000000000000, 0.000000000000000000, 1.000000000000000000 ) ) ;
#4818=CARTESIAN_POINT ( 'NONE',  ( -14.36097942780925685, -20.95583473709189093, 22.20507249208304401 ) ) ;
#4819=CARTESIAN_POINT ( 'NONE',  ( -18.64274437364853654, -29.97976432393976509, 23.07617750791695954 ) ) ;
#4823=CARTESIAN_POINT ( 'NONE',  ( -15.16482700510260706, -26.99999999999998579, 12.13867750791695954 ) ) ;
#4838=CARTESIAN_POINT ( 'NONE',  ( -16.50457296725820555, -28.95583473709189448, 12.35742750791695954 ) ) ;
#4841=CARTESIAN_POINT ( 'NONE',  ( -10.58745947852648328, -26.35725562635138530, 13.23632249208304046 ) ) ;
#4842=CARTESIAN_POINT ( 'NONE',  ( -14.36097942780925685, -20.95583473709189093, 16.95507249208304046 ) ) ;
#4860=CARTESIAN_POINT ( 'NONE',  ( -15.16482700510259640, -28.99999999999998224, 12.13867750791695777 ) ) ;
#4863=CARTESIAN_POINT ( 'NONE',  ( -16.17491895705296656, -29.04416526290807710, 19.58007249208303335 ) ) ;
#4865=CARTESIAN_POINT ( 'NONE',  ( -10.04416526290807710, -25.50457296725819489, 11.04492750791695421 ) ) ;
#4867=CARTESIAN_POINT ( 'NONE',  ( -19.41254052147348830, -26.35725562635142083, 18.26367750791695599 ) ) ;
#4880=CARTESIAN_POINT ( 'NONE',  ( -21.95583473709189803, -26.04047135212049469, 30.95507249208304401 ) ) ;
#4882=CARTESIAN_POINT ( 'NONE',  ( -11.21908421996106142, -27.53959229564982181, 8.205072492083040459 ) ) ;
#4884=CARTESIAN_POINT ( 'NONE',  ( -17.99999999999999645, -23.83517299489736985, 29.20117750791695954 ) ) ;
#4886=CARTESIAN_POINT ( 'NONE',  ( -8.855408670957602979, -27.35725562635137820, 13.23632249208303868 ) ) ;
#4908=CARTESIAN_POINT ( 'NONE',  ( -7.955834737091916686, -22.28918265808470522, 26.35742750791695954 ) ) ;
#4911=CARTESIAN_POINT ( 'NONE',  ( -16.64274437364858272, -21.48433729119797420, 21.54882249208304401 ) ) ;
#4912=CARTESIAN_POINT ( 'NONE',  ( -20.24501739517664234, -29.00369391078761439, 18.04492750791695954 ) ) ;
#4917=CARTESIAN_POINT ( 'NONE',  ( -12.48433729119798130, -25.64274437364855075, 11.26367750791696132 ) ) ;
#4935=CARTESIAN_POINT ( 'NONE',  ( -13.49542703274178379, -19.04416526290806289, 35.98242750791696665 ) ) ;
#4940=CARTESIAN_POINT ( 'NONE',  ( -13.49542703274174116, -28.95583473709188738, 19.14257249208304401 ) ) ;
#4941=CARTESIAN_POINT ( 'NONE',  ( -16.64274437364858272, -21.48433729119797420, 21.54882249208304401 ) ) ;
#4958=CARTESIAN_POINT ( 'NONE',  ( -16.17491895705301275, -18.95583473709189803, 19.79492750791695954 ) ) ;
#4961=CARTESIAN_POINT ( 'NONE',  ( -19.41254052147350961, -21.64274437364857562, 21.11132249208304401 ) ) ;
#4963=CARTESIAN_POINT ( 'NONE',  ( -11.46040770435012668, -27.78091578003887463, 11.48242750791695954 ) ) ;
#4965=CARTESIAN_POINT ( 'NONE',  ( -13.82508104294698015, -29.04416526290806289, 17.16992750791695244 ) ) ;
#4966=CARTESIAN_POINT ( 'NONE',  ( -19.95583473709190514, -25.50457296725823042, 25.70507249208304756 ) ) ;
#4977=CARTESIAN_POINT ( 'NONE',  ( -8.855408670957602979, -27.35725562635137820, 34.23632249208304046 ) ) ;
#4979=CARTESIAN_POINT ( 'NONE',  ( -10.58745947852648328, -26.35725562635138530, 13.23632249208304046 ) ) ;
#4982=CARTESIAN_POINT ( 'NONE',  ( -15.63902057219076269, -20.95583473709189448, 25.04492750791696309 ) ) ;
#4984=CARTESIAN_POINT ( 'NONE',  ( -18.64274437364860049, -18.02023567606023491, 16.29882249208303691 ) ) ;
#5002=CARTESIAN_POINT ( 'NONE',  ( -8.044165262908075320, -26.04047135212042718, 37.29492750791695954 ) ) ;
#5006=CARTESIAN_POINT ( 'NONE',  ( -14.83517299489736985, -26.99999999999998579, 29.86132249208304756 ) ) ;
#5007=CARTESIAN_POINT ( 'NONE',  ( -13.28918265808472299, -31.04416526290805933, 22.41992750791695954 ) ) ;
#5011=CARTESIAN_POINT ( 'NONE',  ( -12.04416526290807887, -24.96867458239596260, 37.29492750791695954 ) ) ;
#5029=CARTESIAN_POINT ( 'NONE',  ( -9.999999999999994671, -24.16482700510257686, 31.82617750791696309 ) ) ;
#5033=CARTESIAN_POINT ( 'NONE',  ( -18.78091578003892081, -20.46040770435013556, 37.08007249208304046 ) ) ;
#5035=CARTESIAN_POINT ( 'NONE',  ( -16.64274437364858272, -21.48433729119797420, 16.29882249208304401 ) ) ;
#5054=CARTESIAN_POINT ( 'NONE',  ( -12.35725562635143682, -19.75228648362908501, 15.20117750791695777 ) ) ;
#5057=CARTESIAN_POINT ( 'NONE',  ( -20.04416526290809131, -22.82508104294699791, 15.64257249208304223 ) ) ;
#5060=CARTESIAN_POINT ( 'NONE',  ( -14.83517299489739649, -18.99999999999997868, 14.76367750791695777 ) ) ;
#5064=CARTESIAN_POINT ( 'NONE',  ( -19.99999999999999645, -23.83517299489738051, 29.20117750791695599 ) ) ;
#5066=CARTESIAN_POINT ( 'NONE',  ( -18.53959229564983247, -27.78091578003891016, 30.51757249208304401 ) ) ;
#5076=CARTESIAN_POINT ( 'NONE',  ( -21.99999999999999289, -24.16482700510262305, 36.42382249208304756 ) ) ;
#5078=CARTESIAN_POINT ( 'NONE',  ( -13.82508104294702100, -18.95583473709188382, 16.95507249208304401 ) ) ;
#5080=CARTESIAN_POINT ( 'NONE',  ( -12.48433729119798130, -25.64274437364855075, 32.26367750791695954 ) ) ;
#5083=CARTESIAN_POINT ( 'NONE',  ( -12.95952864787948755, -30.95583473709188382, 13.89257249208304046 ) ) ;
#5102=CARTESIAN_POINT ( 'NONE',  ( -20.24501739517664234, -29.00369391078761439, 28.54492750791695954 ) ) ;
#5106=CARTESIAN_POINT ( 'NONE',  ( -15.96867458239599635, -21.04416526290806999, 32.26757249208305467 ) ) ;
#5107=CARTESIAN_POINT ( 'NONE',  ( -21.95583473709191580, -21.95952864787954084, 24.16992750791695954 ) ) ;
#5113=CARTESIAN_POINT ( 'NONE',  ( -17.31681416490115311, -26.07549068051209318, 28.54492750791696665 ) ) ;
#5131=CARTESIAN_POINT ( 'NONE',  ( -12.35725562635143682, -19.75228648362908501, 25.70117750791695599 ) ) ;
#5134=CARTESIAN_POINT ( 'NONE',  ( -9.955834737091903364, -25.17491895705294880, 28.76757249208304401 ) ) ;
#5135=CARTESIAN_POINT ( 'NONE',  ( -12.04416526290808420, -23.03132541760398766, 28.33007249208304756 ) ) ;
#5147=CARTESIAN_POINT ( 'NONE',  ( -12.64274437364855252, -28.41254052147347053, 27.45117750791695954 ) ) ;
#5149=CARTESIAN_POINT ( 'NONE',  ( -19.41254052147350961, -21.64274437364857562, 31.61132249208303691 ) ) ;
#5152=CARTESIAN_POINT ( 'NONE',  ( -9.999999999999994671, -24.16482700510257686, 10.82617750791695777 ) ) ;
#5154=CARTESIAN_POINT ( 'NONE',  ( -9.999999999999994671, -24.16482700510257686, 37.07617750791695954 ) ) ;
#5156=CARTESIAN_POINT ( 'NONE',  ( -19.99999999999999645, -24.16482700510261949, 25.92382249208304401 ) ) ;
#5166=CARTESIAN_POINT ( 'NONE',  ( -18.64274437364860049, -18.02023567606023491, 37.29882249208304046 ) ) ;
#5168=CARTESIAN_POINT ( 'NONE',  ( -12.68318583509884157, -21.92450931948787485, 31.16992750791695954 ) ) ;
#5170=CARTESIAN_POINT ( 'NONE',  ( -18.35725562635138886, -30.14459132904237393, 19.79882249208303691 ) ) ;
#5187=CARTESIAN_POINT ( 'NONE',  ( -11.35725562635144925, -18.02023567606020293, 36.20117750791695244 ) ) ;
#5192=ORIENTED_EDGE ( 'NONE', *, *, #12749, .T. ) ;
#5194=CARTESIAN_POINT ( 'NONE',  ( -14.36097942780925685, -20.95583473709189093, 32.70507249208304756 ) ) ;
#5195=CARTESIAN_POINT ( 'NONE',  ( -21.99999999999999289, -23.83517299489739116, 13.45117750791695777 ) ) ;
#5202=CARTESIAN_POINT ( 'NONE',  ( -12.04416526290807887, -24.96867458239596260, 26.79492750791695954 ) ) ;
#5220=CARTESIAN_POINT ( 'NONE',  ( -9.999999999999994671, -24.16482700510257686, 26.57617750791695954 ) ) ;
#5223=CARTESIAN_POINT ( 'NONE',  ( -10.58745947852648328, -26.35725562635138530, 28.98632249208304401 ) ) ;
#5228=CARTESIAN_POINT ( 'NONE',  ( -11.99999999999999289, -23.83517299489735564, 28.54882249208304046 ) ) ;
#5244=CARTESIAN_POINT ( 'NONE',  ( -19.99999999999999645, -23.83517299489738051, 34.45117750791696665 ) ) ;
#5246=CARTESIAN_POINT ( 'NONE',  ( -19.24771351637086880, -26.64274437364857206, 30.73632249208304401 ) ) ;
#5249=CARTESIAN_POINT ( 'NONE',  ( -12.64274437364855252, -28.41254052147347053, 27.45117750791695954 ) ) ;
#5251=CARTESIAN_POINT ( 'NONE',  ( -18.78091578003889595, -27.53959229564985023, 28.54492750791695954 ) ) ;
#5253=CARTESIAN_POINT ( 'NONE',  ( -13.49542703274174116, -28.95583473709188738, 29.64257249208304046 ) ) ;
#5261=CARTESIAN_POINT ( 'NONE',  ( -13.64274437364856141, -26.68048971390460622, 32.70117750791696665 ) ) ;
#5263=CARTESIAN_POINT ( 'NONE',  ( -11.35725562635139418, -29.97976432393972601, 34.67382249208304046 ) ) ;
#5275=CARTESIAN_POINT ( 'NONE',  ( -9.020235676060220698, -27.64274437364852588, 27.01367750791695599 ) ) ;
#5279=CARTESIAN_POINT ( 'NONE',  ( -17.95583473709190869, -24.96867458239598037, 25.70507249208304756 ) ) ;
#5282=CARTESIAN_POINT ( 'NONE',  ( -20.00369391078762860, -18.75498260482333279, 29.85742750791695599 ) ) ;
#5287=CARTESIAN_POINT ( 'NONE',  ( -14.83517299489738761, -20.99999999999997513, 30.51367750791696309 ) ) ;
#5306=CARTESIAN_POINT ( 'NONE',  ( -18.53959229564986799, -20.21908421996107563, 29.85742750791695599 ) ) ;
#5309=CARTESIAN_POINT ( 'NONE',  ( -11.21908421996106320, -27.53959229564982181, 34.45507249208304046 ) ) ;
#5312=CARTESIAN_POINT ( 'NONE',  ( -17.68048971390462754, -22.64274437364856496, 26.36132249208304401 ) ) ;
#5333=EDGE_CURVE ( 'NONE', #1158, #14224, #18089, .T. ) ;
#5334=CARTESIAN_POINT ( 'NONE',  ( -12.35725562635143682, -19.75228648362908501, 25.70117750791695599 ) ) ;
#5337=CARTESIAN_POINT ( 'NONE',  ( -10.58745947852648328, -26.35725562635138530, 39.48632249208304046 ) ) ;
#5339=CARTESIAN_POINT ( 'NONE',  ( -17.35725562635144215, -19.58745947852648683, 30.07617750791695599 ) ) ;
#5341=CARTESIAN_POINT ( 'NONE',  ( -18.78091578003889595, -27.53959229564985023, 39.04492750791695954 ) ) ;
#5344=CARTESIAN_POINT ( 'NONE',  ( -19.24771351637086880, -26.64274437364857206, 20.23632249208304046 ) ) ;
#5359=CARTESIAN_POINT ( 'NONE',  ( -11.21908421996108629, -20.46040770435011069, 4.919927507916955989 ) ) ;
#5361=CARTESIAN_POINT ( 'NONE',  ( -15.16482700510264436, -16.99999999999997868, 27.23632249208303691 ) ) ;
#5378=CARTESIAN_POINT ( 'NONE',  ( -14.83517299489740715, -16.99999999999997868, 41.01367750791695954 ) ) ;
#5383=CARTESIAN_POINT ( 'NONE',  ( -12.31951028609537602, -22.64274437364854364, 5.138677507916959541 ) ) ;
#5384=CARTESIAN_POINT ( 'NONE',  ( -16.71081734191527346, -16.95583473709190159, 25.04492750791695599 ) ) ;
#5405=CARTESIAN_POINT ( 'NONE',  ( -21.99999999999999289, -23.83517299489739116, 2.951177507916956433 ) ) ;
#5408=CARTESIAN_POINT ( 'NONE',  ( -13.49542703274174116, -28.95583473709188738, 34.89257249208304046 ) ) ;
#5412=CARTESIAN_POINT ( 'NONE',  ( -12.68318583509882380, -26.07549068051207541, 29.20507249208304756 ) ) ;
#5421=CARTESIAN_POINT ( 'NONE',  ( -20.04416526290808065, -25.17491895705300209, 23.73242750791694888 ) ) ;
#5427=CARTESIAN_POINT ( 'NONE',  ( -18.78091578003889950, -27.53959229564985378, 28.54492750791695954 ) ) ;
#5429=CARTESIAN_POINT ( 'NONE',  ( -14.83517299489735741, -28.99999999999998224, 35.11132249208304046 ) ) ;
#5434=CARTESIAN_POINT ( 'NONE',  ( -18.53959229564986799, -20.21908421996107563, 35.10742750791694533 ) ) ;
#5437=CARTESIAN_POINT ( 'NONE',  ( -11.46040770435012490, -27.78091578003888173, 32.48242750791695954 ) ) ;
#5448=CARTESIAN_POINT ( 'NONE',  ( -12.31951028609537602, -22.64274437364854364, 36.63867750791695244 ) ) ;
#5450=CARTESIAN_POINT ( 'NONE',  ( -14.83517299489734853, -30.99999999999998224, 35.11132249208304046 ) ) ;
#5463=CARTESIAN_POINT ( 'NONE',  ( -9.996306089212408708, -18.75498260482328661, 1.642572492083039126 ) ) ;
#5468=CARTESIAN_POINT ( 'NONE',  ( -15.96867458239597326, -26.95583473709190159, 1.857427507916959986 ) ) ;
#5469=CARTESIAN_POINT ( 'NONE',  ( -21.14459132904236327, -27.35725562635143149, 34.01367750791695244 ) ) ;
#5492=CARTESIAN_POINT ( 'NONE',  ( -20.00369391078762860, -18.75498260482333279, 8.857427507916955989 ) ) ;
#5495=CARTESIAN_POINT ( 'NONE',  ( -12.31951028609536536, -25.35725562635139596, 2.736322492083043123 ) ) ;
#5498=CARTESIAN_POINT ( 'NONE',  ( -14.83517299489736985, -26.99999999999998579, 35.11132249208304756 ) ) ;
#5508=CARTESIAN_POINT ( 'NONE',  ( -10.04416526290807710, -25.50457296725819489, 26.79492750791695954 ) ) ;
#5511=CARTESIAN_POINT ( 'NONE',  ( -10.58745947852649927, -21.64274437364853654, -0.1113224920830418047 ) ) ;
#5516=UNCERTAINTY_MEASURE_WITH_UNIT (LENGTH_MEASURE( 1.000000000000000082E-05 ), #2713, 'distance_accuracy_value', 'NONE');
#5517=CARTESIAN_POINT ( 'NONE',  ( -12.95952864787948755, -30.95583473709188382, 40.14257249208304756 ) ) ;
#5518=CARTESIAN_POINT ( 'NONE',  ( -19.41254052147348830, -26.35725562635142083, 34.01367750791696665 ) ) ;
#5522=CARTESIAN_POINT ( 'NONE',  ( -18.78091578003892081, -20.46040770435013556, 26.58007249208304401 ) ) ;
#5526=CARTESIAN_POINT ( 'NONE',  ( -18.78091578003889950, -27.53959229564985378, 28.54492750791695954 ) ) ;
#5532=CARTESIAN_POINT ( 'NONE',  ( -10.58745947852648328, -26.35725562635138530, 34.23632249208304046 ) ) ;
#5545=CARTESIAN_POINT ( 'NONE',  ( -13.82508104294698192, -29.04416526290806644, 6.669927507916955989 ) ) ;
#5547=CARTESIAN_POINT ( 'NONE',  ( -20.24501739517669563, -18.99630608921239627, 26.58007249208304046 ) ) ;
#5560=CARTESIAN_POINT ( 'NONE',  ( -14.83517299489734853, -30.99999999999998224, 8.861322492083038682 ) ) ;
#5565=CARTESIAN_POINT ( 'NONE',  ( -15.96867458239599635, -21.04416526290806999, 42.76757249208304756 ) ) ;
#5567=CARTESIAN_POINT ( 'NONE',  ( -18.64274437364853654, -29.97976432393976509, 33.57617750791695954 ) ) ;
#5587=CARTESIAN_POINT ( 'NONE',  ( -19.41254052147348830, -26.35725562635142083, 39.26367750791695954 ) ) ;
#5591=CARTESIAN_POINT ( 'NONE',  ( -17.68048971390462754, -22.64274437364856496, 10.61132249208304401 ) ) ;
#5594=CARTESIAN_POINT ( 'NONE',  ( -15.63902057219073605, -27.04416526290807710, 40.58007249208304756 ) ) ;
#5608=CARTESIAN_POINT ( 'NONE',  ( -17.35725562635144215, -19.58745947852648683, 30.07617750791695599 ) ) ;
#5610=CARTESIAN_POINT ( 'NONE',  ( -19.99999999999999645, -23.83517299489738051, 2.951177507916958209 ) ) ;
#5614=CARTESIAN_POINT ( 'NONE',  ( -19.24771351637086880, -26.64274437364857206, 9.736322492083042235 ) ) ;
#5616=CARTESIAN_POINT ( 'NONE',  ( -11.64274437364854187, -30.14459132904234195, 1.201177507916956433 ) ) ;
#5619=CARTESIAN_POINT ( 'NONE',  ( -17.51566270880199738, -25.64274437364856496, 4.486322492083042235 ) ) ;
#5623=CARTESIAN_POINT ( 'NONE',  ( -16.17491895705301275, -18.95583473709189803, 30.29492750791695244 ) ) ;
#5627=DIRECTION ( 'NONE',  ( 0.1648270051026190508, 0.000000000000000000, -0.9863224920830413467 ) ) ;
#5628=CARTESIAN_POINT ( 'NONE',  ( -10.75228648362912232, -21.35725562635138530, 33.36132249208304046 ) ) ;
#5638=CARTESIAN_POINT ( 'NONE',  ( -20.04416526290808065, -25.17491895705300209, 7.982427507916958653 ) ) ;
#5640=CARTESIAN_POINT ( 'NONE',  ( -19.41254052147348830, -26.35725562635142083, 7.763677507916958653 ) ) ;
#5643=CARTESIAN_POINT ( 'NONE',  ( -15.16482700510264436, -16.99999999999997868, 32.48632249208304046 ) ) ;
#5646=CARTESIAN_POINT ( 'NONE',  ( -15.16482700510260706, -26.99999999999998579, 33.13867750791695954 ) ) ;
#5659=CARTESIAN_POINT ( 'NONE',  ( -18.35725562635138886, -30.14459132904237393, 9.298822492083038682 ) ) ;
#5664=CARTESIAN_POINT ( 'NONE',  ( -12.31951028609536536, -25.35725562635139596, 39.48632249208304756 ) ) ;
#5665=CARTESIAN_POINT ( 'NONE',  ( -7.999999999999996447, -24.16482700510256976, 37.07617750791694533 ) ) ;
#5690=CARTESIAN_POINT ( 'NONE',  ( -16.17491895705301275, -18.95583473709189803, 40.79492750791695954 ) ) ;
#5695=CARTESIAN_POINT ( 'NONE',  ( -16.35725562635141372, -26.68048971390461332, 4.048822492083043123 ) ) ;
#5701=CARTESIAN_POINT ( 'NONE',  ( -13.64274437364856141, -26.68048971390460622, 1.201177507916959986 ) ) ;
#5712=CARTESIAN_POINT ( 'NONE',  ( -15.16482700510259640, -28.99999999999998224, 27.88867750791695954 ) ) ;
#5717=CARTESIAN_POINT ( 'NONE',  ( -20.97976432393974022, -27.64274437364858628, 41.23632249208304046 ) ) ;
#5718=CARTESIAN_POINT ( 'NONE',  ( -9.996306089212364299, -29.24501739517662813, 6.232427507916955989 ) ) ;
#5721=CARTESIAN_POINT ( 'NONE',  ( -14.36097942780925685, -20.95583473709189093, 1.205072492083042901 ) ) ;
#5725=CARTESIAN_POINT ( 'NONE',  ( -14.83517299489739649, -18.99999999999997868, 41.01367750791696665 ) ) ;
#5729=CARTESIAN_POINT ( 'NONE',  ( -16.17491895705296656, -29.04416526290807354, 35.33007249208303335 ) ) ;
#5738=CARTESIAN_POINT ( 'NONE',  ( -19.95583473709191580, -22.49542703274176603, 8.419927507916955989 ) ) ;
#5739=CARTESIAN_POINT ( 'NONE',  ( -15.96867458239597326, -26.95583473709190159, 38.60742750791696665 ) ) ;
#5741=CARTESIAN_POINT ( 'NONE',  ( -12.64274437364858628, -19.58745947852646552, 1.423822492083040903 ) ) ;
#5743=CARTESIAN_POINT ( 'NONE',  ( -9.955834737091912245, -22.82508104294696594, 5.357427507916956877 ) ) ;
#5744=CARTESIAN_POINT ( 'NONE',  ( -19.95583473709191225, -22.49542703274176603, 8.419927507916954212 ) ) ;
#5754=CARTESIAN_POINT ( 'NONE',  ( -18.64274437364860049, -18.02023567606023491, 11.04882249208303868 ) ) ;
#5756=CARTESIAN_POINT ( 'NONE',  ( -13.49542703274174116, -28.95583473709188738, 3.392572492083040903 ) ) ;
#5759=CARTESIAN_POINT ( 'NONE',  ( -15.16482700510262482, -20.99999999999997513, 42.98632249208304756 ) ) ;
#5760=CARTESIAN_POINT ( 'NONE',  ( -11.35725562635139418, -29.97976432393972601, 8.423822492083040459 ) ) ;
#5781=CARTESIAN_POINT ( 'NONE',  ( -9.754982604823348780, -18.99630608921234654, -0.3300724920830435116 ) ) ;
#5787=CARTESIAN_POINT ( 'NONE',  ( -14.36097942780925685, -20.95583473709189093, 1.205072492083042901 ) ) ;
#5792=CARTESIAN_POINT ( 'NONE',  ( -14.03132541760401786, -21.04416526290806289, -0.7675724920830402365 ) ) ;
#5803=CARTESIAN_POINT ( 'NONE',  ( -16.17491895705301275, -18.95583473709189803, 25.04492750791695954 ) ) ;
#5804=CARTESIAN_POINT ( 'NONE',  ( -17.35725562635144215, -19.58745947852648683, 9.076177507916957765 ) ) ;
#5809=CARTESIAN_POINT ( 'NONE',  ( -9.754982604823302594, -29.00369391078756465, 39.70507249208304046 ) ) ;
#5811=CARTESIAN_POINT ( 'NONE',  ( -18.35725562635144925, -17.85540867095761186, 9.076177507916954212 ) ) ;
#5815=CARTESIAN_POINT ( 'NONE',  ( -13.64274437364857739, -21.31951028609534760, 6.673822492083044011 ) ) ;
#5818=CARTESIAN_POINT ( 'NONE',  ( -10.65656631922262321, -20.29120037471566462, 3.747711961066792630E-16 ) ) ;
#5820=CARTESIAN_POINT ( 'NONE',  ( -19.99999999999999645, -23.83517299489738051, 39.70117750791695954 ) ) ;
#5835=CARTESIAN_POINT ( 'NONE',  ( -20.04416526290808065, -25.17491895705300209, 2.732427507916957765 ) ) ;
#5836=CARTESIAN_POINT ( 'NONE',  ( -19.24771351637089367, -21.35725562635142438, 8.638677507916957765 ) ) ;
#5838=CARTESIAN_POINT ( 'NONE',  ( -17.35725562635140307, -28.41254052147349185, 4.048822492083041347 ) ) ;
#5842=CARTESIAN_POINT ( 'NONE',  ( -17.64274437364855430, -28.24771351637087236, 2.076177507916958209 ) ) ;
#5844=CARTESIAN_POINT ( 'NONE',  ( -11.21908421996108984, -20.46040770435011069, 10.16992750791695599 ) ) ;
#5856=CARTESIAN_POINT ( 'NONE',  ( -12.95952864787948755, -30.95583473709188382, 13.89257249208304046 ) ) ;
#5857=( NAMED_UNIT ( * ) PLANE_ANGLE_UNIT ( ) SI_UNIT ( $, .RADIAN. ) );
#5861=CARTESIAN_POINT ( 'NONE',  ( -17.68048971390461688, -25.35725562635141372, 18.26367750791696309 ) ) ;
#5863=CARTESIAN_POINT ( 'NONE',  ( -9.996306089212408708, -18.75498260482328661, 1.642572492083039126 ) ) ;
#5880=CARTESIAN_POINT ( 'NONE',  ( -7.999999999999996447, -24.16482700510256976, 21.32617750791695599 ) ) ;
#5885=CARTESIAN_POINT ( 'NONE',  ( -13.49542703274174116, -28.95583473709188738, 40.14257249208304756 ) ) ;
#5890=CARTESIAN_POINT ( 'NONE',  ( -12.04416526290807887, -24.96867458239596260, 0.5449275079169599856 ) ) ;
#5899=PRODUCT_CONTEXT ( 'NONE', #2313, 'mechanical' ) ;
#5907=CARTESIAN_POINT ( 'NONE',  ( -16.50457296725825174, -19.04416526290807354, 6.017572492083042235 ) ) ;
#5908=CARTESIAN_POINT ( 'NONE',  ( -9.754982604823348780, -18.99630608921234654, 4.919927507916955989 ) ) ;
#5910=CARTESIAN_POINT ( 'NONE',  ( -12.68318583509882380, -26.07549068051207541, 8.205072492083042235 ) ) ;
#5929=CARTESIAN_POINT ( 'NONE',  ( -17.35725562635144215, -19.58745947852648683, 9.076177507916957765 ) ) ;
#5930=CARTESIAN_POINT ( 'NONE',  ( -19.24771351637089367, -21.35725562635142438, 13.88867750791695954 ) ) ;
#5932=CARTESIAN_POINT ( 'NONE',  ( -11.46040770435014977, -20.21908421996103655, 1.642572492083041125 ) ) ;
#5936=CARTESIAN_POINT ( 'NONE',  ( -18.53959229564986799, -20.21908421996107563, 8.857427507916957765 ) ) ;
#5939=CARTESIAN_POINT ( 'NONE',  ( -18.53959229564986799, -20.21908421996107563, 8.857427507916957765 ) ) ;
#5953=CARTESIAN_POINT ( 'NONE',  ( -7.955834737091903364, -25.71081734191518464, 13.01757249208304046 ) ) ;
#5959=CARTESIAN_POINT ( 'NONE',  ( -12.48433729119798130, -25.64274437364855075, 21.76367750791695954 ) ) ;
#5961=CARTESIAN_POINT ( 'NONE',  ( -21.14459132904239169, -20.64274437364858628, 10.61132249208303868 ) ) ;
#5972=CARTESIAN_POINT ( 'NONE',  ( -10.42301891655615087, -22.26810260968755983, 4.401948939463558987E-14 ) ) ;
#5982=CARTESIAN_POINT ( 'NONE',  ( -21.95583473709191580, -21.95952864787954084, 18.91992750791695954 ) ) ;
#5987=CARTESIAN_POINT ( 'NONE',  ( -13.35725562635141195, -26.51566270880198672, 24.17382249208304046 ) ) ;
#5994=CARTESIAN_POINT ( 'NONE',  ( -13.64274437364856141, -26.68048971390460622, 6.451177507916961318 ) ) ;
#6009=CARTESIAN_POINT ( 'NONE',  ( -19.24771351637089367, -21.35725562635142438, 19.13867750791695954 ) ) ;
#6012=CARTESIAN_POINT ( 'NONE',  ( -16.50457296725825174, -19.04416526290807354, 21.76757249208304401 ) ) ;
#6017=CARTESIAN_POINT ( 'NONE',  ( -17.95583473709190869, -24.96867458239598037, 9.955072492083044011 ) ) ;
#6037=CARTESIAN_POINT ( 'NONE',  ( -19.99999999999999645, -23.83517299489738051, 13.45117750791695777 ) ) ;
#6040=CARTESIAN_POINT ( 'NONE',  ( -19.95583473709190514, -25.50457296725822687, 9.955072492083036906 ) ) ;
#6042=CARTESIAN_POINT ( 'NONE',  ( -13.82508104294698192, -29.04416526290806644, 6.669927507916955989 ) ) ;
#6044=CARTESIAN_POINT ( 'NONE',  ( -10.04416526290807710, -25.50457296725819489, 5.794927507916957765 ) ) ;
#6054=CARTESIAN_POINT ( 'NONE',  ( -11.35725562635139418, -29.97976432393972601, 24.17382249208304046 ) ) ;
#6059=CARTESIAN_POINT ( 'NONE',  ( -16.64274437364856496, -26.51566270880199738, 17.82617750791695954 ) ) ;
#6061=CARTESIAN_POINT ( 'NONE',  ( -22.04416526290807710, -25.71081734191525925, 39.48242750791695244 ) ) ;
#6078=ORIENTED_EDGE ( 'NONE', *, *, #4748, .F. ) ;
#6080=CARTESIAN_POINT ( 'NONE',  ( -8.855408670957631401, -20.64274437364852943, 15.63867750791696132 ) ) ;
#6084=CARTESIAN_POINT ( 'NONE',  ( -13.35725562635141195, -26.51566270880198672, 18.92382249208304401 ) ) ;
#6085=CARTESIAN_POINT ( 'NONE',  ( -13.28918265808472299, -31.04416526290805933, 22.41992750791695954 ) ) ;
#6090=CARTESIAN_POINT ( 'NONE',  ( -17.31681416490115311, -26.07549068051209318, 18.04492750791696309 ) ) ;
#6100=( GEOMETRIC_REPRESENTATION_CONTEXT ( 3 ) GLOBAL_UNCERTAINTY_ASSIGNED_CONTEXT ( ( #17466 ) ) GLOBAL_UNIT_ASSIGNED_CONTEXT ( ( #7519, #7319, #1245 ) ) REPRESENTATION_CONTEXT ( 'NONE', 'WORKASPACE' ) );
#6101=CARTESIAN_POINT ( 'NONE',  ( -17.35725562635144215, -19.58745947852648683, 40.57617750791696665 ) ) ;
#6103=CARTESIAN_POINT ( 'NONE',  ( -15.16482700510263371, -18.99999999999997868, 42.98632249208304046 ) ) ;
#6104=CARTESIAN_POINT ( 'NONE',  ( -17.35725562635144215, -19.58745947852648683, 14.32617750791695777 ) ) ;
#6108=CARTESIAN_POINT ( 'NONE',  ( -14.83517299489735741, -28.99999999999998224, 24.61132249208304401 ) ) ;
#6110=CARTESIAN_POINT ( 'NONE',  ( -12.31951028609536536, -25.35725562635139596, 23.73632249208304401 ) ) ;
#6115=CARTESIAN_POINT ( 'NONE',  ( -13.80790879128036153, -18.12502140183178412, 9.743381756881012649E-15 ) ) ;
#6130=CARTESIAN_POINT ( 'NONE',  ( -17.64274437364855430, -28.24771351637087236, 23.07617750791695954 ) ) ;
#6131=CARTESIAN_POINT ( 'NONE',  ( -11.21908421996108629, -20.46040770435011069, 15.41992750791695954 ) ) ;
#6134=CARTESIAN_POINT ( 'NONE',  ( -10.75228648362912232, -21.35725562635138530, 7.111322492083040459 ) ) ;
#6136=CARTESIAN_POINT ( 'NONE',  ( -9.999999999999994671, -24.16482700510257686, 0.3261775079169582647 ) ) ;
#6140=CARTESIAN_POINT ( 'NONE',  ( -14.83517299489739649, -18.99999999999997868, 20.01367750791695954 ) ) ;
#6154=CARTESIAN_POINT ( 'NONE',  ( -17.04047135212050890, -17.04416526290807710, 11.26757249208304046 ) ) ;
#6156=CARTESIAN_POINT ( 'NONE',  ( -16.50457296725825174, -19.04416526290807354, 11.26757249208304046 ) ) ;
#6160=ADVANCED_FACE ( 'NONE', ( #16215 ), #17016, .T. ) ;
#6161=CARTESIAN_POINT ( 'NONE',  ( -17.95583473709191580, -23.03132541760400898, 13.66992750791696309 ) ) ;
#6163=CARTESIAN_POINT ( 'NONE',  ( -7.955834737091903364, -25.71081734191518464, 7.767572492083039570 ) ) ;
#6185=CARTESIAN_POINT ( 'NONE',  ( -12.95952864787955150, -17.04416526290805933, 9.732427507916955989 ) ) ;
#6189=CARTESIAN_POINT ( 'NONE',  ( -12.68318583509882380, -26.07549068051207541, 13.45507249208304401 ) ) ;
#6194=CARTESIAN_POINT ( 'NONE',  ( -12.68318583509884157, -21.92450931948787485, 20.66992750791696665 ) ) ;
#6205=CARTESIAN_POINT ( 'NONE',  ( -11.21908421996108629, -20.46040770435011069, 36.41992750791695954 ) ) ;
#6207=CARTESIAN_POINT ( 'NONE',  ( -11.46040770435012668, -27.78091578003887463, 21.98242750791695244 ) ) ;
#6210=CARTESIAN_POINT ( 'NONE',  ( -10.75228648362912232, -21.35725562635138530, 17.61132249208304401 ) ) ;
#6212=CARTESIAN_POINT ( 'NONE',  ( -17.51566270880199738, -25.64274437364856496, 25.48632249208304401 ) ) ;
#6228=CARTESIAN_POINT ( 'NONE',  ( -11.46040770435012668, -27.78091578003887463, 21.98242750791695244 ) ) ;
#6230=CARTESIAN_POINT ( 'NONE',  ( -17.64274437364858983, -19.75228648362910633, 21.54882249208304401 ) ) ;
#6232=CARTESIAN_POINT ( 'NONE',  ( -19.24771351637089367, -21.35725562635142438, 13.88867750791695954 ) ) ;
#6235=CARTESIAN_POINT ( 'NONE',  ( -9.999999999999994671, -24.16482700510257686, 16.07617750791695954 ) ) ;
#6247=CARTESIAN_POINT ( 'NONE',  ( -7.999999999999996447, -23.83517299489733432, 12.79882249208303691 ) ) ;
#6250=CARTESIAN_POINT ( 'NONE',  ( -19.95583473709190514, -25.50457296725823042, 4.705072492083040459 ) ) ;
#6252=CARTESIAN_POINT ( 'NONE',  ( -13.35725562635142794, -21.48433729119796709, 15.20117750791696132 ) ) ;
#6254=CARTESIAN_POINT ( 'NONE',  ( -11.35725562635139418, -29.97976432393972601, 18.92382249208303691 ) ) ;
#6274=CARTESIAN_POINT ( 'NONE',  ( -16.71081734191527346, -16.95583473709190159, 19.79492750791695954 ) ) ;
#6278=CARTESIAN_POINT ( 'NONE',  ( -17.68048971390462754, -22.64274437364856496, 15.86132249208304401 ) ) ;
#6279=CARTESIAN_POINT ( 'NONE',  ( -14.83517299489740715, -16.99999999999997868, 9.513677507916955989 ) ) ;
#6286=CARTESIAN_POINT ( 'NONE',  ( -13.64274437364856141, -26.68048971390460622, 16.95117750791696309 ) ) ;
#6301=CARTESIAN_POINT ( 'NONE',  ( -17.64274437364855430, -28.24771351637087236, 38.82617750791695954 ) ) ;
#6304=CARTESIAN_POINT ( 'NONE',  ( -17.64274437364855430, -28.24771351637087236, 12.57617750791695777 ) ) ;
#6308=CARTESIAN_POINT ( 'NONE',  ( -17.64274437364858983, -19.75228648362910633, 11.04882249208304046 ) ) ;
#6311=CARTESIAN_POINT ( 'NONE',  ( -18.04416526290808775, -23.36097942780924441, 20.89257249208304046 ) ) ;
#6332=CARTESIAN_POINT ( 'NONE',  ( -16.50457296725820555, -28.95583473709189448, 17.60742750791695599 ) ) ;
#6334=CARTESIAN_POINT ( 'NONE',  ( -19.99999999999999645, -24.16482700510261949, 15.42382249208304046 ) ) ;
#6337=CARTESIAN_POINT ( 'NONE',  ( -18.78091578003889950, -27.53959229564985378, 23.29492750791695954 ) ) ;
#6339=CARTESIAN_POINT ( 'NONE',  ( -19.95583473709191225, -22.49542703274176603, 13.66992750791695599 ) ) ;
#6353=CARTESIAN_POINT ( 'NONE',  ( -21.14459132904239169, -20.64274437364858628, 26.36132249208303691 ) ) ;
#6355=CARTESIAN_POINT ( 'NONE',  ( -13.82508104294702100, -18.95583473709188382, 6.455072492083042235 ) ) ;
#6357=CARTESIAN_POINT ( 'NONE',  ( -15.16482700510260706, -26.99999999999998579, 22.63867750791696309 ) ) ;
#6359=CARTESIAN_POINT ( 'NONE',  ( -22.04416526290809486, -22.28918265808477628, 15.64257249208304223 ) ) ;
#6375=CARTESIAN_POINT ( 'NONE',  ( -11.35725562635144925, -18.02023567606020293, 30.95117750791695954 ) ) ;
#6378=CARTESIAN_POINT ( 'NONE',  ( -14.36097942780925685, -20.95583473709189093, 16.95507249208304046 ) ) ;
#6381=CARTESIAN_POINT ( 'NONE',  ( -7.955834737091916686, -22.28918265808470522, 10.60742750791695599 ) ) ;
#6385=CARTESIAN_POINT ( 'NONE',  ( -17.07549068051210739, -21.68318583509881847, 19.35742750791695954 ) ) ;
#6403=CARTESIAN_POINT ( 'NONE',  ( -10.04416526290807710, -25.50457296725819489, 11.04492750791695421 ) ) ;
#6406=CARTESIAN_POINT ( 'NONE',  ( -11.46040770435014977, -20.21908421996103655, 17.39257249208304401 ) ) ;
#6408=CARTESIAN_POINT ( 'NONE',  ( -17.95583473709190869, -24.96867458239598037, 20.45507249208304401 ) ) ;
#6425=CARTESIAN_POINT ( 'NONE',  ( -10.58745947852649927, -21.64274437364853654, 15.63867750791695777 ) ) ;
#6428=CARTESIAN_POINT ( 'NONE',  ( -19.99999999999999645, -24.16482700510261949, 20.67382249208304401 ) ) ;
#6430=CARTESIAN_POINT ( 'NONE',  ( -11.21908421996108629, -20.46040770435011069, 15.41992750791695954 ) ) ;
#6432=CARTESIAN_POINT ( 'NONE',  ( -17.64274437364855430, -28.24771351637087236, 23.07617750791695954 ) ) ;
#6434=CARTESIAN_POINT ( 'NONE',  ( -17.64274437364858983, -19.75228648362910633, 21.54882249208304401 ) ) ;
#6445=CARTESIAN_POINT ( 'NONE',  ( -16.71081734191520596, -31.04416526290808065, 30.08007249208304046 ) ) ;
#6447=CARTESIAN_POINT ( 'NONE',  ( -19.24771351637086880, -26.64274437364857206, 4.486322492083041347 ) ) ;
#6449=CARTESIAN_POINT ( 'NONE',  ( -17.31681416490115311, -26.07549068051209318, 33.79492750791695954 ) ) ;
#6451=CARTESIAN_POINT ( 'NONE',  ( -14.83517299489734853, -30.99999999999998224, 24.61132249208304046 ) ) ;
#6467=ORIENTED_EDGE ( 'NONE', *, *, #12749, .F. ) ;
#6470=CARTESIAN_POINT ( 'NONE',  ( -12.95952864787955150, -17.04416526290805933, 35.98242750791695244 ) ) ;
#6474=CARTESIAN_POINT ( 'NONE',  ( -17.31681416490117087, -21.92450931948788551, 26.58007249208304756 ) ) ;
#6475=CARTESIAN_POINT ( 'NONE',  ( -20.24501739517664234, -29.00369391078761439, 12.79492750791695599 ) ) ;
#6479=CARTESIAN_POINT ( 'NONE',  ( -12.92450931948788906, -26.31681416490114245, 21.98242750791695954 ) ) ;
#6498=CARTESIAN_POINT ( 'NONE',  ( -12.35725562635143682, -19.75228648362908501, 30.95117750791695954 ) ) ;
#6503=CARTESIAN_POINT ( 'NONE',  ( -19.95583473709190514, -25.50457296725822687, 36.20507249208303335 ) ) ;
#6505=CARTESIAN_POINT ( 'NONE',  ( -12.68318583509882380, -26.07549068051207541, 23.95507249208304756 ) ) ;
#6519=CARTESIAN_POINT ( 'NONE',  ( -9.955834737091912245, -22.82508104294696594, 21.10742750791695599 ) ) ;
#6521=CARTESIAN_POINT ( 'NONE',  ( -11.46040770435014977, -20.21908421996103655, 22.64257249208303335 ) ) ;
#6525=CARTESIAN_POINT ( 'NONE',  ( -13.49542703274178379, -19.04416526290806289, 14.98242750791695777 ) ) ;
#6528=CARTESIAN_POINT ( 'NONE',  ( -14.83517299489739649, -18.99999999999997868, 35.76367750791695954 ) ) ;
#6530=CARTESIAN_POINT ( 'NONE',  ( -19.99999999999999645, -24.16482700510261949, 20.67382249208304401 ) ) ;
#6541=CARTESIAN_POINT ( 'NONE',  ( -8.044165262908093084, -21.95952864787946979, 33.58007249208304046 ) ) ;
#6542=CARTESIAN_POINT ( 'NONE',  ( -18.78091578003892792, -20.46040770435013556, 16.08007249208304046 ) ) ;
#6545=CARTESIAN_POINT ( 'NONE',  ( -17.99999999999999645, -23.83517299489736985, 23.95117750791696309 ) ) ;
#6548=CARTESIAN_POINT ( 'NONE',  ( -11.35725562635139418, -29.97976432393972601, 13.67382249208304046 ) ) ;
#6564=CARTESIAN_POINT ( 'NONE',  ( -9.020235676060220698, -27.64274437364852588, 32.26367750791695244 ) ) ;
#6572=CARTESIAN_POINT ( 'NONE',  ( -16.64274437364858272, -21.48433729119797420, 32.04882249208304756 ) ) ;
#6573=CARTESIAN_POINT ( 'NONE',  ( -20.24501739517664234, -29.00369391078761439, 23.29492750791695599 ) ) ;
#6578=CARTESIAN_POINT ( 'NONE',  ( -14.83517299489738761, -20.99999999999997513, 25.26367750791696309 ) ) ;
#6596=CARTESIAN_POINT ( 'NONE',  ( -13.49542703274178379, -19.04416526290806289, 30.73242750791695599 ) ) ;
#6602=CARTESIAN_POINT ( 'NONE',  ( -12.64274437364858628, -19.58745947852646552, 38.17382249208304046 ) ) ;
#6604=CARTESIAN_POINT ( 'NONE',  ( -14.03132541760400009, -26.95583473709189448, 34.89257249208305467 ) ) ;
#6620=CARTESIAN_POINT ( 'NONE',  ( -17.64274437364855430, -28.24771351637087236, 28.32617750791695954 ) ) ;
#6623=CARTESIAN_POINT ( 'NONE',  ( -14.83517299489735741, -28.99999999999998224, 24.61132249208304401 ) ) ;
#6626=CARTESIAN_POINT ( 'NONE',  ( -20.04416526290808065, -25.17491895705300209, 18.48242750791695954 ) ) ;
#6629=CARTESIAN_POINT ( 'NONE',  ( -11.46040770435012490, -27.78091578003888173, 27.23242750791695599 ) ) ;
#6631=CARTESIAN_POINT ( 'NONE',  ( -14.83517299489735741, -28.99999999999998224, 24.61132249208304401 ) ) ;
#6642=CARTESIAN_POINT ( 'NONE',  ( -12.95952864787948755, -30.95583473709188382, 29.64257249208304401 ) ) ;
#6644=CARTESIAN_POINT ( 'NONE',  ( -14.36097942780923731, -27.04416526290806999, 27.66992750791696665 ) ) ;
#6646=CARTESIAN_POINT ( 'NONE',  ( -11.35725562635139418, -29.97976432393972601, 24.17382249208304046 ) ) ;
#6662=CARTESIAN_POINT ( 'NONE',  ( -16.71081734191527346, -16.95583473709190159, 30.29492750791696665 ) ) ;
#6666=CARTESIAN_POINT ( 'NONE',  ( -17.99999999999999645, -24.16482700510260173, 25.92382249208304756 ) ) ;
#6668=CARTESIAN_POINT ( 'NONE',  ( -11.35725562635144925, -18.02023567606020293, 20.45117750791695954 ) ) ;
#6674=CARTESIAN_POINT ( 'NONE',  ( -17.68048971390461688, -25.35725562635141372, 28.76367750791696309 ) ) ;
#6688=CARTESIAN_POINT ( 'NONE',  ( -19.24771351637089367, -21.35725562635142438, 29.63867750791695599 ) ) ;
#6691=CARTESIAN_POINT ( 'NONE',  ( -17.64274437364858983, -19.75228648362910633, 26.79882249208304401 ) ) ;
#6694=CARTESIAN_POINT ( 'NONE',  ( -14.36097942780925685, -20.95583473709189093, 27.45507249208304756 ) ) ;
#6705=CARTESIAN_POINT ( 'NONE',  ( -12.35725562635143682, -19.75228648362908501, 30.95117750791695954 ) ) ;
#6708=CARTESIAN_POINT ( 'NONE',  ( -16.50457296725825174, -19.04416526290807354, 27.01757249208304046 ) ) ;
#6711=CARTESIAN_POINT ( 'NONE',  ( -15.16482700510259640, -28.99999999999998224, 27.88867750791695954 ) ) ;
#6713=CARTESIAN_POINT ( 'NONE',  ( -15.16482700510259640, -28.99999999999998224, 38.38867750791695954 ) ) ;
#6715=CARTESIAN_POINT ( 'NONE',  ( -17.64274437364858983, -19.75228648362910633, 26.79882249208304401 ) ) ;
#6728=CARTESIAN_POINT ( 'NONE',  ( -13.35725562635142794, -21.48433729119796709, 30.95117750791695954 ) ) ;
#6731=CARTESIAN_POINT ( 'NONE',  ( -9.020235676060250896, -20.35725562635137820, 38.61132249208304046 ) ) ;
#6745=CARTESIAN_POINT ( 'NONE',  ( -11.64274437364854187, -30.14459132904234195, 27.45117750791696309 ) ) ;
#6752=CARTESIAN_POINT ( 'NONE',  ( -17.07549068051208963, -26.31681416490115311, 30.51757249208304756 ) ) ;
#6753=CARTESIAN_POINT ( 'NONE',  ( -12.95952864787955150, -17.04416526290805933, 35.98242750791695244 ) ) ;
#6759=CARTESIAN_POINT ( 'NONE',  ( -14.36097942780923731, -27.04416526290806999, 32.91992750791696665 ) ) ;
#6779=CARTESIAN_POINT ( 'NONE',  ( -16.50457296725820555, -28.95583473709189448, 33.35742750791695954 ) ) ;
#6782=CARTESIAN_POINT ( 'NONE',  ( -10.04416526290808953, -22.49542703274172695, 28.33007249208304401 ) ) ;
#6787=CARTESIAN_POINT ( 'NONE',  ( -17.31681416490117087, -21.92450931948788551, 37.08007249208304756 ) ) ;
#6801=CARTESIAN_POINT ( 'NONE',  ( -17.35725562635144215, -19.58745947852648683, 35.32617750791695954 ) ) ;
#6804=CARTESIAN_POINT ( 'NONE',  ( -15.16482700510263371, -18.99999999999997868, 32.48632249208304046 ) ) ;
#6806=CARTESIAN_POINT ( 'NONE',  ( -16.17491895705301275, -18.95583473709189803, 25.04492750791695954 ) ) ;
#6808=CARTESIAN_POINT ( 'NONE',  ( -13.82508104294698015, -29.04416526290806289, 38.16992750791695954 ) ) ;
#6810=CARTESIAN_POINT ( 'NONE',  ( -12.35725562635140307, -28.24771351637085459, 18.92382249208304401 ) ) ;
#6819=CARTESIAN_POINT ( 'NONE',  ( -17.07549068051210739, -21.68318583509881847, 40.35742750791696665 ) ) ;
#6821=CARTESIAN_POINT ( 'NONE',  ( -9.754982604823302594, -29.00369391078756465, 29.20507249208304046 ) ) ;
#6834=CARTESIAN_POINT ( 'NONE',  ( -22.04416526290809486, -22.28918265808477628, 5.142572492083038682 ) ) ;
#6838=CARTESIAN_POINT ( 'NONE',  ( -14.03132541760400009, -26.95583473709189448, 29.64257249208304401 ) ) ;
#6839=CARTESIAN_POINT ( 'NONE',  ( -13.28918265808472299, -31.04416526290805933, 27.66992750791695954 ) ) ;
#6860=ORIENTED_EDGE ( 'NONE', *, *, #975, .T. ) ;
#6861=CARTESIAN_POINT ( 'NONE',  ( -12.35725562635143682, -19.75228648362908501, 36.20117750791695954 ) ) ;
#6866=CARTESIAN_POINT ( 'NONE',  ( -11.46040770435014977, -20.21908421996103655, 27.89257249208303335 ) ) ;
#6871=CARTESIAN_POINT ( 'NONE',  ( -12.31951028609536536, -25.35725562635139596, 28.98632249208304401 ) ) ;
#6881=CARTESIAN_POINT ( 'NONE',  ( -9.999999999999994671, -24.16482700510257686, 31.82617750791696309 ) ) ;
#6891=CARTESIAN_POINT ( 'NONE',  ( -10.04416526290807710, -25.50457296725819489, 32.04492750791695954 ) ) ;
#6894=CARTESIAN_POINT ( 'NONE',  ( -9.999999999999994671, -23.83517299489734143, 28.54882249208304401 ) ) ;
#6898=CARTESIAN_POINT ( 'NONE',  ( -12.64274437364855252, -28.41254052147347053, 32.70117750791696665 ) ) ;
#6900=CARTESIAN_POINT ( 'NONE',  ( -10.04416526290807710, -25.50457296725819489, 26.79492750791695954 ) ) ;
#6914=CARTESIAN_POINT ( 'NONE',  ( -10.04416526290807710, -25.50457296725819489, 5.794927507916955989 ) ) ;
#6917=CARTESIAN_POINT ( 'NONE',  ( -21.14459132904239169, -20.64274437364858628, 26.36132249208303691 ) ) ;
#6933=CARTESIAN_POINT ( 'NONE',  ( -21.99999999999999289, -24.16482700510262305, 10.17382249208303868 ) ) ;
#6938=CARTESIAN_POINT ( 'NONE',  ( -14.36097942780923731, -27.04416526290806999, 6.669927507916960430 ) ) ;
#6939=CARTESIAN_POINT ( 'NONE',  ( -8.044165262908075320, -26.04047135212042718, 32.04492750791695954 ) ) ;
#6959=CARTESIAN_POINT ( 'NONE',  ( -21.95583473709191580, -21.95952864787954084, 8.419927507916955989 ) ) ;
#6963=CARTESIAN_POINT ( 'NONE',  ( -16.64274437364858272, -21.48433729119797420, 5.798822492083043123 ) ) ;
#6967=CARTESIAN_POINT ( 'NONE',  ( -17.68048971390462754, -22.64274437364856496, 36.86132249208304046 ) ) ;
#6978=CARTESIAN_POINT ( 'NONE',  ( -10.75228648362910100, -26.64274437364854009, 21.76367750791695599 ) ) ;
#6985=CARTESIAN_POINT ( 'NONE',  ( -11.64274437364859693, -17.85540867095757989, 32.92382249208303335 ) ) ;
#6986=CARTESIAN_POINT ( 'NONE',  ( -11.21908421996108629, -20.46040770435011069, 31.16992750791695599 ) ) ;
#6988=CARTESIAN_POINT ( 'NONE',  ( -12.64274437364858628, -19.58745947852646552, 27.67382249208304046 ) ) ;
#6992=CARTESIAN_POINT ( 'NONE',  ( -14.83517299489739649, -18.99999999999997868, 30.51367750791695954 ) ) ;
#7008=CARTESIAN_POINT ( 'NONE',  ( -10.58745947852649927, -21.64274437364853654, -0.1113224920830418047 ) ) ;
#7010=CARTESIAN_POINT ( 'NONE',  ( -11.64274437364859693, -17.85540867095757989, 32.92382249208303335 ) ) ;
#7024=CARTESIAN_POINT ( 'NONE',  ( -8.044165262908093084, -21.95952864787946979, 7.330072492083040459 ) ) ;
#7029=CARTESIAN_POINT ( 'NONE',  ( -17.31681416490117087, -21.92450931948788551, 42.33007249208304756 ) ) ;
#7030=CARTESIAN_POINT ( 'NONE',  ( -7.955834737091916686, -22.28918265808470522, 26.35742750791695954 ) ) ;
#7046=AXIS2_PLACEMENT_3D ( 'NONE', #6103, #12067, #11671 ) ;
#7053=CARTESIAN_POINT ( 'NONE',  ( -8.855408670957631401, -20.64274437364852943, -0.1113224920830435533 ) ) ;
#7056=CARTESIAN_POINT ( 'NONE',  ( -17.95583473709190869, -24.96867458239598037, 9.955072492083044011 ) ) ;
#7060=CARTESIAN_POINT ( 'NONE',  ( -14.83517299489738761, -20.99999999999997513, 9.513677507916957765 ) ) ;
#7068=EDGE_CURVE ( 'NONE', #15887, #18550, #18281, .T. ) ;
#7073=CARTESIAN_POINT ( 'NONE',  ( -9.955834737091912245, -22.82508104294696594, 26.35742750791695954 ) ) ;
#7081=CARTESIAN_POINT ( 'NONE',  ( -16.17491895705296656, -29.04416526290807710, 9.080072492083036906 ) ) ;
#7082=CARTESIAN_POINT ( 'NONE',  ( -9.754982604823348780, -18.99630608921234654, -0.3300724920830435116 ) ) ;
#7084=CARTESIAN_POINT ( 'NONE',  ( -15.96867458239599635, -21.04416526290806999, 11.26757249208304579 ) ) ;
#7088=CARTESIAN_POINT ( 'NONE',  ( -10.58745947852649927, -21.64274437364853654, 31.38867750791696309 ) ) ;
#7094=CARTESIAN_POINT ( 'NONE',  ( -12.35725562635140307, -28.24771351637085459, 34.67382249208304046 ) ) ;
#7104=CARTESIAN_POINT ( 'NONE',  ( -13.82508104294698192, -29.04416526290806644, 6.669927507916955989 ) ) ;
#7106=CARTESIAN_POINT ( 'NONE',  ( -16.50457296725820555, -28.95583473709189448, 1.857427507916957765 ) ) ;
#7109=CARTESIAN_POINT ( 'NONE',  ( -8.855408670957602979, -27.35725562635137820, 28.98632249208304401 ) ) ;
#7111=CARTESIAN_POINT ( 'NONE',  ( -17.51566270880201159, -22.35725562635141728, 34.88867750791696665 ) ) ;
#7112=CARTESIAN_POINT ( 'NONE',  ( -16.17491895705301275, -18.95583473709189448, 9.294927507916955989 ) ) ;
#7123=CARTESIAN_POINT ( 'NONE',  ( -22.04416526290809486, -22.28918265808477628, 10.39257249208303691 ) ) ;
#7128=CARTESIAN_POINT ( 'NONE',  ( -17.07549068051208963, -26.31681416490115311, 41.01757249208304756 ) ) ;
#7129=CARTESIAN_POINT ( 'NONE',  ( -17.04047135212043784, -30.95583473709190159, 28.10742750791695954 ) ) ;
#7149=CARTESIAN_POINT ( 'NONE',  ( -12.95952864787955150, -17.04416526290805933, 4.482427507916956877 ) ) ;
#7153=CARTESIAN_POINT ( 'NONE',  ( -19.24771351637086880, -26.64274437364857206, 41.23632249208304046 ) ) ;
#7156=CARTESIAN_POINT ( 'NONE',  ( -15.16482700510262482, -20.99999999999997513, 42.98632249208304756 ) ) ;
#7168=CARTESIAN_POINT ( 'NONE',  ( -12.64274437364855252, -28.41254052147347053, 32.70117750791696665 ) ) ;
#7170=CARTESIAN_POINT ( 'NONE',  ( -10.75228648362910100, -26.64274437364854009, 0.7636775079169582092 ) ) ;
#7174=CARTESIAN_POINT ( 'NONE',  ( -21.95583473709189803, -26.04047135212049469, 41.45507249208303335 ) ) ;
#7176=CARTESIAN_POINT ( 'NONE',  ( -11.35725562635144925, -18.02023567606020293, 4.701177507916955989 ) ) ;
#7179=CARTESIAN_POINT ( 'NONE',  ( -20.04416526290809131, -22.82508104294699791, 41.89257249208301914 ) ) ;
#7188=CARTESIAN_POINT ( 'NONE',  ( -12.64274437364858628, -19.58745947852646552, 32.92382249208304046 ) ) ;
#7200=CARTESIAN_POINT ( 'NONE',  ( -10.58745947852649927, -21.64274437364853654, 10.38867750791695777 ) ) ;
#7202=CARTESIAN_POINT ( 'NONE',  ( -12.64274437364855252, -28.41254052147347053, 1.201177507916958431 ) ) ;
#7204=CARTESIAN_POINT ( 'NONE',  ( -19.99999999999999645, -24.16482700510261949, 4.923822492083040459 ) ) ;
#7207=CARTESIAN_POINT ( 'NONE',  ( -11.99999999999999289, -24.16482700510258752, 37.07617750791695954 ) ) ;
#7208=CARTESIAN_POINT ( 'NONE',  ( -18.78091578003889595, -27.53959229564985023, 2.294927507916958209 ) ) ;
#7223=CARTESIAN_POINT ( 'NONE',  ( -16.71081734191520596, -31.04416526290808065, 9.080072492083038682 ) ) ;
#7224=( NAMED_UNIT ( * ) SI_UNIT ( $, .STERADIAN. ) SOLID_ANGLE_UNIT ( ) );
#7229=CARTESIAN_POINT ( 'NONE',  ( -14.36097942780923731, -27.04416526290806999, 1.419927507916959986 ) ) ;
#7230=CARTESIAN_POINT ( 'NONE',  ( -13.28918265808478694, -16.95583473709189093, 11.70507249208304046 ) ) ;
#7254=CARTESIAN_POINT ( 'NONE',  ( -19.24771351637089367, -21.35725562635142438, 40.13867750791695954 ) ) ;
#7258=CARTESIAN_POINT ( 'NONE',  ( -17.07549068051208963, -26.31681416490115311, 4.267572492083044011 ) ) ;
#7261=CARTESIAN_POINT ( 'NONE',  ( -12.31951028609537602, -22.64274437364854364, -0.1113224920830400977 ) ) ;
#7269=SHAPE_REPRESENTATION ( 'spring', ( #1791 ), #2725 ) ;
#7274=CARTESIAN_POINT ( 'NONE',  ( -19.24771351637089367, -21.35725562635142438, 29.63867750791695599 ) ) ;
#7276=CARTESIAN_POINT ( 'NONE',  ( -19.24771351637089367, -21.35725562635142438, 8.638677507916957765 ) ) ;
#7279=CARTESIAN_POINT ( 'NONE',  ( -16.17491895705296656, -29.04416526290807710, 3.830072492083041347 ) ) ;
#7280=CARTESIAN_POINT ( 'NONE',  ( -9.020235676060220698, -27.64274437364852588, 0.7636775079169565439 ) ) ;
#7282=CARTESIAN_POINT ( 'NONE',  ( -14.36097942780925685, -20.95583473709189093, 6.455072492083044899 ) ) ;
#7285=CARTESIAN_POINT ( 'NONE',  ( -10.18851321905033913, -22.11378838432466409, 4.586222366145915297E-17 ) ) ;
#7289=CARTESIAN_POINT ( 'NONE',  ( -16.17491895705301275, -18.95583473709189448, 40.79492750791696665 ) ) ;
#7291=CARTESIAN_POINT ( 'NONE',  ( -15.16482700510263371, -18.99999999999997868, 32.48632249208304046 ) ) ;
#7294=SURFACE_STYLE_FILL_AREA ( #13558 ) ;
#7298=CARTESIAN_POINT ( 'NONE',  ( -16.50457296725820555, -28.95583473709189448, 1.857427507916957765 ) ) ;
#7299=CARTESIAN_POINT ( 'NONE',  ( -15.16482700510259640, -28.99999999999998224, 17.38867750791695599 ) ) ;
#7301=CARTESIAN_POINT ( 'NONE',  ( -16.71081734191520596, -31.04416526290808065, 40.58007249208304756 ) ) ;
#7303=CARTESIAN_POINT ( 'NONE',  ( -12.92450931948788906, -26.31681416490114245, 37.73242750791696665 ) ) ;
#7304=CARTESIAN_POINT ( 'NONE',  ( -13.49542703274178201, -19.04416526290806289, 9.732427507916957765 ) ) ;
#7317=CARTESIAN_POINT ( 'NONE',  ( -21.14459132904239169, -20.64274437364858628, 21.11132249208304046 ) ) ;
#7319=( NAMED_UNIT ( * ) PLANE_ANGLE_UNIT ( ) SI_UNIT ( $, .RADIAN. ) );
#7323=CARTESIAN_POINT ( 'NONE',  ( -12.68318583509884157, -21.92450931948787485, 4.919927507916961318 ) ) ;
#7325=CARTESIAN_POINT ( 'NONE',  ( -21.95583473709189803, -26.04047135212049469, 4.705072492083038682 ) ) ;
#7342=CARTESIAN_POINT ( 'NONE',  ( -14.83517299489740715, -16.99999999999997868, 14.76367750791695777 ) ) ;
#7348=CARTESIAN_POINT ( 'NONE',  ( -12.48433729119799196, -22.35725562635139596, 7.111322492083044011 ) ) ;
#7354=CARTESIAN_POINT ( 'NONE',  ( -14.03132541760400009, -26.95583473709189448, 40.14257249208306177 ) ) ;
#7367=CARTESIAN_POINT ( 'NONE',  ( -10.75228648362910100, -26.64274437364854009, 37.51367750791695954 ) ) ;
#7369=CARTESIAN_POINT ( 'NONE',  ( -15.16482700510259640, -28.99999999999998224, 1.638677507916958431 ) ) ;
#7373=CARTESIAN_POINT ( 'NONE',  ( -18.35725562635138886, -30.14459132904237393, 40.79882249208304046 ) ) ;
#7376=CARTESIAN_POINT ( 'NONE',  ( -21.99999999999999289, -23.83517299489739116, 2.951177507916956433 ) ) ;
#7379=CARTESIAN_POINT ( 'NONE',  ( -19.99999999999999645, -24.16482700510261949, 41.67382249208304046 ) ) ;
#7398=CARTESIAN_POINT ( 'NONE',  ( -19.24771351637089367, -21.35725562635142438, 8.638677507916957765 ) ) ;
#7399=CARTESIAN_POINT ( 'NONE',  ( -17.35725562635144215, -19.58745947852648683, 19.57617750791695954 ) ) ;
#7401=CARTESIAN_POINT ( 'NONE',  ( -13.82508104294702100, -18.95583473709188382, 6.455072492083041347 ) ) ;
#7405=CARTESIAN_POINT ( 'NONE',  ( -11.21908421996108629, -20.46040770435011069, -0.3300724920830416798 ) ) ;
#7406=CARTESIAN_POINT ( 'NONE',  ( -11.46040770435012490, -27.78091578003888173, 11.48242750791695777 ) ) ;
#7419=CARTESIAN_POINT ( 'NONE',  ( -16.71081734191520596, -31.04416526290808065, 14.33007249208304046 ) ) ;
#7423=CARTESIAN_POINT ( 'NONE',  ( -11.99999999999999289, -24.16482700510258752, 21.32617750791695954 ) ) ;
#7425=CARTESIAN_POINT ( 'NONE',  ( -22.04416526290809486, -22.28918265808477628, 5.142572492083038682 ) ) ;
#7433=CARTESIAN_POINT ( 'NONE',  ( -13.25540099147408846, -20.31871257162172739, 7.657166918419680705E-13 ) ) ;
#7443=CARTESIAN_POINT ( 'NONE',  ( -21.99999999999999289, -23.83517299489739116, 18.70117750791695599 ) ) ;
#7447=CARTESIAN_POINT ( 'NONE',  ( -11.95583473709190514, -24.63902057219072361, 23.51757249208304401 ) ) ;
#7452=CARTESIAN_POINT ( 'NONE',  ( -14.83517299489738761, -20.99999999999997513, -0.9863224920830401254 ) ) ;
#7467=CARTESIAN_POINT ( 'NONE',  ( -16.17491895705301275, -18.95583473709189803, 19.79492750791695954 ) ) ;
#7470=CARTESIAN_POINT ( 'NONE',  ( -21.99999999999999289, -24.16482700510262305, 41.67382249208304756 ) ) ;
#7472=CARTESIAN_POINT ( 'NONE',  ( -12.31951028609536536, -25.35725562635139596, 2.736322492083043123 ) ) ;
#7493=CARTESIAN_POINT ( 'NONE',  ( -15.16482700510259640, -28.99999999999998224, 1.638677507916958431 ) ) ;
#7494=CARTESIAN_POINT ( 'NONE',  ( -18.78091578003889950, -27.53959229564985378, 12.79492750791695421 ) ) ;
#7496=CARTESIAN_POINT ( 'NONE',  ( -16.17491895705296656, -29.04416526290807710, 9.080072492083036906 ) ) ;
#7499=CARTESIAN_POINT ( 'NONE',  ( -17.68048971390461688, -25.35725562635141372, 39.26367750791696665 ) ) ;
#7501=CARTESIAN_POINT ( 'NONE',  ( -16.17491895705301275, -18.95583473709189448, 4.044927507916959541 ) ) ;
#7517=CARTESIAN_POINT ( 'NONE',  ( -13.28918265808478694, -16.95583473709189093, 22.20507249208304046 ) ) ;
#7519=( LENGTH_UNIT ( ) NAMED_UNIT ( * ) SI_UNIT ( .MILLI., .METRE. ) );
#7523=CARTESIAN_POINT ( 'NONE',  ( -16.64274437364856496, -26.51566270880199738, 12.57617750791695954 ) ) ;
#7525=CARTESIAN_POINT ( 'NONE',  ( -11.35725562635139418, -29.97976432393972601, 3.173822492083039126 ) ) ;
#7544=CARTESIAN_POINT ( 'NONE',  ( -20.00369391078762860, -18.75498260482333279, 14.10742750791695777 ) ) ;
#7549=CARTESIAN_POINT ( 'NONE',  ( -12.92450931948790149, -21.68318583509881137, 17.39257249208304046 ) ) ;
#7553=CARTESIAN_POINT ( 'NONE',  ( -16.35725562635142794, -21.31951028609535470, 19.57617750791696309 ) ) ;
#7569=CARTESIAN_POINT ( 'NONE',  ( -14.83517299489739649, -18.99999999999997868, 35.76367750791695954 ) ) ;
#7571=CARTESIAN_POINT ( 'NONE',  ( -9.955834737091912245, -22.82508104294696594, 10.60742750791695777 ) ) ;
#7575=CARTESIAN_POINT ( 'NONE',  ( -12.35725562635140307, -28.24771351637085459, 13.67382249208304223 ) ) ;
#7579=CARTESIAN_POINT ( 'NONE',  ( -18.04416526290808775, -23.36097942780924441, 15.64257249208304579 ) ) ;
#7597=CARTESIAN_POINT ( 'NONE',  ( -20.04416526290808065, -25.17491895705300209, 13.23242750791695777 ) ) ;
#7598=CARTESIAN_POINT ( 'NONE',  ( -13.49542703274178379, -19.04416526290806289, 14.98242750791695777 ) ) ;
#7600=CARTESIAN_POINT ( 'NONE',  ( -18.35725562635138886, -30.14459132904237393, 40.79882249208304046 ) ) ;
#7604=CARTESIAN_POINT ( 'NONE',  ( -15.16482700510260706, -26.99999999999998579, 38.38867750791695954 ) ) ;
#7607=CARTESIAN_POINT ( 'NONE',  ( -10.75228648362910100, -26.64274437364854009, 16.51367750791695954 ) ) ;
#7621=CARTESIAN_POINT ( 'NONE',  ( -14.83517299489734853, -30.99999999999998224, 14.11132249208304046 ) ) ;
#7626=CARTESIAN_POINT ( 'NONE',  ( -12.48433729119798130, -25.64274437364855075, 16.51367750791695954 ) ) ;
#7628=CARTESIAN_POINT ( 'NONE',  ( -13.28918265808478694, -16.95583473709189093, 1.205072492083039126 ) ) ;
#7645=CARTESIAN_POINT ( 'NONE',  ( -7.999999999999996447, -24.16482700510256976, 10.82617750791695599 ) ) ;
#7646=DIRECTION ( 'NONE',  ( 1.000000000000000000, 0.000000000000000000, 0.000000000000000000 ) ) ;
#7650=CARTESIAN_POINT ( 'NONE',  ( -11.99999999999999289, -23.83517299489735564, 12.79882249208304223 ) ) ;
#7655=CARTESIAN_POINT ( 'NONE',  ( -15.63902057219076269, -20.95583473709189448, 14.54492750791695954 ) ) ;
#7667=CARTESIAN_POINT ( 'NONE',  ( -19.95583473709191580, -22.49542703274176603, 39.91992750791695954 ) ) ;
#7670=CARTESIAN_POINT ( 'NONE',  ( -11.21908421996108629, -20.46040770435011069, 10.16992750791695244 ) ) ;
#7674=CARTESIAN_POINT ( 'NONE',  ( -15.16482700510263371, -18.99999999999997868, 11.48632249208304046 ) ) ;
#7676=CARTESIAN_POINT ( 'NONE',  ( -15.63902057219073605, -27.04416526290807710, 24.83007249208304046 ) ) ;
#7696=CARTESIAN_POINT ( 'NONE',  ( -18.53959229564986799, -20.21908421996107563, 24.60742750791695954 ) ) ;
#7699=CARTESIAN_POINT ( 'NONE',  ( -10.04416526290808953, -22.49542703274172695, 17.83007249208303691 ) ) ;
#7701=CARTESIAN_POINT ( 'NONE',  ( -19.41254052147348830, -26.35725562635142083, 18.26367750791695599 ) ) ;
#7704=CARTESIAN_POINT ( 'NONE',  ( -20.04416526290808065, -25.17491895705300209, 23.73242750791695599 ) ) ;
#7720=CARTESIAN_POINT ( 'NONE',  ( -15.16482700510264436, -16.99999999999997868, 21.98632249208304046 ) ) ;
#7724=CARTESIAN_POINT ( 'NONE',  ( -16.50457296725825174, -19.04416526290807354, 6.017572492083041347 ) ) ;
#7727=CARTESIAN_POINT ( 'NONE',  ( -14.83517299489738761, -20.99999999999997513, 20.01367750791696309 ) ) ;
#7729=CARTESIAN_POINT ( 'NONE',  ( -8.044165262908093084, -21.95952864787946979, 12.58007249208304046 ) ) ;
#7748=CARTESIAN_POINT ( 'NONE',  ( -18.35725562635144925, -17.85540867095761186, 14.32617750791695599 ) ) ;
#7751=CARTESIAN_POINT ( 'NONE',  ( -15.63902057219073605, -27.04416526290807710, 14.33007249208304223 ) ) ;
#7752=CARTESIAN_POINT ( 'NONE',  ( -22.04416526290807710, -25.71081734191525925, 7.982427507916956877 ) ) ;
#7757=CARTESIAN_POINT ( 'NONE',  ( -14.36097942780923731, -27.04416526290806999, 11.91992750791695954 ) ) ;
#7770=CARTESIAN_POINT ( 'NONE',  ( -10.04416526290807710, -25.50457296725819489, 37.29492750791697375 ) ) ;
#7773=CARTESIAN_POINT ( 'NONE',  ( -19.41254052147348830, -26.35725562635142083, 18.26367750791695599 ) ) ;
#7776=CARTESIAN_POINT ( 'NONE',  ( -12.64274437364858628, -19.58745947852646552, 17.17382249208304401 ) ) ;
#7778=CARTESIAN_POINT ( 'NONE',  ( -13.35725562635141195, -26.51566270880198672, 18.92382249208304401 ) ) ;
#7794=CARTESIAN_POINT ( 'NONE',  ( -10.04416526290807710, -25.50457296725819489, 16.29492750791695954 ) ) ;
#7796=CARTESIAN_POINT ( 'NONE',  ( -9.999999999999994671, -23.83517299489734143, 18.04882249208304401 ) ) ;
#7798=CARTESIAN_POINT ( 'NONE',  ( -16.17491895705301275, -18.95583473709189803, 14.54492750791695421 ) ) ;
#7801=CARTESIAN_POINT ( 'NONE',  ( -20.04416526290808065, -25.17491895705300209, 18.48242750791695599 ) ) ;
#7815=CARTESIAN_POINT ( 'NONE',  ( -21.95583473709189803, -26.04047135212049469, 25.70507249208304046 ) ) ;
#7819=CARTESIAN_POINT ( 'NONE',  ( -10.04416526290808598, -22.49542703274172695, 7.330072492083041347 ) ) ;
#7821=CARTESIAN_POINT ( 'NONE',  ( -17.99999999999999645, -23.83517299489736985, 13.45117750791696309 ) ) ;
#7823=CARTESIAN_POINT ( 'NONE',  ( -8.855408670957602979, -27.35725562635137820, 18.48632249208304046 ) ) ;
#7847=CARTESIAN_POINT ( 'NONE',  ( -18.64274437364853654, -29.97976432393976509, 28.32617750791695954 ) ) ;
#7851=CARTESIAN_POINT ( 'NONE',  ( -16.64274437364858272, -21.48433729119797420, 11.04882249208304223 ) ) ;
#7852=CARTESIAN_POINT ( 'NONE',  ( -22.04416526290807710, -25.71081734191525925, 18.48242750791695954 ) ) ;
#7856=CARTESIAN_POINT ( 'NONE',  ( -12.68318583509884157, -21.92450931948787485, 10.16992750791695954 ) ) ;
#7876=CARTESIAN_POINT ( 'NONE',  ( -12.35725562635143682, -19.75228648362908501, 20.45117750791695954 ) ) ;
#7880=CARTESIAN_POINT ( 'NONE',  ( -18.78091578003892081, -20.46040770435013556, 16.08007249208304401 ) ) ;
#7882=CARTESIAN_POINT ( 'NONE',  ( -13.64274437364857739, -21.31951028609534760, 17.17382249208304401 ) ) ;
#7901=CARTESIAN_POINT ( 'NONE',  ( -9.955834737091912245, -22.82508104294696594, 15.85742750791695777 ) ) ;
#7903=CARTESIAN_POINT ( 'NONE',  ( -19.41254052147350961, -21.64274437364857562, 15.86132249208304223 ) ) ;
#7905=CARTESIAN_POINT ( 'NONE',  ( -13.82508104294698192, -29.04416526290806644, 11.91992750791695421 ) ) ;
#7907=CARTESIAN_POINT ( 'NONE',  ( -10.58745947852649927, -21.64274437364853654, 20.88867750791695954 ) ) ;
#7920=CARTESIAN_POINT ( 'NONE',  ( -20.97976432393974022, -27.64274437364858628, 30.73632249208304046 ) ) ;
#7922=CARTESIAN_POINT ( 'NONE',  ( -18.53959229564983247, -27.78091578003891016, 14.76757249208303868 ) ) ;
#7924=CARTESIAN_POINT ( 'NONE',  ( -17.51566270880201159, -22.35725562635141728, 29.63867750791695954 ) ) ;
#7926=CARTESIAN_POINT ( 'NONE',  ( -21.99999999999999289, -24.16482700510262305, 15.42382249208304046 ) ) ;
#7945=CARTESIAN_POINT ( 'NONE',  ( -18.64274437364853654, -29.97976432393976509, 33.57617750791695954 ) ) ;
#7948=CARTESIAN_POINT ( 'NONE',  ( -17.95583473709190869, -24.96867458239598037, 36.20507249208304756 ) ) ;
#7949=CARTESIAN_POINT ( 'NONE',  ( -21.14459132904236327, -27.35725562635143149, 18.26367750791695599 ) ) ;
#7953=CARTESIAN_POINT ( 'NONE',  ( -14.03132541760401786, -21.04416526290806289, 9.732427507916959541 ) ) ;
#7970=CARTESIAN_POINT ( 'NONE',  ( -19.99999999999999645, -23.83517299489738051, 34.45117750791696665 ) ) ;
#7975=CARTESIAN_POINT ( 'NONE',  ( -9.999999999999994671, -23.83517299489734143, 33.79882249208304046 ) ) ;
#7977=CARTESIAN_POINT ( 'NONE',  ( -17.07549068051208963, -26.31681416490115311, 14.76757249208304223 ) ) ;
#7984=MECHANICAL_DESIGN_GEOMETRIC_PRESENTATION_REPRESENTATION('',(#13598),#6100);
#7987=DIRECTION ( 'NONE',  ( 0.1648270051026194671, 0.000000000000000000, -0.9863224920830413467 ) ) ;
#7995=CARTESIAN_POINT ( 'NONE',  ( -18.53959229564986799, -20.21908421996107563, 19.35742750791695599 ) ) ;
#7998=CARTESIAN_POINT ( 'NONE',  ( -11.21908421996106320, -27.53959229564982181, 18.70507249208304401 ) ) ;
#8000=CARTESIAN_POINT ( 'NONE',  ( -13.49542703274178379, -19.04416526290806289, 9.732427507916959541 ) ) ;
#8002=CARTESIAN_POINT ( 'NONE',  ( -13.82508104294698015, -29.04416526290806289, 11.91992750791695777 ) ) ;
#8004=CARTESIAN_POINT ( 'NONE',  ( -10.75228648362912232, -21.35725562635138530, 28.11132249208304046 ) ) ;
#8016=CARTESIAN_POINT ( 'NONE',  ( -9.996306089212408708, -18.75498260482328661, 33.14257249208303335 ) ) ;
#8018=CARTESIAN_POINT ( 'NONE',  ( -13.49542703274174116, -28.95583473709188738, 8.642572492083040459 ) ) ;
#8020=CARTESIAN_POINT ( 'NONE',  ( -17.31681416490115311, -26.07549068051209318, 28.54492750791696665 ) ) ;
#8022=CARTESIAN_POINT ( 'NONE',  ( -9.754982604823302594, -29.00369391078756465, 13.45507249208303868 ) ) ;
#8027=ORIENTED_EDGE ( 'NONE', *, *, #5333, .F. ) ;
#8042=CARTESIAN_POINT ( 'NONE',  ( -17.04047135212043784, -30.95583473709190159, 28.10742750791695954 ) ) ;
#8046=CARTESIAN_POINT ( 'NONE',  ( -16.64274437364858272, -21.48433729119797420, 37.29882249208304046 ) ) ;
#8047=CARTESIAN_POINT ( 'NONE',  ( -16.71081734191527346, -16.95583473709190159, 19.79492750791695954 ) ) ;
#8052=CARTESIAN_POINT ( 'NONE',  ( -16.35725562635142794, -21.31951028609535470, 30.07617750791696309 ) ) ;
#8071=CARTESIAN_POINT ( 'NONE',  ( -16.50457296725820555, -28.95583473709189448, 28.10742750791695954 ) ) ;
#8074=CARTESIAN_POINT ( 'NONE',  ( -16.50457296725825174, -19.04416526290807354, 37.51757249208304046 ) ) ;
#8075=CARTESIAN_POINT ( 'NONE',  ( -12.31951028609536536, -25.35725562635139596, 34.23632249208304756 ) ) ;
#8091=CARTESIAN_POINT ( 'NONE',  ( -19.41254052147348830, -26.35725562635142083, 28.76367750791695954 ) ) ;
#8093=CARTESIAN_POINT ( 'NONE',  ( -14.83517299489735741, -28.99999999999998224, 19.36132249208304046 ) ) ;
#8095=CARTESIAN_POINT ( 'NONE',  ( -19.24771351637089367, -21.35725562635142438, 19.13867750791695954 ) ) ;
#8097=CARTESIAN_POINT ( 'NONE',  ( -10.75228648362910100, -26.64274437364854009, 32.26367750791695954 ) ) ;
#8099=CARTESIAN_POINT ( 'NONE',  ( -10.58745947852648328, -26.35725562635138530, 18.48632249208304401 ) ) ;
#8109=CARTESIAN_POINT ( 'NONE',  ( -12.95952864787948755, -30.95583473709188382, 34.89257249208303335 ) ) ;
#8110=CARTESIAN_POINT ( 'NONE',  ( -17.64274437364858983, -19.75228648362910633, 5.798822492083041347 ) ) ;
#8111=CARTESIAN_POINT ( 'NONE',  ( -17.51566270880201159, -22.35725562635141728, 34.88867750791696665 ) ) ;
#8113=CARTESIAN_POINT ( 'NONE',  ( -20.00369391078757886, -29.24501739517668142, 20.01757249208303691 ) ) ;
#8131=CARTESIAN_POINT ( 'NONE',  ( -15.16482700510258574, -30.99999999999998224, 33.13867750791695954 ) ) ;
#8136=CARTESIAN_POINT ( 'NONE',  ( -12.48433729119799196, -22.35725562635139596, 38.61132249208304046 ) ) ;
#8137=CARTESIAN_POINT ( 'NONE',  ( -17.04047135212043784, -30.95583473709190159, 12.35742750791695777 ) ) ;
#8143=CARTESIAN_POINT ( 'NONE',  ( -15.16482700510260706, -26.99999999999998579, 27.88867750791696309 ) ) ;
#8156=DIRECTION ( 'NONE',  ( -0.9863224920830415687, -5.704848896154130918E-15, -0.1648270051026189120 ) ) ;
#8160=CARTESIAN_POINT ( 'NONE',  ( -13.82508104294698192, -29.04416526290806644, 27.66992750791695244 ) ) ;
#8164=CARTESIAN_POINT ( 'NONE',  ( -19.41254052147350961, -21.64274437364857562, 26.36132249208304401 ) ) ;
#8167=CARTESIAN_POINT ( 'NONE',  ( -11.99999999999999289, -23.83517299489735564, 33.79882249208304756 ) ) ;
#8189=CARTESIAN_POINT ( 'NONE',  ( -11.21908421996108629, -20.46040770435011069, 25.91992750791694888 ) ) ;
#8192=CARTESIAN_POINT ( 'NONE',  ( -17.64274437364858983, -19.75228648362910633, 37.29882249208303335 ) ) ;
#8195=CARTESIAN_POINT ( 'NONE',  ( -10.04416526290807710, -25.50457296725819489, 37.29492750791697375 ) ) ;
#8198=CARTESIAN_POINT ( 'NONE',  ( -9.999999999999994671, -24.16482700510257686, 31.82617750791696309 ) ) ;
#8200=CARTESIAN_POINT ( 'NONE',  ( -11.21908421996106142, -27.53959229564982181, 23.95507249208304046 ) ) ;
#8213=CARTESIAN_POINT ( 'NONE',  ( -15.96867458239597326, -26.95583473709190159, 22.85742750791695954 ) ) ;
#8216=CARTESIAN_POINT ( 'NONE',  ( -18.64274437364860049, -18.02023567606023491, 32.04882249208304046 ) ) ;
#8232=CARTESIAN_POINT ( 'NONE',  ( -9.754982604823348780, -18.99630608921234654, 36.41992750791695954 ) ) ;
#8233=ORIENTED_EDGE ( 'NONE', *, *, #3894, .T. ) ;
#8236=CARTESIAN_POINT ( 'NONE',  ( -16.64274437364858272, -21.48433729119797420, 26.79882249208304401 ) ) ;
#8237=CARTESIAN_POINT ( 'NONE',  ( -18.64274437364853654, -29.97976432393976509, 17.82617750791695954 ) ) ;
#8242=CARTESIAN_POINT ( 'NONE',  ( -12.68318583509884157, -21.92450931948787485, 31.16992750791695954 ) ) ;
#8257=CARTESIAN_POINT ( 'NONE',  ( -20.04416526290808065, -25.17491895705300209, 28.98242750791695244 ) ) ;
#8261=CARTESIAN_POINT ( 'NONE',  ( -14.83517299489735741, -28.99999999999998224, 35.11132249208304046 ) ) ;
#8263=CARTESIAN_POINT ( 'NONE',  ( -17.51566270880199738, -25.64274437364856496, 30.73632249208304401 ) ) ;
#8276=CARTESIAN_POINT ( 'NONE',  ( -10.75228648362910100, -26.64274437364854009, 32.26367750791695954 ) ) ;
#8278=CARTESIAN_POINT ( 'NONE',  ( -13.82508104294702100, -18.95583473709188382, 37.95507249208304756 ) ) ;
#8281=CARTESIAN_POINT ( 'NONE',  ( -19.95583473709191580, -22.49542703274176603, 24.16992750791694888 ) ) ;
#8283=CARTESIAN_POINT ( 'NONE',  ( -16.50457296725820555, -28.95583473709189803, 33.35742750791695954 ) ) ;
#8285=CARTESIAN_POINT ( 'NONE',  ( -19.95583473709190514, -25.50457296725823042, 30.95507249208304046 ) ) ;
#8296=CARTESIAN_POINT ( 'NONE',  ( -17.95583473709191580, -23.03132541760400898, 39.91992750791695954 ) ) ;
#8298=CARTESIAN_POINT ( 'NONE',  ( -11.35725562635139418, -29.97976432393972601, 39.92382249208304046 ) ) ;
#8314=CARTESIAN_POINT ( 'NONE',  ( -7.999999999999996447, -23.83517299489733432, 2.298822492083038682 ) ) ;
#8321=CARTESIAN_POINT ( 'NONE',  ( -16.35725562635141372, -26.68048971390461332, 35.54882249208304046 ) ) ;
#8322=CARTESIAN_POINT ( 'NONE',  ( -8.044165262908075320, -26.04047135212042718, 26.79492750791695954 ) ) ;
#8343=CARTESIAN_POINT ( 'NONE',  ( -11.21908421996108629, -20.46040770435011069, 31.16992750791695599 ) ) ;
#8346=CARTESIAN_POINT ( 'NONE',  ( -18.78091578003892081, -20.46040770435013556, 31.83007249208304401 ) ) ;
#8351=CARTESIAN_POINT ( 'NONE',  ( -11.95583473709190514, -24.63902057219072361, 28.76757249208304401 ) ) ;
#8360=AXIS2_PLACEMENT_3D ( 'NONE', #10173, #9010, #18045 ) ;
#8368=CARTESIAN_POINT ( 'NONE',  ( -10.58745947852649927, -21.64274437364853654, 31.38867750791696309 ) ) ;
#8370=CARTESIAN_POINT ( 'NONE',  ( -9.955834737091903364, -25.17491895705294880, 28.76757249208304401 ) ) ;
#8374=CARTESIAN_POINT ( 'NONE',  ( -19.99999999999999645, -23.83517299489738051, 29.20117750791695599 ) ) ;
#8376=CARTESIAN_POINT ( 'NONE',  ( -19.24771351637089367, -21.35725562635142438, 29.63867750791695599 ) ) ;
#8377=CARTESIAN_POINT ( 'NONE',  ( -15.16482700510263371, -18.99999999999997868, 21.98632249208304401 ) ) ;
#8385=CARTESIAN_POINT ( 'NONE',  ( -17.68048971390461688, -25.35725562635141372, 39.26367750791696665 ) ) ;
#8387=CARTESIAN_POINT ( 'NONE',  ( -8.044165262908093084, -21.95952864787946979, 33.58007249208304046 ) ) ;
#8402=CARTESIAN_POINT ( 'NONE',  ( -17.04047135212050890, -17.04416526290807710, 6.017572492083039570 ) ) ;
#8407=CARTESIAN_POINT ( 'NONE',  ( -13.64274437364856141, -26.68048971390460622, 1.201177507916959986 ) ) ;
#8408=CARTESIAN_POINT ( 'NONE',  ( -21.95583473709191580, -21.95952864787954084, 29.41992750791695954 ) ) ;
#8430=CARTESIAN_POINT ( 'NONE',  ( -9.020235676060220698, -27.64274437364852588, 6.013677507916956877 ) ) ;
#8433=CARTESIAN_POINT ( 'NONE',  ( -12.04416526290808420, -23.03132541760398766, 7.330072492083044011 ) ) ;
#8440=CARTESIAN_POINT ( 'NONE',  ( -15.96867458239599635, -21.04416526290806999, 27.01757249208303691 ) ) ;
#8452=CARTESIAN_POINT ( 'NONE',  ( -13.49542703274178379, -19.04416526290806289, 25.48242750791694888 ) ) ;
#8455=CARTESIAN_POINT ( 'NONE',  ( -13.49542703274178379, -19.04416526290806289, -0.7675724920830416798 ) ) ;
#8460=CARTESIAN_POINT ( 'NONE',  ( -9.020235676060250896, -20.35725562635137820, 28.11132249208304046 ) ) ;
#8461=CARTESIAN_POINT ( 'NONE',  ( -10.75228648362910100, -26.64274437364854009, 37.51367750791695954 ) ) ;
#8463=CARTESIAN_POINT ( 'NONE',  ( -17.64274437364858983, -19.75228648362910633, 32.04882249208304046 ) ) ;
#8467=CARTESIAN_POINT ( 'NONE',  ( -17.35725562635144215, -19.58745947852648683, 35.32617750791695954 ) ) ;
#8469=CARTESIAN_POINT ( 'NONE',  ( -10.04416526290807710, -25.50457296725819489, 32.04492750791695954 ) ) ;
#8471=CARTESIAN_POINT ( 'NONE',  ( -15.00000000000001421, -18.99999999999997868, -4.336808689942017736E-16 ) ) ;
#8472=CARTESIAN_POINT ( 'NONE',  ( -12.64274437364858628, -19.58745947852646552, 38.17382249208304046 ) ) ;
#8483=CARTESIAN_POINT ( 'NONE',  ( -16.17491895705301275, -18.95583473709189803, 4.044927507916959541 ) ) ;
#8485=CARTESIAN_POINT ( 'NONE',  ( -9.996306089212408708, -18.75498260482328661, 33.14257249208303335 ) ) ;
#8499=CARTESIAN_POINT ( 'NONE',  ( -20.97976432393974022, -27.64274437364858628, 4.486322492083039570 ) ) ;
#8503=CARTESIAN_POINT ( 'NONE',  ( -17.99999999999999645, -23.83517299489736985, 8.201177507916959541 ) ) ;
#8505=CARTESIAN_POINT ( 'NONE',  ( -14.83517299489740715, -16.99999999999997868, 35.76367750791694533 ) ) ;
#8528=CARTESIAN_POINT ( 'NONE',  ( -7.999999999999996447, -24.16482700510256976, 0.3261775079169564884 ) ) ;
#8532=CARTESIAN_POINT ( 'NONE',  ( -15.63902057219073605, -27.04416526290807710, 3.830072492083042679 ) ) ;
#8536=CARTESIAN_POINT ( 'NONE',  ( -12.48433729119798130, -25.64274437364855075, 6.013677507916959541 ) ) ;
#8546=CARTESIAN_POINT ( 'NONE',  ( -19.41254052147348830, -26.35725562635142083, 34.01367750791696665 ) ) ;
#8550=CARTESIAN_POINT ( 'NONE',  ( -9.999999999999994671, -24.16482700510257686, 0.3261775079169582647 ) ) ;
#8553=CARTESIAN_POINT ( 'NONE',  ( -10.75228648362912232, -21.35725562635138530, 1.861322492083040903 ) ) ;
#8554=CARTESIAN_POINT ( 'NONE',  ( -19.95583473709191580, -22.49542703274176603, 39.91992750791695954 ) ) ;
#8556=CARTESIAN_POINT ( 'NONE',  ( -11.46040770435014977, -20.21908421996103655, 27.89257249208303335 ) ) ;
#8559=CARTESIAN_POINT ( 'NONE',  ( -18.78091578003889950, -27.53959229564985378, 33.79492750791696665 ) ) ;
#8563=CARTESIAN_POINT ( 'NONE',  ( -11.46040770435015332, -20.21908421996104011, 33.14257249208303335 ) ) ;
#8575=CARTESIAN_POINT ( 'NONE',  ( -16.50457296725820555, -28.95583473709189448, 7.107427507916955989 ) ) ;
#8577=CARTESIAN_POINT ( 'NONE',  ( -22.04416526290809486, -22.28918265808477628, 36.64257249208304046 ) ) ;
#8579=CARTESIAN_POINT ( 'NONE',  ( -17.99999999999999645, -23.83517299489736985, 34.45117750791695954 ) ) ;
#8580=CARTESIAN_POINT ( 'NONE',  ( -16.50457296725820555, -28.95583473709189803, 7.107427507916956877 ) ) ;
#8592=CARTESIAN_POINT ( 'NONE',  ( -20.97976432393974022, -27.64274437364858628, 9.736322492083036906 ) ) ;
#8596=CARTESIAN_POINT ( 'NONE',  ( -17.68048971390461688, -25.35725562635141372, 2.513677507916959986 ) ) ;
#8597=CARTESIAN_POINT ( 'NONE',  ( -18.35725562635144925, -17.85540867095761186, 35.32617750791695244 ) ) ;
#8620=CARTESIAN_POINT ( 'NONE',  ( -22.04416526290807710, -25.71081734191525925, 2.732427507916957321 ) ) ;
#8623=CARTESIAN_POINT ( 'NONE',  ( -16.50457296725825174, -19.04416526290807354, 42.76757249208303335 ) ) ;
#8626=CARTESIAN_POINT ( 'NONE',  ( -17.68048971390462754, -22.64274437364856496, 42.11132249208304756 ) ) ;
#8639=CARTESIAN_POINT ( 'NONE',  ( -10.58745947852649927, -21.64274437364853654, 26.13867750791695599 ) ) ;
#8641=CARTESIAN_POINT ( 'NONE',  ( -11.21908421996108629, -20.46040770435011069, -0.3300724920830416798 ) ) ;
#8643=CARTESIAN_POINT ( 'NONE',  ( -15.16482700510263371, -18.99999999999997868, 42.98632249208304046 ) ) ;
#8646=CARTESIAN_POINT ( 'NONE',  ( -8.855408670957602979, -27.35725562635137820, 39.48632249208304046 ) ) ;
#8647=CARTESIAN_POINT ( 'NONE',  ( -19.99999999999999645, -23.83517299489738051, 39.70117750791695954 ) ) ;
#8649=CARTESIAN_POINT ( 'NONE',  ( -16.64274437364858272, -21.48433729119797420, 5.798822492083043123 ) ) ;
#8657=CARTESIAN_POINT ( 'NONE',  ( -19.24771351637089367, -21.35725562635142438, 40.13867750791695954 ) ) ;
#8659=CARTESIAN_POINT ( 'NONE',  ( -16.50457296725825174, -19.04416526290807354, 32.26757249208304046 ) ) ;
#8667=CARTESIAN_POINT ( 'NONE',  ( -11.21908421996108629, -20.46040770435011069, 10.16992750791695244 ) ) ;
#8668=CARTESIAN_POINT ( 'NONE',  ( -11.21908421996108629, -20.46040770435011069, -0.3300724920830416798 ) ) ;
#8670=CARTESIAN_POINT ( 'NONE',  ( -14.83517299489735741, -28.99999999999998224, 8.861322492083040459 ) ) ;
#8673=CARTESIAN_POINT ( 'NONE',  ( -12.68318583509884157, -21.92450931948787485, 36.41992750791695954 ) ) ;
#8674=CARTESIAN_POINT ( 'NONE',  ( -13.82508104294698015, -29.04416526290806289, 1.419927507916958209 ) ) ;
#8685=CARTESIAN_POINT ( 'NONE',  ( -20.24501739517669563, -18.99630608921239627, 5.580072492083037794 ) ) ;
#8687=CARTESIAN_POINT ( 'NONE',  ( -10.04416526290808598, -22.49542703274172695, 2.080072492083040903 ) ) ;
#8691=CARTESIAN_POINT ( 'NONE',  ( -12.68318583509884157, -21.92450931948787485, -0.3300724920830400699 ) ) ;
#8692=CARTESIAN_POINT ( 'NONE',  ( -11.35725562635144925, -18.02023567606020293, 25.70117750791695599 ) ) ;
#8710=CARTESIAN_POINT ( 'NONE',  ( -20.97976432393977575, -20.35725562635143504, 3.388677507916956877 ) ) ;
#8715=CARTESIAN_POINT ( 'NONE',  ( -18.53959229564982536, -27.78091578003890660, 41.01757249208304046 ) ) ;
#8718=CARTESIAN_POINT ( 'NONE',  ( -15.63902057219076269, -20.95583473709189448, 4.044927507916962206 ) ) ;
#8729=CARTESIAN_POINT ( 'NONE',  ( -13.82508104294698192, -29.04416526290806644, 32.91992750791695954 ) ) ;
#8735=CARTESIAN_POINT ( 'NONE',  ( -10.04416526290808953, -22.49542703274172695, 2.080072492083040903 ) ) ;
#8737=CARTESIAN_POINT ( 'NONE',  ( -9.754982604823348780, -18.99630608921234654, 10.16992750791695777 ) ) ;
#8742=CARTESIAN_POINT ( 'NONE',  ( -12.04416526290808420, -23.03132541760398766, 2.080072492083043567 ) ) ;
#8746=CARTESIAN_POINT ( 'NONE',  ( -10.20349328142095224, -22.14960319667834909, 2.322403871605816721E-12 ) ) ;
#8752=CARTESIAN_POINT ( 'NONE',  ( -17.35725562635140307, -28.41254052147349185, 40.79882249208304046 ) ) ;
#8764=CARTESIAN_POINT ( 'NONE',  ( -9.955834737091912245, -22.82508104294696594, 0.1074275079169582509 ) ) ;
#8765=CARTESIAN_POINT ( 'NONE',  ( -11.46040770435012668, -27.78091578003887463, 11.48242750791695954 ) ) ;
#8767=CARTESIAN_POINT ( 'NONE',  ( -12.64274437364858628, -19.58745947852646552, 11.92382249208304223 ) ) ;
#8770=CARTESIAN_POINT ( 'NONE',  ( -9.999999999999994671, -24.16482700510257686, 5.576177507916958653 ) ) ;
#8771=CARTESIAN_POINT ( 'NONE',  ( -14.83517299489739649, -18.99999999999997868, 9.513677507916957765 ) ) ;
#8786=CARTESIAN_POINT ( 'NONE',  ( -7.999999999999996447, -23.83517299489733432, 18.04882249208304046 ) ) ;
#8793=CARTESIAN_POINT ( 'NONE',  ( -15.63902057219073605, -27.04416526290807710, 40.58007249208304756 ) ) ;
#8796=CARTESIAN_POINT ( 'NONE',  ( -18.35725562635144925, -17.85540867095761186, 40.57617750791695244 ) ) ;
#8819=CARTESIAN_POINT ( 'NONE',  ( -17.04047135212043784, -30.95583473709190159, 1.857427507916956211 ) ) ;
#8824=CARTESIAN_POINT ( 'NONE',  ( -14.36097942780925685, -20.95583473709189093, 6.455072492083044899 ) ) ;
#8828=CARTESIAN_POINT ( 'NONE',  ( -12.68318583509884157, -21.92450931948787485, 4.919927507916961318 ) ) ;
#8838=CARTESIAN_POINT ( 'NONE',  ( -19.95583473709191580, -22.49542703274176603, 29.41992750791695599 ) ) ;
#8844=CARTESIAN_POINT ( 'NONE',  ( -9.955834737091903364, -25.17491895705294880, 2.517572492083040903 ) ) ;
#8845=CARTESIAN_POINT ( 'NONE',  ( -17.35725562635144215, -19.58745947852648683, 40.57617750791696665 ) ) ;
#8847=CARTESIAN_POINT ( 'NONE',  ( -14.03132541760400009, -26.95583473709189448, 8.642572492083042235 ) ) ;
#8865=CARTESIAN_POINT ( 'NONE',  ( -19.41254052147348830, -26.35725562635142083, 7.763677507916958653 ) ) ;
#8866=CARTESIAN_POINT ( 'NONE',  ( -19.95583473709191580, -22.49542703274176603, 18.91992750791694888 ) ) ;
#8868=CARTESIAN_POINT ( 'NONE',  ( -12.35725562635140307, -28.24771351637085459, 8.423822492083042235 ) ) ;
#8870=CARTESIAN_POINT ( 'NONE',  ( -19.24771351637089367, -21.35725562635142438, 8.638677507916957765 ) ) ;
#8872=CARTESIAN_POINT ( 'NONE',  ( -12.64274437364855252, -28.41254052147347053, 6.451177507916959541 ) ) ;
#8883=CARTESIAN_POINT ( 'NONE',  ( -9.754982604823302594, -29.00369391078756465, 23.95507249208304046 ) ) ;
#8884=SURFACE_STYLE_FILL_AREA ( #1544 ) ;
#8888=CARTESIAN_POINT ( 'NONE',  ( -12.68318583509884157, -21.92450931948787485, 15.41992750791695954 ) ) ;
#8890=CARTESIAN_POINT ( 'NONE',  ( -21.95583473709191580, -21.95952864787954084, 39.91992750791695954 ) ) ;
#8910=CARTESIAN_POINT ( 'NONE',  ( -9.020235676060220698, -27.64274437364852588, 21.76367750791695954 ) ) ;
#8915=CARTESIAN_POINT ( 'NONE',  ( -12.48433729119799196, -22.35725562635139596, 22.86132249208304401 ) ) ;
#8919=CARTESIAN_POINT ( 'NONE',  ( -18.04416526290808420, -24.63902057219074493, 7.982427507916962206 ) ) ;
#8933=CARTESIAN_POINT ( 'NONE',  ( -17.35725562635144215, -19.58745947852648683, 19.57617750791695954 ) ) ;
#8936=CARTESIAN_POINT ( 'NONE',  ( -15.16482700510263371, -18.99999999999997868, 0.9863224920830410136 ) ) ;
#8941=CARTESIAN_POINT ( 'NONE',  ( -14.03132541760400009, -26.95583473709189448, 3.392572492083043567 ) ) ;
#8956=PRESENTATION_STYLE_ASSIGNMENT (( #2975 ) ) ;
#8961=CARTESIAN_POINT ( 'NONE',  ( -19.99999999999999645, -23.83517299489738051, 8.201177507916957765 ) ) ;
#8962=CARTESIAN_POINT ( 'NONE',  ( -10.58745947852649927, -21.64274437364853654, 15.63867750791695777 ) ) ;
#8964=CARTESIAN_POINT ( 'NONE',  ( -20.00369391078757886, -29.24501739517668142, 41.01757249208304046 ) ) ;
#8968=CARTESIAN_POINT ( 'NONE',  ( -18.04416526290808420, -24.63902057219074493, 39.48242750791696665 ) ) ;
#8970=CARTESIAN_POINT ( 'NONE',  ( -9.999999999999994671, -24.16482700510257686, 5.576177507916958653 ) ) ;
#8982=CARTESIAN_POINT ( 'NONE',  ( -9.754982604823302594, -29.00369391078756465, 18.70507249208304046 ) ) ;
#8987=CARTESIAN_POINT ( 'NONE',  ( -14.83517299489738761, -20.99999999999997513, 9.513677507916957765 ) ) ;
#8989=CARTESIAN_POINT ( 'NONE',  ( -21.99999999999999289, -23.83517299489739116, 39.70117750791695954 ) ) ;
#9009=CARTESIAN_POINT ( 'NONE',  ( -21.95583473709191580, -21.95952864787954084, 13.66992750791695954 ) ) ;
#9010=DIRECTION ( 'NONE',  ( -0.9863224920830415687, -6.131453374264637327E-15, -0.1648270051026182181 ) ) ;
#9013=CARTESIAN_POINT ( 'NONE',  ( -12.48433729119799196, -22.35725562635139596, 17.61132249208304401 ) ) ;
#9018=CARTESIAN_POINT ( 'NONE',  ( -11.99999999999999289, -24.16482700510258752, 10.82617750791695954 ) ) ;
#9030=CARTESIAN_POINT ( 'NONE',  ( -19.99999999999999645, -23.83517299489738051, 34.45117750791696665 ) ) ;
#9031=FACE_OUTER_BOUND ( 'NONE', #11346, .T. ) ;
#9032=CARTESIAN_POINT ( 'NONE',  ( -19.41254052147348830, -26.35725562635142083, 23.51367750791695954 ) ) ;
#9038=CARTESIAN_POINT ( 'NONE',  ( -12.35725562635140307, -28.24771351637085459, 24.17382249208304046 ) ) ;
#9042=CARTESIAN_POINT ( 'NONE',  ( -12.48433729119799196, -22.35725562635139596, 1.861322492083043123 ) ) ;
#9043=CIRCLE ( 'NONE', #19062, 1.000000000000000000 ) ;
#9046=CARTESIAN_POINT ( 'NONE',  ( -14.69695850531174131, -17.99999999999998934, -4.336808689941901379E-16 ) ) ;
#9061=CARTESIAN_POINT ( 'NONE',  ( -19.24771351637089367, -21.35725562635142438, 19.13867750791695954 ) ) ;
#9062=CARTESIAN_POINT ( 'NONE',  ( -11.21908421996108629, -20.46040770435011069, 10.16992750791695244 ) ) ;
#9064=CARTESIAN_POINT ( 'NONE',  ( -22.04416526290809486, -22.28918265808477628, 41.89257249208304046 ) ) ;
#9067=CARTESIAN_POINT ( 'NONE',  ( -13.49542703274178379, -19.04416526290806289, -0.7675724920830416798 ) ) ;
#9070=CARTESIAN_POINT ( 'NONE',  ( -10.04416526290807710, -25.50457296725819489, 21.54492750791695599 ) ) ;
#9085=CARTESIAN_POINT ( 'NONE',  ( -18.64274437364860049, -18.02023567606023491, 16.29882249208303691 ) ) ;
#9086=CARTESIAN_POINT ( 'NONE',  ( -11.21908421996106142, -27.53959229564982181, 2.955072492083040903 ) ) ;
#9089=CARTESIAN_POINT ( 'NONE',  ( -17.51566270880201159, -22.35725562635141728, 8.638677507916959541 ) ) ;
#9091=CARTESIAN_POINT ( 'NONE',  ( -9.996306089212408708, -18.75498260482328661, 6.892572492083038682 ) ) ;
#9101=CARTESIAN_POINT ( 'NONE',  ( -12.64915539091913566, -20.59698958850244210, -1.847635612036354826E-16 ) ) ;
#9109=CARTESIAN_POINT ( 'NONE',  ( -17.04047135212043784, -30.95583473709190159, 12.35742750791695777 ) ) ;
#9114=CARTESIAN_POINT ( 'NONE',  ( -12.68318583509882380, -26.07549068051207541, 18.70507249208304401 ) ) ;
#9119=CARTESIAN_POINT ( 'NONE',  ( -18.04416526290808420, -24.63902057219074493, 13.23242750791696132 ) ) ;
#9138=CARTESIAN_POINT ( 'NONE',  ( -13.82508104294698192, -29.04416526290806644, 17.16992750791694888 ) ) ;
#9141=CARTESIAN_POINT ( 'NONE',  ( -14.83517299489735741, -28.99999999999998224, 14.11132249208304046 ) ) ;
#9143=CARTESIAN_POINT ( 'NONE',  ( -17.31681416490117087, -21.92450931948788551, 16.08007249208304401 ) ) ;
#9161=CARTESIAN_POINT ( 'NONE',  ( -11.21908421996108629, -20.46040770435011069, 15.41992750791695954 ) ) ;
#9162=CARTESIAN_POINT ( 'NONE',  ( -9.955834737091912245, -22.82508104294696594, 10.60742750791695777 ) ) ;
#9164=CARTESIAN_POINT ( 'NONE',  ( -10.75228648362912232, -21.35725562635138530, 22.86132249208304401 ) ) ;
#9167=CARTESIAN_POINT ( 'NONE',  ( -15.96867458239597326, -26.95583473709190159, 38.60742750791696665 ) ) ;
#9170=CARTESIAN_POINT ( 'NONE',  ( -17.35725562635144215, -19.58745947852648683, 14.32617750791695777 ) ) ;
#9183=CARTESIAN_POINT ( 'NONE',  ( -9.996306089212408708, -18.75498260482328661, 17.39257249208304046 ) ) ;
#9184=CARTESIAN_POINT ( 'NONE',  ( -12.35725562635140307, -28.24771351637085459, 8.423822492083042235 ) ) ;
#9187=CARTESIAN_POINT ( 'NONE',  ( -14.03132541760401786, -21.04416526290806289, 20.23242750791696309 ) ) ;
#9189=CARTESIAN_POINT ( 'NONE',  ( -20.24501739517669563, -18.99630608921239627, 10.83007249208304046 ) ) ;
#9206=CARTESIAN_POINT ( 'NONE',  ( -21.14459132904236327, -27.35725562635143149, 18.26367750791695599 ) ) ;
#9209=CARTESIAN_POINT ( 'NONE',  ( -12.92450931948790149, -21.68318583509881137, 12.14257249208304223 ) ) ;
#9210=CARTESIAN_POINT ( 'NONE',  ( -19.24771351637089367, -21.35725562635142438, 40.13867750791695954 ) ) ;
#9215=CARTESIAN_POINT ( 'NONE',  ( -12.48433729119798130, -25.64274437364855075, 21.76367750791695954 ) ) ;
#9227=CARTESIAN_POINT ( 'NONE',  ( -13.82508104294698192, -29.04416526290806644, 38.16992750791695244 ) ) ;
#9231=CARTESIAN_POINT ( 'NONE',  ( -10.58745947852649927, -21.64274437364853654, 10.38867750791695777 ) ) ;
#9234=CARTESIAN_POINT ( 'NONE',  ( -12.64274437364858628, -19.58745947852646552, 11.92382249208304223 ) ) ;
#9236=CARTESIAN_POINT ( 'NONE',  ( -12.68318583509882380, -26.07549068051207541, 18.70507249208304401 ) ) ;
#9255=CARTESIAN_POINT ( 'NONE',  ( -10.04416526290807710, -25.50457296725819489, 11.04492750791695421 ) ) ;
#9259=CARTESIAN_POINT ( 'NONE',  ( -13.82508104294702100, -18.95583473709188382, 16.95507249208304046 ) ) ;
#9261=CARTESIAN_POINT ( 'NONE',  ( -10.75228648362910100, -26.64274437364854009, 21.76367750791695599 ) ) ;
#9264=CARTESIAN_POINT ( 'NONE',  ( -19.99999999999999645, -23.83517299489738051, 13.45117750791695777 ) ) ;
#9276=CARTESIAN_POINT ( 'NONE',  ( -22.04416526290809486, -22.28918265808477628, 36.64257249208304046 ) ) ;
#9279=CARTESIAN_POINT ( 'NONE',  ( -19.41254052147350961, -21.64274437364857562, 10.61132249208304046 ) ) ;
#9282=CARTESIAN_POINT ( 'NONE',  ( -15.16482700510260706, -26.99999999999998579, 12.13867750791695954 ) ) ;
#9284=CARTESIAN_POINT ( 'NONE',  ( -13.28918265808478694, -16.95583473709189093, 22.20507249208304046 ) ) ;
#9303=CARTESIAN_POINT ( 'NONE',  ( -9.754982604823348780, -18.99630608921234654, 20.66992750791695954 ) ) ;
#9307=CARTESIAN_POINT ( 'NONE',  ( -12.31951028609536536, -25.35725562635139596, 18.48632249208304401 ) ) ;
#9308=CARTESIAN_POINT ( 'NONE',  ( -15.16482700510258574, -30.99999999999998224, 12.13867750791695421 ) ) ;
#9312=CARTESIAN_POINT ( 'NONE',  ( -17.51566270880201159, -22.35725562635141728, 19.13867750791695954 ) ) ;
#9326=CARTESIAN_POINT ( 'NONE',  ( -18.53959229564986799, -20.21908421996107563, 14.10742750791695777 ) ) ;
#9329=CARTESIAN_POINT ( 'NONE',  ( -16.17491895705296656, -29.04416526290807710, 19.58007249208303335 ) ) ;
#9330=CARTESIAN_POINT ( 'NONE',  ( -12.68318583509882380, -26.07549068051207541, 13.45507249208304401 ) ) ;
#9346=CARTESIAN_POINT ( 'NONE',  ( -18.78091578003889950, -27.53959229564985378, 12.79492750791695421 ) ) ;
#9349=CARTESIAN_POINT ( 'NONE',  ( -12.35725562635140307, -28.24771351637085459, 24.17382249208304046 ) ) ;
#9351=CARTESIAN_POINT ( 'NONE',  ( -14.83517299489739649, -18.99999999999997868, 9.513677507916957765 ) ) ;
#9355=CARTESIAN_POINT ( 'NONE',  ( -13.49542703274178201, -19.04416526290806289, 20.23242750791695954 ) ) ;
#9367=CARTESIAN_POINT ( 'NONE',  ( -8.044165262908093084, -21.95952864787946979, 38.83007249208303335 ) ) ;
#9370=CARTESIAN_POINT ( 'NONE',  ( -12.64274437364858628, -19.58745947852646552, 11.92382249208304223 ) ) ;
#9372=CARTESIAN_POINT ( 'NONE',  ( -11.99999999999999289, -24.16482700510258752, 26.57617750791696309 ) ) ;
#9374=CARTESIAN_POINT ( 'NONE',  ( -8.855408670957602979, -27.35725562635137820, 23.73632249208303691 ) ) ;
#9396=CARTESIAN_POINT ( 'NONE',  ( -13.28918265808472299, -31.04416526290805933, 32.91992750791695244 ) ) ;
#9400=CARTESIAN_POINT ( 'NONE',  ( -11.99999999999999289, -23.83517299489735564, 33.79882249208304756 ) ) ;
#9401=CARTESIAN_POINT ( 'NONE',  ( -21.95583473709191580, -21.95952864787954084, 18.91992750791695954 ) ) ;
#9406=CARTESIAN_POINT ( 'NONE',  ( -15.96867458239597326, -26.95583473709190159, 12.35742750791696132 ) ) ;
#9427=CARTESIAN_POINT ( 'NONE',  ( -18.53959229564986799, -20.21908421996107563, 24.60742750791695954 ) ) ;
#9432=CARTESIAN_POINT ( 'NONE',  ( -17.35725562635140307, -28.41254052147349185, 14.54882249208304046 ) ) ;
#9434=CARTESIAN_POINT ( 'NONE',  ( -13.64274437364857739, -21.31951028609534760, 22.42382249208304401 ) ) ;
#9452=CARTESIAN_POINT ( 'NONE',  ( -14.83517299489739649, -18.99999999999997868, 20.01367750791695954 ) ) ;
#9454=CARTESIAN_POINT ( 'NONE',  ( -10.58745947852648328, -26.35725562635138530, 18.48632249208304401 ) ) ;
#9458=CARTESIAN_POINT ( 'NONE',  ( -16.17491895705301275, -18.95583473709189803, 19.79492750791695954 ) ) ;
#9459=CARTESIAN_POINT ( 'NONE',  ( -14.83517299489739649, -18.99999999999997868, 41.01367750791696665 ) ) ;
#9460=CARTESIAN_POINT ( 'NONE',  ( -18.53959229564986799, -20.21908421996107563, 14.10742750791695777 ) ) ;
#9462=CARTESIAN_POINT ( 'NONE',  ( -10.58745947852648328, -26.35725562635138530, 23.73632249208304046 ) ) ;
#9471=CARTESIAN_POINT ( 'NONE',  ( -21.14459132904239169, -20.64274437364858628, 36.86132249208304046 ) ) ;
#9472=CARTESIAN_POINT ( 'NONE',  ( -11.46040770435015332, -20.21908421996104011, 6.892572492083040459 ) ) ;
#9474=CARTESIAN_POINT ( 'NONE',  ( -17.31681416490115311, -26.07549068051209318, 23.29492750791696309 ) ) ;
#9477=CARTESIAN_POINT ( 'NONE',  ( -7.999999999999996447, -23.83517299489733432, 12.79882249208303691 ) ) ;
#9492=CARTESIAN_POINT ( 'NONE',  ( -21.95583473709191580, -21.95952864787954084, 34.66992750791696665 ) ) ;
#9496=CARTESIAN_POINT ( 'NONE',  ( -17.68048971390462754, -22.64274437364856496, 36.86132249208304046 ) ) ;
#9497=CARTESIAN_POINT ( 'NONE',  ( -20.97976432393977575, -20.35725562635143504, 13.88867750791695599 ) ) ;
#9504=CARTESIAN_POINT ( 'NONE',  ( -13.35725562635142794, -21.48433729119796709, 30.95117750791695954 ) ) ;
#9520=CARTESIAN_POINT ( 'NONE',  ( -10.04416526290807710, -25.50457296725819489, 37.29492750791697375 ) ) ;
#9524=CARTESIAN_POINT ( 'NONE',  ( -12.35725562635140307, -28.24771351637085459, 29.42382249208304401 ) ) ;
#9526=CARTESIAN_POINT ( 'NONE',  ( -12.48433729119799196, -22.35725562635139596, 22.86132249208304401 ) ) ;
#9543=CARTESIAN_POINT ( 'NONE',  ( -16.50457296725820555, -28.95583473709189448, 38.60742750791694533 ) ) ;
#9546=CARTESIAN_POINT ( 'NONE',  ( -9.999999999999994671, -23.83517299489734143, 12.79882249208304046 ) ) ;
#9549=CARTESIAN_POINT ( 'NONE',  ( -9.999999999999994671, -24.16482700510257686, 21.32617750791695599 ) ) ;
#9551=CARTESIAN_POINT ( 'NONE',  ( -17.64274437364855430, -28.24771351637087236, 28.32617750791695954 ) ) ;
#9553=CARTESIAN_POINT ( 'NONE',  ( -12.64274437364858628, -19.58745947852646552, 27.67382249208304046 ) ) ;
#9562=CARTESIAN_POINT ( 'NONE',  ( -9.020235676060250896, -20.35725562635137820, 33.36132249208304046 ) ) ;
#9563=CARTESIAN_POINT ( 'NONE',  ( -11.46040770435015332, -20.21908421996104011, 17.39257249208304401 ) ) ;
#9564=CARTESIAN_POINT ( 'NONE',  ( -15.96867458239597326, -26.95583473709190159, 33.35742750791695954 ) ) ;
#9566=CARTESIAN_POINT ( 'NONE',  ( -18.35725562635138886, -30.14459132904237393, 14.54882249208303868 ) ) ;
#9584=CARTESIAN_POINT ( 'NONE',  ( -21.14459132904236327, -27.35725562635143149, 23.51367750791695599 ) ) ;
#9589=CARTESIAN_POINT ( 'NONE',  ( -13.64274437364857739, -21.31951028609534760, 38.17382249208304046 ) ) ;
#9592=CARTESIAN_POINT ( 'NONE',  ( -7.999999999999996447, -24.16482700510256976, 10.82617750791695599 ) ) ;
#9597=CARTESIAN_POINT ( 'NONE',  ( -16.35725562635142794, -21.31951028609535470, 24.82617750791696309 ) ) ;
#9616=CARTESIAN_POINT ( 'NONE',  ( -11.21908421996108629, -20.46040770435011069, 25.91992750791694888 ) ) ;
#9620=CARTESIAN_POINT ( 'NONE',  ( -10.75228648362912232, -21.35725562635138530, 28.11132249208304046 ) ) ;
#9622=CARTESIAN_POINT ( 'NONE',  ( -12.68318583509882380, -26.07549068051207541, 39.70507249208305467 ) ) ;
#9637=UNCERTAINTY_MEASURE_WITH_UNIT (LENGTH_MEASURE( 1.000000000000000082E-05 ), #16512, 'distance_accuracy_value', 'NONE');
#9640=CARTESIAN_POINT ( 'NONE',  ( -16.17491895705301275, -18.95583473709189803, 25.04492750791695954 ) ) ;
#9642=CARTESIAN_POINT ( 'NONE',  ( -18.78091578003892081, -20.46040770435013556, 31.83007249208304401 ) ) ;
#9644=CARTESIAN_POINT ( 'NONE',  ( -19.41254052147348830, -26.35725562635142083, 13.01367750791695777 ) ) ;
#9646=CARTESIAN_POINT ( 'NONE',  ( -10.75228648362910100, -26.64274437364854009, 37.51367750791695954 ) ) ;
#9648=CARTESIAN_POINT ( 'NONE',  ( -20.04416526290809131, -22.82508104294700502, 20.89257249208304046 ) ) ;
#9657=CARTESIAN_POINT ( 'NONE',  ( -14.83517299489734853, -30.99999999999998224, 29.86132249208304046 ) ) ;
#9659=CARTESIAN_POINT ( 'NONE',  ( -14.83517299489738761, -20.99999999999997513, 25.26367750791696309 ) ) ;
#9662=CARTESIAN_POINT ( 'NONE',  ( -21.99999999999999289, -24.16482700510262305, 36.42382249208304756 ) ) ;
#9679=CARTESIAN_POINT ( 'NONE',  ( -16.71081734191527346, -16.95583473709190159, 25.04492750791695599 ) ) ;
#9685=CARTESIAN_POINT ( 'NONE',  ( -17.68048971390462754, -22.64274437364856496, 26.36132249208304401 ) ) ;
#9686=CARTESIAN_POINT ( 'NONE',  ( -11.64274437364854187, -30.14459132904234195, 16.95117750791695954 ) ) ;
#9691=CARTESIAN_POINT ( 'NONE',  ( -13.35725562635142794, -21.48433729119796709, 25.70117750791695954 ) ) ;
#9709=CARTESIAN_POINT ( 'NONE',  ( -17.64274437364855430, -28.24771351637087236, 28.32617750791695954 ) ) ;
#9713=CARTESIAN_POINT ( 'NONE',  ( -13.82508104294702100, -18.95583473709188382, 32.70507249208304046 ) ) ;
#9717=CARTESIAN_POINT ( 'NONE',  ( -16.35725562635141372, -26.68048971390461332, 35.54882249208304046 ) ) ;
#9731=AXIS2_PLACEMENT_3D ( 'NONE', #14814, #17651, #11754 ) ;
#9734=CARTESIAN_POINT ( 'NONE',  ( -17.35725562635144215, -19.58745947852648683, 30.07617750791695599 ) ) ;
#9736=CARTESIAN_POINT ( 'NONE',  ( -12.64274437364858628, -19.58745947852646552, 38.17382249208304046 ) ) ;
#9741=CARTESIAN_POINT ( 'NONE',  ( -16.50457296725820555, -28.95583473709189448, 33.35742750791695954 ) ) ;
#9745=CARTESIAN_POINT ( 'NONE',  ( -16.50457296725820555, -28.95583473709189803, 38.60742750791695954 ) ) ;
#9747=CARTESIAN_POINT ( 'NONE',  ( -13.49542703274174116, -28.95583473709188738, 24.39257249208304046 ) ) ;
#9757=CARTESIAN_POINT ( 'NONE',  ( -15.63902057219076269, -20.95583473709189448, 35.54492750791696665 ) ) ;
#9759=CARTESIAN_POINT ( 'NONE',  ( -13.28918265808478694, -16.95583473709189093, 32.70507249208304756 ) ) ;
#9773=CARTESIAN_POINT ( 'NONE',  ( -7.955834737091916686, -22.28918265808470522, 36.85742750791695244 ) ) ;
#9779=CARTESIAN_POINT ( 'NONE',  ( -14.03132541760400009, -26.95583473709189448, 34.89257249208305467 ) ) ;
#9780=CARTESIAN_POINT ( 'NONE',  ( -15.16482700510258574, -30.99999999999998224, 33.13867750791695954 ) ) ;
#9800=CARTESIAN_POINT ( 'NONE',  ( -14.83517299489739649, -18.99999999999997868, 25.26367750791695599 ) ) ;
#9804=CARTESIAN_POINT ( 'NONE',  ( -19.99999999999999645, -24.16482700510261949, 36.42382249208304046 ) ) ;
#9806=CARTESIAN_POINT ( 'NONE',  ( -12.48433729119799196, -22.35725562635139596, 28.11132249208304401 ) ) ;
#9820=CARTESIAN_POINT ( 'NONE',  ( -15.16482700510259640, -28.99999999999998224, 33.13867750791696665 ) ) ;
#9824=CARTESIAN_POINT ( 'NONE',  ( -10.04416526290808953, -22.49542703274172695, 33.58007249208304046 ) ) ;
#9827=CARTESIAN_POINT ( 'NONE',  ( -19.95583473709191580, -22.49542703274176603, 34.66992750791694533 ) ) ;
#9830=CARTESIAN_POINT ( 'NONE',  ( -19.24771351637089367, -21.35725562635142438, 34.88867750791696665 ) ) ;
#9832=CARTESIAN_POINT ( 'NONE',  ( -10.04416526290808598, -22.49542703274172695, 23.08007249208303691 ) ) ;
#9843=CARTESIAN_POINT ( 'NONE',  ( -17.31681416490115311, -26.07549068051209318, 39.04492750791695954 ) ) ;
#9845=CARTESIAN_POINT ( 'NONE',  ( -16.71081734191520596, -31.04416526290808065, 30.08007249208304046 ) ) ;
#9862=CARTESIAN_POINT ( 'NONE',  ( -21.14459132904236327, -27.35725562635143149, 39.26367750791695244 ) ) ;
#9869=CARTESIAN_POINT ( 'NONE',  ( -14.83517299489738761, -20.99999999999997513, 4.263677507916960430 ) ) ;
#9871=CARTESIAN_POINT ( 'NONE',  ( -9.020235676060220698, -27.64274437364852588, 27.01367750791695599 ) ) ;
#9892=CARTESIAN_POINT ( 'NONE',  ( -22.04416526290807710, -25.71081734191525925, 7.982427507916956877 ) ) ;
#9895=CARTESIAN_POINT ( 'NONE',  ( -16.17491895705296656, -29.04416526290807710, 30.08007249208304401 ) ) ;
#9900=CARTESIAN_POINT ( 'NONE',  ( -15.16482700510262482, -20.99999999999997513, 27.23632249208304046 ) ) ;
#9908=CARTESIAN_POINT ( 'NONE',  ( -16.50457296725820555, -28.95583473709189448, 33.35742750791695954 ) ) ;
#9911=CARTESIAN_POINT ( 'NONE',  ( -17.64274437364855430, -28.24771351637087236, 7.326177507916957765 ) ) ;
#9914=CARTESIAN_POINT ( 'NONE',  ( -9.955834737091912245, -22.82508104294696594, 36.85742750791696665 ) ) ;
#9916=CARTESIAN_POINT ( 'NONE',  ( -18.53959229564982536, -27.78091578003890660, 30.51757249208304401 ) ) ;
#9919=CARTESIAN_POINT ( 'NONE',  ( -15.16482700510259640, -28.99999999999998224, 33.13867750791696665 ) ) ;
#9921=CARTESIAN_POINT ( 'NONE',  ( -17.64274437364855430, -28.24771351637087236, 33.57617750791696665 ) ) ;
#9923=CARTESIAN_POINT ( 'NONE',  ( -16.50457296725825174, -19.04416526290807354, 42.76757249208303335 ) ) ;
#9933=CARTESIAN_POINT ( 'NONE',  ( -14.36097942780923731, -27.04416526290806999, 38.16992750791696665 ) ) ;
#9936=CARTESIAN_POINT ( 'NONE',  ( -9.996306089212408708, -18.75498260482328661, 27.89257249208303691 ) ) ;
#9950=CARTESIAN_POINT ( 'NONE',  ( -7.955834737091903364, -25.71081734191518464, 2.517572492083039126 ) ) ;
#9955=CARTESIAN_POINT ( 'NONE',  ( -16.64274437364856496, -26.51566270880199738, 7.326177507916959541 ) ) ;
#9956=CARTESIAN_POINT ( 'NONE',  ( -20.24501739517664234, -29.00369391078761439, 28.54492750791695954 ) ) ;
#9966=LINE ( 'NONE', #11250, #16275 ) ;
#9979=CARTESIAN_POINT ( 'NONE',  ( -8.044165262908075320, -26.04047135212042718, 0.5449275079169564329 ) ) ;
#9982=CARTESIAN_POINT ( 'NONE',  ( -17.07549068051208963, -26.31681416490115311, 9.517572492083044011 ) ) ;
#9987=CARTESIAN_POINT ( 'NONE',  ( -17.07549068051210739, -21.68318583509881847, 8.857427507916959541 ) ) ;
#10000=CARTESIAN_POINT ( 'NONE',  ( -20.04416526290808065, -25.17491895705300209, 28.98242750791695244 ) ) ;
#10003=CARTESIAN_POINT ( 'NONE',  ( -19.24771351637089367, -21.35725562635142438, 3.388677507916958653 ) ) ;
#10007=CARTESIAN_POINT ( 'NONE',  ( -15.16482700510264436, -16.99999999999997868, 42.98632249208304756 ) ) ;
#10008=CARTESIAN_POINT ( 'NONE',  ( -8.855408670957631401, -20.64274437364852943, 5.138677507916955989 ) ) ;
#10012=CARTESIAN_POINT ( 'NONE',  ( -19.24771351637086880, -26.64274437364857206, 35.98632249208304046 ) ) ;
#10017=CARTESIAN_POINT ( 'NONE',  ( -10.75228648362910100, -26.64274437364854009, 32.26367750791695954 ) ) ;
#10022=CARTESIAN_POINT ( 'NONE',  ( -13.49542703274174116, -28.95583473709188738, 40.14257249208304046 ) ) ;
#10036=CARTESIAN_POINT ( 'NONE',  ( -10.04416526290807710, -25.50457296725819489, 0.5449275079169579872 ) ) ;
#10038=CARTESIAN_POINT ( 'NONE',  ( -18.64274437364860049, -18.02023567606023491, 37.29882249208304046 ) ) ;
#10041=CARTESIAN_POINT ( 'NONE',  ( -12.31951028609537602, -22.64274437364854364, 26.13867750791696309 ) ) ;
#10042=CARTESIAN_POINT ( 'NONE',  ( -19.95583473709191225, -22.49542703274176603, 3.169927507916957765 ) ) ;
#10052=CARTESIAN_POINT ( 'NONE',  ( -21.95583473709189803, -26.04047135212049469, 4.705072492083038682 ) ) ;
#10057=CARTESIAN_POINT ( 'NONE',  ( -17.99999999999999645, -24.16482700510260173, 41.67382249208304756 ) ) ;
#10058=CARTESIAN_POINT ( 'NONE',  ( -9.996306089212364299, -29.24501739517662813, 32.48242750791695244 ) ) ;
#10079=CARTESIAN_POINT ( 'NONE',  ( -13.28918265808472299, -31.04416526290805933, 1.419927507916956433 ) ) ;
#10083=CARTESIAN_POINT ( 'NONE',  ( -10.58745947852648328, -26.35725562635138530, 39.48632249208304046 ) ) ;
#10087=CARTESIAN_POINT ( 'NONE',  ( -18.04416526290808420, -24.63902057219074493, 2.732427507916960430 ) ) ;
#10097=CARTESIAN_POINT ( 'NONE',  ( -19.41254052147348830, -26.35725562635142083, 23.51367750791695954 ) ) ;
#10099=CARTESIAN_POINT ( 'NONE',  ( -11.46040770435012668, -27.78091578003887463, 6.232427507916956877 ) ) ;
#10103=CARTESIAN_POINT ( 'NONE',  ( -19.41254052147350961, -21.64274437364857562, 10.61132249208304046 ) ) ;
#10104=CARTESIAN_POINT ( 'NONE',  ( -12.95952864787955150, -17.04416526290805933, 4.482427507916956877 ) ) ;
#10107=CARTESIAN_POINT ( 'NONE',  ( -11.95583473709190514, -24.63902057219072361, 7.767572492083043123 ) ) ;
#10111=CARTESIAN_POINT ( 'NONE',  ( -9.955834737091912245, -22.82508104294696594, 36.85742750791696665 ) ) ;
#10115=CARTESIAN_POINT ( 'NONE',  ( -10.04416526290808598, -22.49542703274172695, 33.58007249208303335 ) ) ;
#10126=CARTESIAN_POINT ( 'NONE',  ( -12.92450931948788906, -26.31681416490114245, 37.73242750791696665 ) ) ;
#10128=CARTESIAN_POINT ( 'NONE',  ( -20.04416526290809131, -22.82508104294699791, 5.142572492083038682 ) ) ;
#10131=CARTESIAN_POINT ( 'NONE',  ( -18.04416526290808420, -24.63902057219074493, 34.23242750791695954 ) ) ;
#10143=CARTESIAN_POINT ( 'NONE',  ( -17.04047135212043784, -30.95583473709190159, 38.60742750791695954 ) ) ;
#10147=CARTESIAN_POINT ( 'NONE',  ( -18.04416526290808420, -24.63902057219074493, 2.732427507916960430 ) ) ;
#10148=CARTESIAN_POINT ( 'NONE',  ( -14.83517299489740715, -16.99999999999997868, 30.51367750791695954 ) ) ;
#10149=PRODUCT_DEFINITION_FORMATION_WITH_SPECIFIED_SOURCE ( 'ANY', '', #18808, .NOT_KNOWN. ) ;
#10150=AXIS2_PLACEMENT_3D ( 'NONE', #16879, #2072, #10779 ) ;
#10171=CARTESIAN_POINT ( 'NONE',  ( -9.996306089212364299, -29.24501739517662813, 6.232427507916955989 ) ) ;
#10173=CARTESIAN_POINT ( 'NONE',  ( -15.16482700510263371, -18.99999999999997868, 0.9863224920830410136 ) ) ;
#10176=CARTESIAN_POINT ( 'NONE',  ( -17.35725562635140307, -28.41254052147349185, 40.79882249208304046 ) ) ;
#10180=CARTESIAN_POINT ( 'NONE',  ( -17.07549068051208963, -26.31681416490115311, 41.01757249208304756 ) ) ;
#10195=CARTESIAN_POINT ( 'NONE',  ( -11.21908421996108629, -20.46040770435011069, 25.91992750791694888 ) ) ;
#10197=CARTESIAN_POINT ( 'NONE',  ( -14.83517299489739649, -18.99999999999997868, -0.9863224920830417908 ) ) ;
#10204=CARTESIAN_POINT ( 'NONE',  ( -19.24771351637086880, -26.64274437364857206, 4.486322492083041347 ) ) ;
#10205=CARTESIAN_POINT ( 'NONE',  ( -21.14459132904236327, -27.35725562635143149, 7.763677507916957765 ) ) ;
#10207=CARTESIAN_POINT ( 'NONE',  ( -18.78091578003892081, -20.46040770435013556, 42.33007249208301914 ) ) ;
#10211=CARTESIAN_POINT ( 'NONE',  ( -20.04416526290808065, -25.17491895705300209, 39.48242750791695244 ) ) ;
#10216=CARTESIAN_POINT ( 'NONE',  ( -9.955834737091903364, -25.17491895705295235, 34.01757249208303335 ) ) ;
#10231=CARTESIAN_POINT ( 'NONE',  ( -18.78091578003889950, -27.53959229564985378, 2.294927507916958209 ) ) ;
#10232=CARTESIAN_POINT ( 'NONE',  ( -14.83517299489738761, -20.99999999999997513, 41.01367750791695954 ) ) ;
#10234=CARTESIAN_POINT ( 'NONE',  ( -13.82508104294702100, -18.95583473709188382, 1.205072492083041125 ) ) ;
#10237=CARTESIAN_POINT ( 'NONE',  ( -14.83517299489739649, -18.99999999999997868, -0.9863224920830417908 ) ) ;
#10238=CARTESIAN_POINT ( 'NONE',  ( -9.999999999999994671, -24.16482700510257686, 0.3261775079169582647 ) ) ;
#10248=CARTESIAN_POINT ( 'NONE',  ( -9.996306089212408708, -18.75498260482328661, 22.64257249208304046 ) ) ;
#10249=CARTESIAN_POINT ( 'NONE',  ( -17.35725562635140307, -28.41254052147349185, 4.048822492083041347 ) ) ;
#10252=CARTESIAN_POINT ( 'NONE',  ( -13.35725562635142794, -21.48433729119796709, 4.701177507916959541 ) ) ;
#10253=CARTESIAN_POINT ( 'NONE',  ( -12.95952864787948755, -30.95583473709188382, 3.392572492083039570 ) ) ;
#10271=CARTESIAN_POINT ( 'NONE',  ( -13.28918265808472299, -31.04416526290805933, 6.669927507916955989 ) ) ;
#10276=CARTESIAN_POINT ( 'NONE',  ( -12.04416526290808420, -23.03132541760398766, 2.080072492083043567 ) ) ;
#10280=CARTESIAN_POINT ( 'NONE',  ( -15.96867458239597326, -26.95583473709190159, 1.857427507916959986 ) ) ;
#10292=CARTESIAN_POINT ( 'NONE',  ( -19.99999999999999645, -23.83517299489738051, 23.95117750791695954 ) ) ;
#10294=CARTESIAN_POINT ( 'NONE',  ( -15.16482700510259640, -28.99999999999998224, 6.888677507916957765 ) ) ;
#10298=CARTESIAN_POINT ( 'NONE',  ( -12.64274437364858628, -19.58745947852646552, 1.423822492083040903 ) ) ;
#10300=CARTESIAN_POINT ( 'NONE',  ( -18.64274437364853654, -29.97976432393976509, 2.076177507916956433 ) ) ;
#10303=CARTESIAN_POINT ( 'NONE',  ( -12.68318583509882380, -26.07549068051207541, 2.955072492083043123 ) ) ;
#10307=CARTESIAN_POINT ( 'NONE',  ( -10.16296170546024058, -21.54789006923565964, 6.318196777486344053E-14 ) ) ;
#10309=CARTESIAN_POINT ( 'NONE',  ( -10.75228648362910100, -26.64274437364854009, 37.51367750791695954 ) ) ;
#10325=CARTESIAN_POINT ( 'NONE',  ( -15.16482700510259640, -28.99999999999998224, 6.888677507916957765 ) ) ;
#10327=CARTESIAN_POINT ( 'NONE',  ( -9.999999999999994671, -24.16482700510257686, 16.07617750791695954 ) ) ;
#10330=CARTESIAN_POINT ( 'NONE',  ( -10.04416526290808953, -22.49542703274172695, 7.330072492083041347 ) ) ;
#10333=CARTESIAN_POINT ( 'NONE',  ( -19.99999999999999645, -23.83517299489738051, 8.201177507916957765 ) ) ;
#10334=CARTESIAN_POINT ( 'NONE',  ( -9.999999999999994671, -24.16482700510257686, 10.82617750791695777 ) ) ;
#10347=CARTESIAN_POINT ( 'NONE',  ( -18.64274437364860049, -18.02023567606023491, 21.54882249208304046 ) ) ;
#10348=SHAPE_REPRESENTATION_RELATIONSHIP ( 'NONE' , 'NONE' ,  #7269, #12712 ) ;
#10355=CARTESIAN_POINT ( 'NONE',  ( -16.35725562635142794, -21.31951028609535470, 19.57617750791696309 ) ) ;
#10357=CARTESIAN_POINT ( 'NONE',  ( -14.83517299489734853, -30.99999999999998224, 3.611322492083039570 ) ) ;
#10367=CARTESIAN_POINT ( 'NONE',  ( -10.36397326697674437, -22.27655863311489171, -4.119453415160648062E-17 ) ) ;
#10377=CARTESIAN_POINT ( 'NONE',  ( -20.24501739517664234, -29.00369391078761439, 18.04492750791695954 ) ) ;
#10382=CARTESIAN_POINT ( 'NONE',  ( -19.95583473709190514, -25.50457296725822687, 41.45507249208304046 ) ) ;
#10387=CARTESIAN_POINT ( 'NONE',  ( -17.68048971390461688, -25.35725562635141372, 7.763677507916960430 ) ) ;
#10395=SHAPE_DEFINITION_REPRESENTATION ( #13329, #7269 ) ;
#10399=CARTESIAN_POINT ( 'NONE',  ( -10.58745947852649927, -21.64274437364853654, 15.63867750791695777 ) ) ;
#10402=CARTESIAN_POINT ( 'NONE',  ( -10.75228648362912232, -21.35725562635138530, 7.111322492083040459 ) ) ;
#10404=CARTESIAN_POINT ( 'NONE',  ( -12.48433729119799196, -22.35725562635139596, 7.111322492083044011 ) ) ;
#10407=CARTESIAN_POINT ( 'NONE',  ( -10.82721319696594442, -20.04049993200424140, 1.010946030694833753E-16 ) ) ;
#10409=CARTESIAN_POINT ( 'NONE',  ( -13.82508104294698192, -29.04416526290806644, 38.16992750791695244 ) ) ;
#10421=CARTESIAN_POINT ( 'NONE',  ( -9.955834737091912245, -22.82508104294696594, 5.357427507916956877 ) ) ;
#10422=CARTESIAN_POINT ( 'NONE',  ( -11.46040770435012668, -27.78091578003887463, 16.73242750791695954 ) ) ;
#10425=CARTESIAN_POINT ( 'NONE',  ( -19.95583473709190514, -25.50457296725822687, 4.705072492083039570 ) ) ;
#10428=CARTESIAN_POINT ( 'NONE',  ( -10.75228648362910100, -26.64274437364854009, 0.7636775079169582092 ) ) ;
#10429=APPLICATION_CONTEXT ( 'automotive_design' ) ;
#10445=CARTESIAN_POINT ( 'NONE',  ( -8.044165262908093084, -21.95952864787946979, 12.58007249208304046 ) ) ;
#10450=CARTESIAN_POINT ( 'NONE',  ( -11.95583473709191047, -23.36097942780921954, 15.85742750791696309 ) ) ;
#10452=CARTESIAN_POINT ( 'NONE',  ( -16.71081734191527346, -16.95583473709190159, 40.79492750791695244 ) ) ;
#10461=CARTESIAN_POINT ( 'NONE',  ( -12.84660369577459882, -20.49551723709882012, 7.657166918419683734E-13 ) ) ;
#10472=CARTESIAN_POINT ( 'NONE',  ( -20.24501739517664234, -29.00369391078761439, 23.29492750791695599 ) ) ;
#10478=CARTESIAN_POINT ( 'NONE',  ( -17.07549068051208963, -26.31681416490115311, 14.76757249208304223 ) ) ;
#10482=CARTESIAN_POINT ( 'NONE',  ( -15.96867458239597326, -26.95583473709190159, 22.85742750791695954 ) ) ;
#10495=CARTESIAN_POINT ( 'NONE',  ( -16.50457296725820555, -28.95583473709189448, 22.85742750791695954 ) ) ;
#10498=CARTESIAN_POINT ( 'NONE',  ( -9.999999999999994671, -23.83517299489734143, 23.29882249208304046 ) ) ;
#10503=CARTESIAN_POINT ( 'NONE',  ( -18.04416526290808775, -23.36097942780924441, 5.142572492083044011 ) ) ;
#10522=CARTESIAN_POINT ( 'NONE',  ( -10.75228648362910100, -26.64274437364854009, 0.7636775079169582092 ) ) ;
#10523=CARTESIAN_POINT ( 'NONE',  ( -9.999999999999994671, -24.16482700510257686, 10.82617750791695777 ) ) ;
#10525=CARTESIAN_POINT ( 'NONE',  ( -18.53959229564982536, -27.78091578003890660, 4.267572492083038682 ) ) ;
#10529=CARTESIAN_POINT ( 'NONE',  ( -12.35725562635143682, -19.75228648362908501, 4.701177507916957765 ) ) ;
#10531=CARTESIAN_POINT ( 'NONE',  ( -9.955834737091912245, -22.82508104294696238, 15.85742750791695954 ) ) ;
#10545=CARTESIAN_POINT ( 'NONE',  ( -7.955834737091903364, -25.71081734191518464, 23.51757249208304401 ) ) ;
#10551=CARTESIAN_POINT ( 'NONE',  ( -12.31951028609537602, -22.64274437364854364, 10.38867750791695954 ) ) ;
#10553=CARTESIAN_POINT ( 'NONE',  ( -20.00369391078757886, -29.24501739517668142, 4.267572492083039570 ) ) ;
#10570=CARTESIAN_POINT ( 'NONE',  ( -20.00369391078762860, -18.75498260482333279, 19.35742750791695954 ) ) ;
#10574=CARTESIAN_POINT ( 'NONE',  ( -12.04416526290808420, -23.03132541760398766, 12.58007249208304401 ) ) ;
#10581=CARTESIAN_POINT ( 'NONE',  ( -12.04416526290807887, -24.96867458239596260, 16.29492750791696665 ) ) ;
#10592=CARTESIAN_POINT ( 'NONE',  ( -16.17491895705301275, -18.95583473709189803, 40.79492750791695954 ) ) ;
#10594=CARTESIAN_POINT ( 'NONE',  ( -11.46040770435012668, -27.78091578003887463, 16.73242750791695954 ) ) ;
#10598=CARTESIAN_POINT ( 'NONE',  ( -18.53959229564982536, -27.78091578003890660, 20.01757249208304046 ) ) ;
#10601=CARTESIAN_POINT ( 'NONE',  ( -11.99999999999999289, -23.83517299489735564, 18.04882249208304046 ) ) ;
#10619=CARTESIAN_POINT ( 'NONE',  ( -19.41254052147348830, -26.35725562635142083, 13.01367750791695777 ) ) ;
#10620=CARTESIAN_POINT ( 'NONE',  ( -12.35725562635143682, -19.75228648362908501, 9.951177507916959541 ) ) ;
#10622=CARTESIAN_POINT ( 'NONE',  ( -10.58745947852648328, -26.35725562635138530, 23.73632249208304046 ) ) ;
#10624=CARTESIAN_POINT ( 'NONE',  ( -17.35725562635144215, -19.58745947852648683, 3.826177507916958209 ) ) ;
#10626=CARTESIAN_POINT ( 'NONE',  ( -13.49542703274178201, -19.04416526290806289, 25.48242750791695244 ) ) ;
#10633=CIRCLE ( 'NONE', #1393, 0.9999999999999974465 ) ;
#10641=CARTESIAN_POINT ( 'NONE',  ( -13.28918265808478694, -16.95583473709189093, 11.70507249208304046 ) ) ;
#10643=CARTESIAN_POINT ( 'NONE',  ( -16.17491895705296656, -29.04416526290807354, 14.33007249208304046 ) ) ;
#10646=CARTESIAN_POINT ( 'NONE',  ( -17.95583473709191580, -23.03132541760400898, 18.91992750791695954 ) ) ;
#10648=CARTESIAN_POINT ( 'NONE',  ( -21.99999999999999289, -24.16482700510262305, 10.17382249208303868 ) ) ;
#10668=CARTESIAN_POINT ( 'NONE',  ( -9.020235676060220698, -27.64274437364852588, 16.51367750791695954 ) ) ;
#10673=CARTESIAN_POINT ( 'NONE',  ( -11.95583473709190514, -24.63902057219072361, 18.26757249208304401 ) ) ;
#10676=CARTESIAN_POINT ( 'NONE',  ( -22.04416526290807710, -25.71081734191525925, 2.732427507916957321 ) ) ;
#10681=CARTESIAN_POINT ( 'NONE',  ( -12.92450931948788906, -26.31681416490114245, 16.73242750791696309 ) ) ;
#10694=CARTESIAN_POINT ( 'NONE',  ( -17.35725562635144215, -19.58745947852648683, 35.32617750791695954 ) ) ;
#10699=CARTESIAN_POINT ( 'NONE',  ( -13.82508104294698192, -29.04416526290806644, 22.41992750791695244 ) ) ;
#10702=CARTESIAN_POINT ( 'NONE',  ( -11.21908421996106320, -27.53959229564982181, 18.70507249208304401 ) ) ;
#10705=CARTESIAN_POINT ( 'NONE',  ( -17.95583473709190869, -24.96867458239598037, 25.70507249208304756 ) ) ;
#10723=CARTESIAN_POINT ( 'NONE',  ( -18.53959229564986799, -20.21908421996107563, 14.10742750791695777 ) ) ;
#10725=CARTESIAN_POINT ( 'NONE',  ( -9.999999999999994671, -23.83517299489734143, 23.29882249208304046 ) ) ;
#10727=CARTESIAN_POINT ( 'NONE',  ( -12.35725562635143682, -19.75228648362908501, 9.951177507916959541 ) ) ;
#10729=CARTESIAN_POINT ( 'NONE',  ( -15.16482700510259640, -28.99999999999998224, 17.38867750791695599 ) ) ;
#10741=CARTESIAN_POINT ( 'NONE',  ( -16.71081734191520596, -31.04416526290808065, 35.33007249208304046 ) ) ;
#10743=CARTESIAN_POINT ( 'NONE',  ( -18.53959229564983247, -27.78091578003891016, 4.267572492083039570 ) ) ;
#10745=CARTESIAN_POINT ( 'NONE',  ( -15.96867458239597326, -26.95583473709190159, 17.60742750791696309 ) ) ;
#10747=CARTESIAN_POINT ( 'NONE',  ( -14.83517299489734853, -30.99999999999998224, 14.11132249208304046 ) ) ;
#10762=CARTESIAN_POINT ( 'NONE',  ( -13.28918265808472299, -31.04416526290805933, 11.91992750791695777 ) ) ;
#10765=CARTESIAN_POINT ( 'NONE',  ( -13.64274437364857739, -21.31951028609534760, 17.17382249208304401 ) ) ;
#10766=CARTESIAN_POINT ( 'NONE',  ( -22.04416526290807710, -25.71081734191525925, 13.23242750791695777 ) ) ;
#10771=CARTESIAN_POINT ( 'NONE',  ( -17.68048971390461688, -25.35725562635141372, 18.26367750791696309 ) ) ;
#10779=DIRECTION ( 'NONE',  ( 0.000000000000000000, 1.000000000000000000, 0.000000000000000000 ) ) ;
#10791=CARTESIAN_POINT ( 'NONE',  ( -17.64274437364855430, -28.24771351637087236, 17.82617750791695599 ) ) ;
#10796=CARTESIAN_POINT ( 'NONE',  ( -11.46040770435014977, -20.21908421996103655, 12.14257249208304046 ) ) ;
#10798=CARTESIAN_POINT ( 'NONE',  ( -17.31681416490117087, -21.92450931948788551, 21.33007249208304401 ) ) ;
#10817=CARTESIAN_POINT ( 'NONE',  ( -10.75228648362910100, -26.64274437364854009, 11.26367750791695777 ) ) ;
#10819=CARTESIAN_POINT ( 'NONE',  ( -11.46040770435014977, -20.21908421996103655, 12.14257249208304046 ) ) ;
#10823=CARTESIAN_POINT ( 'NONE',  ( -11.46040770435012668, -27.78091578003887463, 21.98242750791695244 ) ) ;
#10827=CARTESIAN_POINT ( 'NONE',  ( -17.35725562635144215, -19.58745947852648683, 19.57617750791695954 ) ) ;
#10840=CARTESIAN_POINT ( 'NONE',  ( -21.99999999999999289, -24.16482700510262305, 31.17382249208304046 ) ) ;
#10843=CARTESIAN_POINT ( 'NONE',  ( -19.99999999999999645, -24.16482700510261949, 10.17382249208304046 ) ) ;
#10846=CARTESIAN_POINT ( 'NONE',  ( -11.99999999999999289, -24.16482700510258752, 31.82617750791696309 ) ) ;
#10849=CARTESIAN_POINT ( 'NONE',  ( -17.04047135212050890, -17.04416526290807710, 21.76757249208304401 ) ) ;
#10866=CARTESIAN_POINT ( 'NONE',  ( -21.99999999999999289, -23.83517299489739116, 23.95117750791696309 ) ) ;
#10870=CARTESIAN_POINT ( 'NONE',  ( -11.99999999999999289, -23.83517299489735564, 28.54882249208304046 ) ) ;
#10871=CARTESIAN_POINT ( 'NONE',  ( -11.64274437364854187, -30.14459132904234195, 22.20117750791695599 ) ) ;
#10876=CARTESIAN_POINT ( 'NONE',  ( -17.31681416490115311, -26.07549068051209318, 12.79492750791696132 ) ) ;
#10884=PLANE ( 'NONE',  #10150 ) ;
#10892=CARTESIAN_POINT ( 'NONE',  ( -19.95583473709191580, -22.49542703274176603, 29.41992750791695599 ) ) ;
#10897=CARTESIAN_POINT ( 'NONE',  ( -9.955834737091903364, -25.17491895705294880, 23.51757249208304401 ) ) ;
#10898=CARTESIAN_POINT ( 'NONE',  ( -15.96867458239599635, -21.04416526290806999, 21.76757249208304756 ) ) ;
#10914=CARTESIAN_POINT ( 'NONE',  ( -9.999999999999994671, -24.16482700510257686, 21.32617750791695599 ) ) ;
#10917=CARTESIAN_POINT ( 'NONE',  ( -9.955834737091903364, -25.17491895705294880, 18.26757249208304401 ) ) ;
#10919=CARTESIAN_POINT ( 'NONE',  ( -11.46040770435012668, -27.78091578003887463, 16.73242750791695954 ) ) ;
#10922=CARTESIAN_POINT ( 'NONE',  ( -11.46040770435012490, -27.78091578003888173, 21.98242750791695244 ) ) ;
#10924=CARTESIAN_POINT ( 'NONE',  ( -15.16482700510263371, -18.99999999999997868, 27.23632249208304046 ) ) ;
#10935=CARTESIAN_POINT ( 'NONE',  ( -20.97976432393974022, -27.64274437364858628, 35.98632249208303335 ) ) ;
#10937=CARTESIAN_POINT ( 'NONE',  ( -13.49542703274174116, -28.95583473709188738, 13.89257249208304046 ) ) ;
#10939=CARTESIAN_POINT ( 'NONE',  ( -14.03132541760401786, -21.04416526290806289, 35.98242750791695954 ) ) ;
#10941=CARTESIAN_POINT ( 'NONE',  ( -21.14459132904239169, -20.64274437364858628, 15.86132249208304223 ) ) ;
#10960=CARTESIAN_POINT ( 'NONE',  ( -22.04416526290807710, -25.71081734191525925, 28.98242750791695599 ) ) ;
#10964=CARTESIAN_POINT ( 'NONE',  ( -17.95583473709190869, -24.96867458239598037, 30.95507249208304401 ) ) ;
#10965=CARTESIAN_POINT ( 'NONE',  ( -20.00369391078762860, -18.75498260482333279, 19.35742750791695954 ) ) ;
#10971=CARTESIAN_POINT ( 'NONE',  ( -15.63902057219076269, -20.95583473709189448, 35.54492750791696665 ) ) ;
#10989=CARTESIAN_POINT ( 'NONE',  ( -12.64274437364855252, -28.41254052147347053, 32.70117750791696665 ) ) ;
#10994=CARTESIAN_POINT ( 'NONE',  ( -17.64274437364858983, -19.75228648362910633, 37.29882249208303335 ) ) ;
#10996=CARTESIAN_POINT ( 'NONE',  ( -12.48433729119799196, -22.35725562635139596, 17.61132249208304401 ) ) ;
#11014=CARTESIAN_POINT ( 'NONE',  ( -19.24771351637089367, -21.35725562635142438, 13.88867750791695954 ) ) ;
#11016=CARTESIAN_POINT ( 'NONE',  ( -11.21908421996106320, -27.53959229564982181, 13.45507249208304223 ) ) ;
#11018=CARTESIAN_POINT ( 'NONE',  ( -18.78091578003889950, -27.53959229564985378, 18.04492750791695954 ) ) ;
#11020=CARTESIAN_POINT ( 'NONE',  ( -9.955834737091912245, -22.82508104294696238, 36.85742750791696665 ) ) ;
#11022=CARTESIAN_POINT ( 'NONE',  ( -9.955834737091903364, -25.17491895705295235, 18.26757249208304401 ) ) ;
#11033=CARTESIAN_POINT ( 'NONE',  ( -21.99999999999999289, -24.16482700510262305, 25.92382249208304046 ) ) ;
#11036=CARTESIAN_POINT ( 'NONE',  ( -12.64274437364858628, -19.58745947852646552, 17.17382249208304401 ) ) ;
#11037=CARTESIAN_POINT ( 'NONE',  ( -15.63902057219076269, -20.95583473709189448, 30.29492750791697020 ) ) ;
#11040=CARTESIAN_POINT ( 'NONE',  ( -9.996306089212408708, -18.75498260482328661, 17.39257249208304046 ) ) ;
#11056=CARTESIAN_POINT ( 'NONE',  ( -20.24501739517664234, -29.00369391078761439, 33.79492750791695244 ) ) ;
#11060=CARTESIAN_POINT ( 'NONE',  ( -13.35725562635141195, -26.51566270880198672, 34.67382249208304756 ) ) ;
#11061=CARTESIAN_POINT ( 'NONE',  ( -20.97976432393977575, -20.35725562635143504, 24.38867750791695954 ) ) ;
#11066=CARTESIAN_POINT ( 'NONE',  ( -11.95583473709191047, -23.36097942780921954, 31.60742750791695599 ) ) ;
#11084=CARTESIAN_POINT ( 'NONE',  ( -15.16482700510259640, -28.99999999999998224, 27.88867750791695954 ) ) ;
#11088=CARTESIAN_POINT ( 'NONE',  ( -12.64274437364858628, -19.58745947852646552, 32.92382249208304046 ) ) ;
#11091=CARTESIAN_POINT ( 'NONE',  ( -13.35725562635141195, -26.51566270880198672, 29.42382249208304401 ) ) ;
#11107=CARTESIAN_POINT ( 'NONE',  ( -9.999999999999994671, -24.16482700510257686, 31.82617750791696309 ) ) ;
#11111=CARTESIAN_POINT ( 'NONE',  ( -10.04416526290808953, -22.49542703274172695, 28.33007249208304401 ) ) ;
#11113=CARTESIAN_POINT ( 'NONE',  ( -15.16482700510259640, -28.99999999999998224, 12.13867750791695777 ) ) ;
#11115=CARTESIAN_POINT ( 'NONE',  ( -10.58745947852649927, -21.64274437364853654, 36.63867750791695954 ) ) ;
#11117=CARTESIAN_POINT ( 'NONE',  ( -14.83517299489735741, -28.99999999999998224, 19.36132249208304046 ) ) ;
#11127=CARTESIAN_POINT ( 'NONE',  ( -9.754982604823302594, -29.00369391078756465, 29.20507249208304046 ) ) ;
#11129=CARTESIAN_POINT ( 'NONE',  ( -17.07549068051210739, -21.68318583509881847, 35.10742750791696665 ) ) ;
#11131=CARTESIAN_POINT ( 'NONE',  ( -9.020235676060250896, -20.35725562635137820, 12.36132249208304046 ) ) ;
#11148=CARTESIAN_POINT ( 'NONE',  ( -16.71081734191527346, -16.95583473709190159, 35.54492750791695954 ) ) ;
#11152=CARTESIAN_POINT ( 'NONE',  ( -18.04416526290808775, -23.36097942780924441, 31.39257249208304401 ) ) ;
#11153=CARTESIAN_POINT ( 'NONE',  ( -21.95583473709191580, -21.95952864787954084, 13.66992750791695954 ) ) ;
#11158=CARTESIAN_POINT ( 'NONE',  ( -15.63902057219076269, -20.95583473709189448, 30.29492750791697020 ) ) ;
#11170=CARTESIAN_POINT ( 'NONE',  ( -15.00000000000001421, -18.99999999999997868, 42.00000000000000000 ) ) ;
#11174=CARTESIAN_POINT ( 'NONE',  ( -11.21908421996108629, -20.46040770435011069, 36.41992750791695954 ) ) ;
#11179=CARTESIAN_POINT ( 'NONE',  ( -17.64274437364858983, -19.75228648362910633, 32.04882249208304046 ) ) ;
#11182=CARTESIAN_POINT ( 'NONE',  ( -17.95583473709190869, -24.96867458239598037, 30.95507249208304401 ) ) ;
#11197=CARTESIAN_POINT ( 'NONE',  ( -19.95583473709191580, -22.49542703274176603, 34.66992750791694533 ) ) ;
#11199=CARTESIAN_POINT ( 'NONE',  ( -9.999999999999994671, -23.83517299489734143, 33.79882249208304046 ) ) ;
#11201=CARTESIAN_POINT ( 'NONE',  ( -11.21908421996108629, -20.46040770435011069, 25.91992750791694888 ) ) ;
#11203=CARTESIAN_POINT ( 'NONE',  ( -12.64274437364855252, -28.41254052147347053, 27.45117750791695954 ) ) ;
#11205=CARTESIAN_POINT ( 'NONE',  ( -19.24771351637086880, -26.64274437364857206, 30.73632249208304401 ) ) ;
#11215=CARTESIAN_POINT ( 'NONE',  ( -18.04416526290808420, -24.63902057219074493, 34.23242750791695954 ) ) ;
#11218=CARTESIAN_POINT ( 'NONE',  ( -8.044165262908093084, -21.95952864787946979, 38.83007249208303335 ) ) ;
#11234=CARTESIAN_POINT ( 'NONE',  ( -7.999999999999996447, -24.16482700510256976, 26.57617750791695954 ) ) ;
#11239=CARTESIAN_POINT ( 'NONE',  ( -12.48433729119799196, -22.35725562635139596, 33.36132249208304756 ) ) ;
#11240=CARTESIAN_POINT ( 'NONE',  ( -13.28918265808472299, -31.04416526290805933, 38.16992750791695954 ) ) ;
#11246=CARTESIAN_POINT ( 'NONE',  ( -12.92450931948788906, -26.31681416490114245, 32.48242750791695954 ) ) ;
#11250=CARTESIAN_POINT ( 'NONE',  ( -15.00000000000001599, -18.99999999999997868, 0.000000000000000000 ) ) ;
#11266=CARTESIAN_POINT ( 'NONE',  ( -9.999999999999994671, -24.16482700510257686, 37.07617750791695954 ) ) ;
#11270=CARTESIAN_POINT ( 'NONE',  ( -19.24771351637086880, -26.64274437364857206, 35.98632249208304046 ) ) ;
#11274=CARTESIAN_POINT ( 'NONE',  ( -13.64274437364857739, -21.31951028609534760, 27.67382249208304401 ) ) ;
#11296=CARTESIAN_POINT ( 'NONE',  ( -13.49542703274178379, -19.04416526290806289, 35.98242750791696665 ) ) ;
#11298=CARTESIAN_POINT ( 'NONE',  ( -9.999999999999994671, -23.83517299489734143, 39.04882249208304046 ) ) ;
#11301=CARTESIAN_POINT ( 'NONE',  ( -11.46040770435012668, -27.78091578003887463, 32.48242750791695954 ) ) ;
#11304=CARTESIAN_POINT ( 'NONE',  ( -10.04416526290807710, -25.50457296725819489, 37.29492750791695954 ) ) ;
#11306=CARTESIAN_POINT ( 'NONE',  ( -16.50457296725825174, -19.04416526290807354, 21.76757249208304401 ) ) ;
#11319=CARTESIAN_POINT ( 'NONE',  ( -9.999999999999994671, -24.16482700510257686, 5.576177507916958653 ) ) ;
#11321=CARTESIAN_POINT ( 'NONE',  ( -11.64274437364859693, -17.85540867095757989, 27.67382249208304401 ) ) ;
#11336=CARTESIAN_POINT ( 'NONE',  ( -7.999999999999996447, -23.83517299489733432, 7.548822492083037794 ) ) ;
#11341=CARTESIAN_POINT ( 'NONE',  ( -11.99999999999999289, -24.16482700510258752, 5.576177507916960430 ) ) ;
#11342=CARTESIAN_POINT ( 'NONE',  ( -12.95952864787955150, -17.04416526290805933, 25.48242750791696309 ) ) ;
#11346=EDGE_LOOP ( 'NONE', ( #18903, #18884 ) ) ;
#11360=CARTESIAN_POINT ( 'NONE',  ( -18.64274437364853654, -29.97976432393976509, 7.326177507916955989 ) ) ;
#11363=CARTESIAN_POINT ( 'NONE',  ( -17.35725562635140307, -28.41254052147349185, 30.29882249208304401 ) ) ;
#11366=CARTESIAN_POINT ( 'NONE',  ( -14.36097942780925685, -20.95583473709189093, 32.70507249208304756 ) ) ;
#11377=CARTESIAN_POINT ( 'NONE',  ( -10.75228648362910100, -26.64274437364854009, 32.26367750791695954 ) ) ;
#11385=CARTESIAN_POINT ( 'NONE',  ( -10.58745947852649927, -21.64274437364853654, 36.63867750791695954 ) ) ;
#11387=CARTESIAN_POINT ( 'NONE',  ( -19.41254052147350961, -21.64274437364857562, 26.36132249208304401 ) ) ;
#11390=CARTESIAN_POINT ( 'NONE',  ( -10.58745947852649927, -21.64274437364853654, 26.13867750791695599 ) ) ;
#11393=CARTESIAN_POINT ( 'NONE',  ( -19.99999999999999645, -23.83517299489738051, 34.45117750791696665 ) ) ;
#11407=CARTESIAN_POINT ( 'NONE',  ( -16.64274437364856496, -26.51566270880199738, 38.82617750791695954 ) ) ;
#11410=CARTESIAN_POINT ( 'NONE',  ( -16.71081734191520596, -31.04416526290808065, 35.33007249208304046 ) ) ;
#11426=CARTESIAN_POINT ( 'NONE',  ( -20.00369391078757886, -29.24501739517668142, 4.267572492083039570 ) ) ;
#11433=CARTESIAN_POINT ( 'NONE',  ( -17.31681416490115311, -26.07549068051209318, 2.294927507916959986 ) ) ;
#11434=CARTESIAN_POINT ( 'NONE',  ( -22.04416526290807710, -25.71081734191525925, 34.23242750791695244 ) ) ;
#11455=CARTESIAN_POINT ( 'NONE',  ( -18.35725562635144925, -17.85540867095761186, 9.076177507916954212 ) ) ;
#11458=CARTESIAN_POINT ( 'NONE',  ( -14.83517299489736985, -26.99999999999998579, 8.861322492083040459 ) ) ;
#11463=CARTESIAN_POINT ( 'NONE',  ( -16.64274437364858272, -21.48433729119797420, 37.29882249208304046 ) ) ;
#11473=CARTESIAN_POINT ( 'NONE',  ( -12.64274437364855252, -28.41254052147347053, 27.45117750791695954 ) ) ;
#11476=CARTESIAN_POINT ( 'NONE',  ( -12.64274437364855252, -28.41254052147347053, 1.201177507916958431 ) ) ;
#11479=CARTESIAN_POINT ( 'NONE',  ( -15.16482700510263371, -18.99999999999997868, 6.236322492083041347 ) ) ;
#11480=CARTESIAN_POINT ( 'NONE',  ( -13.82508104294698192, -29.04416526290806644, 38.16992750791695244 ) ) ;
#11482=CARTESIAN_POINT ( 'NONE',  ( -11.46040770435014977, -20.21908421996103655, 33.14257249208303335 ) ) ;
#11487=CARTESIAN_POINT ( 'NONE',  ( -20.04416526290808065, -25.17491895705300209, 23.73242750791694888 ) ) ;
#11501=CARTESIAN_POINT ( 'NONE',  ( -15.16482700510259640, -28.99999999999998224, 6.888677507916957765 ) ) ;
#11503=CARTESIAN_POINT ( 'NONE',  ( -20.24501739517669563, -18.99630608921239627, 37.08007249208304046 ) ) ;
#11518=CARTESIAN_POINT ( 'NONE',  ( -16.71081734191527346, -16.95583473709190159, 40.79492750791695244 ) ) ;
#11523=CARTESIAN_POINT ( 'NONE',  ( -17.95583473709191580, -23.03132541760400898, 3.169927507916960874 ) ) ;
#11524=CARTESIAN_POINT ( 'NONE',  ( -11.64274437364854187, -30.14459132904234195, 32.70117750791695244 ) ) ;
#11549=CARTESIAN_POINT ( 'NONE',  ( -9.020235676060220698, -27.64274437364852588, 0.7636775079169565439 ) ) ;
#11552=CARTESIAN_POINT ( 'NONE',  ( -11.95583473709190514, -24.63902057219072361, 7.767572492083043123 ) ) ;
#11556=CARTESIAN_POINT ( 'NONE',  ( -17.31681416490117087, -21.92450931948788551, 42.33007249208304756 ) ) ;
#11569=CARTESIAN_POINT ( 'NONE',  ( -16.50457296725820555, -28.95583473709189448, 22.85742750791695954 ) ) ;
#11577=CARTESIAN_POINT ( 'NONE',  ( -19.95583473709190514, -25.50457296725822687, 9.955072492083036906 ) ) ;
#11578=CARTESIAN_POINT ( 'NONE',  ( -17.04047135212043784, -30.95583473709190159, 1.857427507916956211 ) ) ;
#11581=CARTESIAN_POINT ( 'NONE',  ( -14.36097942780925685, -20.95583473709189093, 11.70507249208304223 ) ) ;
#11586=CARTESIAN_POINT ( 'NONE',  ( -19.24771351637089367, -21.35725562635142438, 29.63867750791695599 ) ) ;
#11590=CARTESIAN_POINT ( 'NONE',  ( -9.999999999999994671, -23.83517299489734143, 33.79882249208304046 ) ) ;
#11601=CARTESIAN_POINT ( 'NONE',  ( -20.04416526290808065, -25.17491895705300209, 7.982427507916958653 ) ) ;
#11603=CARTESIAN_POINT ( 'NONE',  ( -21.99999999999999289, -24.16482700510262305, 31.17382249208304046 ) ) ;
#11606=CARTESIAN_POINT ( 'NONE',  ( -16.35725562635142794, -21.31951028609535470, 35.32617750791695244 ) ) ;
#11607=CARTESIAN_POINT ( 'NONE',  ( -10.04416526290807710, -25.50457296725819489, 0.5449275079169580982 ) ) ;
#11622=CARTESIAN_POINT ( 'NONE',  ( -21.99999999999999289, -24.16482700510262305, 4.923822492083038682 ) ) ;
#11628=CARTESIAN_POINT ( 'NONE',  ( -17.95583473709190869, -24.96867458239598037, 41.45507249208304046 ) ) ;
#11629=CARTESIAN_POINT ( 'NONE',  ( -8.044165262908075320, -26.04047135212042718, 37.29492750791695954 ) ) ;
#11650=CARTESIAN_POINT ( 'NONE',  ( -7.955834737091916686, -22.28918265808470522, 0.1074275079169565300 ) ) ;
#11654=CARTESIAN_POINT ( 'NONE',  ( -17.31681416490117087, -21.92450931948788551, 5.580072492083043123 ) ) ;
#11660=CARTESIAN_POINT ( 'NONE',  ( -15.16482700510260706, -26.99999999999998579, 1.638677507916960208 ) ) ;
#11670=CARTESIAN_POINT ( 'NONE',  ( -19.24771351637089367, -21.35725562635142438, 24.38867750791695954 ) ) ;
#11671=DIRECTION ( 'NONE',  ( -0.1648270051026180794, 0.000000000000000000, 0.9863224920830415687 ) ) ;
#11672=FACE_OUTER_BOUND ( 'NONE', #15273, .T. ) ;
#11676=CARTESIAN_POINT ( 'NONE',  ( -20.24501739517669563, -18.99630608921239627, 42.33007249208303335 ) ) ;
#11677=CARTESIAN_POINT ( 'NONE',  ( -17.04047135212043784, -30.95583473709190159, 7.107427507916957765 ) ) ;
#11679=CARTESIAN_POINT ( 'NONE',  ( -19.95583473709190514, -25.50457296725822687, 41.45507249208304046 ) ) ;
#11683=CARTESIAN_POINT ( 'NONE',  ( -16.50457296725820555, -28.95583473709189448, 38.60742750791694533 ) ) ;
#11687=CARTESIAN_POINT ( 'NONE',  ( -16.50457296725825174, -19.04416526290807354, 37.51757249208304046 ) ) ;
#11699=CARTESIAN_POINT ( 'NONE',  ( -12.35725562635143682, -19.75228648362908501, 4.701177507916957765 ) ) ;
#11701=CARTESIAN_POINT ( 'NONE',  ( -18.78091578003892081, -20.46040770435013556, 5.580072492083041347 ) ) ;
#11703=CARTESIAN_POINT ( 'NONE',  ( -17.31681416490115311, -26.07549068051209318, 39.04492750791695954 ) ) ;
#11704=CARTESIAN_POINT ( 'NONE',  ( -19.24771351637089367, -21.35725562635142438, 8.638677507916957765 ) ) ;
#11716=CARTESIAN_POINT ( 'NONE',  ( -18.64274437364853654, -29.97976432393976509, 38.82617750791695244 ) ) ;
#11721=CARTESIAN_POINT ( 'NONE',  ( -16.35725562635142794, -21.31951028609535470, 3.826177507916959986 ) ) ;
#11722=CARTESIAN_POINT ( 'NONE',  ( -21.95583473709189803, -26.04047135212049469, 9.955072492083038682 ) ) ;
#11743=CARTESIAN_POINT ( 'NONE',  ( -16.71081734191527346, -16.95583473709190159, 4.044927507916956877 ) ) ;
#11747=CARTESIAN_POINT ( 'NONE',  ( -9.955834737091903364, -25.17491895705294880, 39.26757249208304046 ) ) ;
#11752=CARTESIAN_POINT ( 'NONE',  ( -11.95583473709191047, -23.36097942780921954, 0.1074275079169599995 ) ) ;
#11754=DIRECTION ( 'NONE',  ( 0.1648270051026190508, 0.000000000000000000, -0.9863224920830413467 ) ) ;
#11766=CARTESIAN_POINT ( 'NONE',  ( -9.955834737091912245, -22.82508104294696594, 21.10742750791695599 ) ) ;
#11770=CARTESIAN_POINT ( 'NONE',  ( -10.58745947852649927, -21.64274437364853654, 5.138677507916957765 ) ) ;
#11776=CARTESIAN_POINT ( 'NONE',  ( -14.83517299489735741, -28.99999999999998224, 3.611322492083041347 ) ) ;
#11777=CARTESIAN_POINT ( 'NONE',  ( -20.00369391078762860, -18.75498260482333279, 8.857427507916955989 ) ) ;
#11779=CARTESIAN_POINT ( 'NONE',  ( -11.99999999999999289, -23.83517299489735564, 7.548822492083043123 ) ) ;
#11799=CARTESIAN_POINT ( 'NONE',  ( -19.95583473709191580, -22.49542703274176603, 3.169927507916957321 ) ) ;
#11800=CARTESIAN_POINT ( 'NONE',  ( -13.49542703274178379, -19.04416526290806289, 9.732427507916959541 ) ) ;
#11802=CARTESIAN_POINT ( 'NONE',  ( -19.24771351637086880, -26.64274437364857206, 4.486322492083041347 ) ) ;
#11804=CARTESIAN_POINT ( 'NONE',  ( -11.46040770435012668, -27.78091578003887463, 6.232427507916956877 ) ) ;
#11805=CARTESIAN_POINT ( 'NONE',  ( -10.75228648362910100, -26.64274437364854009, 0.7636775079169582092 ) ) ;
#11817=CARTESIAN_POINT ( 'NONE',  ( -8.855408670957602979, -27.35725562635137820, 18.48632249208304046 ) ) ;
#11821=CARTESIAN_POINT ( 'NONE',  ( -17.07549068051210739, -21.68318583509881847, 14.10742750791695954 ) ) ;
#11823=CARTESIAN_POINT ( 'NONE',  ( -7.955834737091903364, -25.71081734191518464, 2.517572492083039126 ) ) ;
#11841=CARTESIAN_POINT ( 'NONE',  ( -7.955834737091916686, -22.28918265808470522, 21.10742750791695954 ) ) ;
#11846=CARTESIAN_POINT ( 'NONE',  ( -11.99999999999999289, -23.83517299489735564, 2.298822492083042235 ) ) ;
#11850=CARTESIAN_POINT ( 'NONE',  ( -15.96867458239597326, -26.95583473709190159, 7.107427507916960430 ) ) ;
#11863=EDGE_CURVE ( 'NONE', #14224, #12569, #18287, .T. ) ;
#11865=CARTESIAN_POINT ( 'NONE',  ( -12.35725562635143682, -19.75228648362908501, 36.20117750791695954 ) ) ;
#11867=CARTESIAN_POINT ( 'NONE',  ( -16.50457296725820555, -28.95583473709189448, 7.107427507916955989 ) ) ;
#11872=CARTESIAN_POINT ( 'NONE',  ( -13.82508104294702100, -18.95583473709188382, 6.455072492083041347 ) ) ;
#11874=CARTESIAN_POINT ( 'NONE',  ( -8.044165262908075320, -26.04047135212042718, 5.794927507916956877 ) ) ;
#11877=CARTESIAN_POINT ( 'NONE',  ( -12.04416526290808420, -23.03132541760398766, 7.330072492083044011 ) ) ;
#11882=CARTESIAN_POINT ( 'NONE',  ( -10.14139447615844425, -21.69985965322670296, -1.842058582391767589E-17 ) ) ;
#11901=CARTESIAN_POINT ( 'NONE',  ( -17.35725562635144215, -19.58745947852648683, 14.32617750791695777 ) ) ;
#11903=CARTESIAN_POINT ( 'NONE',  ( -10.04416526290808953, -22.49542703274172695, 2.080072492083040903 ) ) ;
#11908=CARTESIAN_POINT ( 'NONE',  ( -17.35725562635144215, -19.58745947852648683, 9.076177507916957765 ) ) ;
#11910=CARTESIAN_POINT ( 'NONE',  ( -10.04416526290807710, -25.50457296725819489, 11.04492750791695599 ) ) ;
#11924=CARTESIAN_POINT ( 'NONE',  ( -21.95583473709189803, -26.04047135212049469, 15.20507249208304046 ) ) ;
#11930=CARTESIAN_POINT ( 'NONE',  ( -12.92450931948788906, -26.31681416490114245, 21.98242750791695954 ) ) ;
#11932=CARTESIAN_POINT ( 'NONE',  ( -17.04047135212050890, -17.04416526290807710, 11.26757249208304046 ) ) ;
#11951=CARTESIAN_POINT ( 'NONE',  ( -15.16482700510258574, -30.99999999999998224, 22.63867750791695954 ) ) ;
#11956=CARTESIAN_POINT ( 'NONE',  ( -14.03132541760400009, -26.95583473709189448, 24.39257249208304046 ) ) ;
#11960=CARTESIAN_POINT ( 'NONE',  ( -15.96867458239599635, -21.04416526290806999, 42.76757249208304756 ) ) ;
#11971=CARTESIAN_POINT ( 'NONE',  ( -10.75228648362910100, -26.64274437364854009, 21.76367750791695599 ) ) ;
#11973=ORIENTED_EDGE ( 'NONE', *, *, #11863, .F. ) ;
#11974=CARTESIAN_POINT ( 'NONE',  ( -12.64274437364858628, -19.58745947852646552, 22.42382249208304401 ) ) ;
#11977=CARTESIAN_POINT ( 'NONE',  ( -17.99999999999999645, -24.16482700510260173, 10.17382249208304223 ) ) ;
#11980=CARTESIAN_POINT ( 'NONE',  ( -10.31147837279037738, -22.25502639194775512, -4.119453415160654225E-17 ) ) ;
#11982=CARTESIAN_POINT ( 'NONE',  ( -17.35725562635144215, -19.58745947852648683, 40.57617750791696665 ) ) ;
#11994=CARTESIAN_POINT ( 'NONE',  ( -14.83517299489739649, -18.99999999999997868, 14.76367750791695777 ) ) ;
#11997=CARTESIAN_POINT ( 'NONE',  ( -20.04416526290809131, -22.82508104294699791, 10.39257249208304223 ) ) ;
#11999=CARTESIAN_POINT ( 'NONE',  ( -16.50457296725820555, -28.95583473709189448, 7.107427507916955989 ) ) ;
#12001=CARTESIAN_POINT ( 'NONE',  ( -17.64274437364855430, -28.24771351637087236, 17.82617750791695599 ) ) ;
#12016=CARTESIAN_POINT ( 'NONE',  ( -14.83517299489734853, -30.99999999999998224, 24.61132249208304046 ) ) ;
#12019=CARTESIAN_POINT ( 'NONE',  ( -13.82508104294702100, -18.95583473709188382, 1.205072492083040903 ) ) ;
#12022=CARTESIAN_POINT ( 'NONE',  ( -17.31681416490115311, -26.07549068051209318, 12.79492750791696132 ) ) ;
#12024=CARTESIAN_POINT ( 'NONE',  ( -14.83517299489740715, -16.99999999999997868, 41.01367750791695954 ) ) ;
#12044=CARTESIAN_POINT ( 'NONE',  ( -21.14459132904236327, -27.35725562635143149, 13.01367750791695777 ) ) ;
#12050=CARTESIAN_POINT ( 'NONE',  ( -17.95583473709190869, -24.96867458239598037, 15.20507249208304579 ) ) ;
#12054=CARTESIAN_POINT ( 'NONE',  ( -17.99999999999999645, -23.83517299489736985, 18.70117750791695599 ) ) ;
#12067=DIRECTION ( 'NONE',  ( -0.9863224920830415687, -6.560347287104328168E-15, -0.1648270051026180794 ) ) ;
#12068=CARTESIAN_POINT ( 'NONE',  ( -9.955834737091912245, -22.82508104294696594, 15.85742750791695777 ) ) ;
#12071=CARTESIAN_POINT ( 'NONE',  ( -16.17491895705296656, -29.04416526290807710, 24.83007249208304046 ) ) ;
#12076=CARTESIAN_POINT ( 'NONE',  ( -13.35725562635141195, -26.51566270880198672, 24.17382249208304046 ) ) ;
#12092=CARTESIAN_POINT ( 'NONE',  ( -19.41254052147348830, -26.35725562635142083, 23.51367750791695954 ) ) ;
#12093=CARTESIAN_POINT ( 'NONE',  ( -16.17491895705301275, -18.95583473709189803, 9.294927507916954212 ) ) ;
#12095=CARTESIAN_POINT ( 'NONE',  ( -10.58745947852648328, -26.35725562635138530, 7.986322492083041347 ) ) ;
#12099=CARTESIAN_POINT ( 'NONE',  ( -10.04416526290807710, -25.50457296725819489, 0.5449275079169579872 ) ) ;
#12101=CARTESIAN_POINT ( 'NONE',  ( -17.35725562635144215, -19.58745947852648683, 24.82617750791695954 ) ) ;
#12116=CARTESIAN_POINT ( 'NONE',  ( -11.64274437364859693, -17.85540867095757989, 11.92382249208304046 ) ) ;
#12118=CARTESIAN_POINT ( 'NONE',  ( -19.95583473709190514, -25.50457296725823042, 15.20507249208304046 ) ) ;
#12121=CARTESIAN_POINT ( 'NONE',  ( -11.99999999999999289, -24.16482700510258752, 16.07617750791696309 ) ) ;
#12123=CARTESIAN_POINT ( 'NONE',  ( -9.754982604823302594, -29.00369391078756465, 8.205072492083040459 ) ) ;
#12142=CARTESIAN_POINT ( 'NONE',  ( -9.996306089212364299, -29.24501739517662813, 16.73242750791695954 ) ) ;
#12146=CARTESIAN_POINT ( 'NONE',  ( -11.95583473709190514, -24.63902057219072361, 13.01757249208304401 ) ) ;
#12150=CARTESIAN_POINT ( 'NONE',  ( -16.64274437364856496, -26.51566270880199738, 12.57617750791695954 ) ) ;
#12164=CARTESIAN_POINT ( 'NONE',  ( -14.83517299489739649, -18.99999999999997868, 41.01367750791696665 ) ) ;
#12167=CARTESIAN_POINT ( 'NONE',  ( -19.95583473709191580, -22.49542703274176603, 18.91992750791694888 ) ) ;
#12171=CARTESIAN_POINT ( 'NONE',  ( -9.999999999999994671, -23.83517299489734143, 18.04882249208304401 ) ) ;
#12175=CARTESIAN_POINT ( 'NONE',  ( -14.83517299489736985, -26.99999999999998579, 14.11132249208304223 ) ) ;
#12193=CARTESIAN_POINT ( 'NONE',  ( -16.50457296725820555, -28.95583473709189448, 22.85742750791695954 ) ) ;
#12195=CARTESIAN_POINT ( 'NONE',  ( -19.24771351637086880, -26.64274437364857206, 25.48632249208304401 ) ) ;
#12198=CARTESIAN_POINT ( 'NONE',  ( -19.99999999999999645, -23.83517299489738051, 18.70117750791695954 ) ) ;
#12200=CARTESIAN_POINT ( 'NONE',  ( -19.24771351637089367, -21.35725562635142438, 13.88867750791695954 ) ) ;
#12214=CARTESIAN_POINT ( 'NONE',  ( -21.99999999999999289, -24.16482700510262305, 20.67382249208304046 ) ) ;
#12216=CARTESIAN_POINT ( 'NONE',  ( -16.17491895705296656, -29.04416526290807354, 9.080072492083038682 ) ) ;
#12218=CARTESIAN_POINT ( 'NONE',  ( -16.35725562635142794, -21.31951028609535470, 9.076177507916959541 ) ) ;
#12220=CARTESIAN_POINT ( 'NONE',  ( -16.71081734191520596, -31.04416526290808065, 19.58007249208303691 ) ) ;
#12244=CARTESIAN_POINT ( 'NONE',  ( -11.35725562635144925, -18.02023567606020293, 20.45117750791695954 ) ) ;
#12248=CARTESIAN_POINT ( 'NONE',  ( -17.99999999999999645, -24.16482700510260173, 20.67382249208304046 ) ) ;
#12250=CARTESIAN_POINT ( 'NONE',  ( -13.28918265808472299, -31.04416526290805933, 11.91992750791695777 ) ) ;
#12256=CARTESIAN_POINT ( 'NONE',  ( -16.64274437364856496, -26.51566270880199738, 17.82617750791695954 ) ) ;
#12271=CARTESIAN_POINT ( 'NONE',  ( -10.58745947852649927, -21.64274437364853654, 36.63867750791695954 ) ) ;
#12274=CARTESIAN_POINT ( 'NONE',  ( -9.999999999999994671, -24.16482700510257686, 16.07617750791695954 ) ) ;
#12279=CARTESIAN_POINT ( 'NONE',  ( -16.50457296725825174, -19.04416526290807354, 11.26757249208304046 ) ) ;
#12282=CARTESIAN_POINT ( 'NONE',  ( -12.31951028609536536, -25.35725562635139596, 13.23632249208304223 ) ) ;
#12298=CARTESIAN_POINT ( 'NONE',  ( -18.78091578003889950, -27.53959229564985378, 18.04492750791695954 ) ) ;
#12300=CARTESIAN_POINT ( 'NONE',  ( -17.35725562635140307, -28.41254052147349185, 25.04882249208304401 ) ) ;
#12302=CARTESIAN_POINT ( 'NONE',  ( -9.955834737091912245, -22.82508104294696594, 21.10742750791695599 ) ) ;
#12304=CARTESIAN_POINT ( 'NONE',  ( -11.46040770435012490, -27.78091578003888173, 16.73242750791695954 ) ) ;
#12316=CARTESIAN_POINT ( 'NONE',  ( -18.35725562635138886, -30.14459132904237393, 30.29882249208304401 ) ) ;
#12318=CARTESIAN_POINT ( 'NONE',  ( -10.58745947852648328, -26.35725562635138530, 7.986322492083041347 ) ) ;
#12320=CARTESIAN_POINT ( 'NONE',  ( -12.31951028609537602, -22.64274437364854364, 26.13867750791696309 ) ) ;
#12322=CARTESIAN_POINT ( 'NONE',  ( -12.95952864787948755, -30.95583473709188382, 19.14257249208303691 ) ) ;
#12338=CARTESIAN_POINT ( 'NONE',  ( -9.754982604823348780, -18.99630608921234654, 31.16992750791695954 ) ) ;
#12342=CARTESIAN_POINT ( 'NONE',  ( -18.04416526290808775, -23.36097942780924441, 15.64257249208304579 ) ) ;
#12343=CARTESIAN_POINT ( 'NONE',  ( -20.00369391078762860, -18.75498260482333279, 14.10742750791695777 ) ) ;
#12348=CARTESIAN_POINT ( 'NONE',  ( -15.63902057219076269, -20.95583473709189448, 19.79492750791695954 ) ) ;
#12368=CARTESIAN_POINT ( 'NONE',  ( -19.24771351637089367, -21.35725562635142438, 13.88867750791695954 ) ) ;
#12372=CARTESIAN_POINT ( 'NONE',  ( -11.21908421996106320, -27.53959229564982181, 13.45507249208304223 ) ) ;
#12373=CARTESIAN_POINT ( 'NONE',  ( -17.68048971390462754, -22.64274437364856496, 21.11132249208304401 ) ) ;
#12392=CARTESIAN_POINT ( 'NONE',  ( -19.95583473709191580, -22.49542703274176603, 18.91992750791694888 ) ) ;
#12394=CARTESIAN_POINT ( 'NONE',  ( -10.75228648362912232, -21.35725562635138530, 17.61132249208304401 ) ) ;
#12396=CARTESIAN_POINT ( 'NONE',  ( -12.64274437364855252, -28.41254052147347053, 16.95117750791695954 ) ) ;
#12399=CARTESIAN_POINT ( 'NONE',  ( -19.41254052147348830, -26.35725562635142083, 23.51367750791695954 ) ) ;
#12401=CARTESIAN_POINT ( 'NONE',  ( -18.78091578003892792, -20.46040770435013556, 26.58007249208304401 ) ) ;
#12412=CARTESIAN_POINT ( 'NONE',  ( -14.83517299489734853, -30.99999999999998224, 35.11132249208304046 ) ) ;
#12416=CARTESIAN_POINT ( 'NONE',  ( -19.95583473709190514, -25.50457296725823042, 9.955072492083040459 ) ) ;
#12418=CARTESIAN_POINT ( 'NONE',  ( -14.36097942780923731, -27.04416526290806999, 32.91992750791696665 ) ) ;
#12420=CARTESIAN_POINT ( 'NONE',  ( -21.95583473709189803, -26.04047135212049469, 25.70507249208304046 ) ) ;
#12437=CARTESIAN_POINT ( 'NONE',  ( -21.95583473709191580, -21.95952864787954084, 24.16992750791695954 ) ) ;
#12441=CARTESIAN_POINT ( 'NONE',  ( -13.64274437364857739, -21.31951028609534760, 27.67382249208304401 ) ) ;
#12442=CARTESIAN_POINT ( 'NONE',  ( -8.044165262908075320, -26.04047135212042718, 21.54492750791695599 ) ) ;
#12446=CARTESIAN_POINT ( 'NONE',  ( -13.64274437364856141, -26.68048971390460622, 22.20117750791696309 ) ) ;
#12461=CARTESIAN_POINT ( 'NONE',  ( -18.78091578003889950, -27.53959229564985378, 28.54492750791695954 ) ) ;
#12464=CARTESIAN_POINT ( 'NONE',  ( -20.04416526290809131, -22.82508104294699791, 31.39257249208304046 ) ) ;
#12465=CARTESIAN_POINT ( 'NONE',  ( -11.99999999999999289, -23.83517299489735564, 23.29882249208304046 ) ) ;
#12484=CARTESIAN_POINT ( 'NONE',  ( -20.04416526290808065, -25.17491895705300209, 18.48242750791695954 ) ) ;
#12487=CARTESIAN_POINT ( 'NONE',  ( -15.16482700510263371, -18.99999999999997868, 16.73632249208304401 ) ) ;
#12490=CARTESIAN_POINT ( 'NONE',  ( -10.58745947852649927, -21.64274437364853654, 15.63867750791695777 ) ) ;
#12493=CARTESIAN_POINT ( 'NONE',  ( -11.21908421996108984, -20.46040770435011069, 36.41992750791696665 ) ) ;
#12495=CARTESIAN_POINT ( 'NONE',  ( -10.58745947852648328, -26.35725562635138530, 28.98632249208304401 ) ) ;
#12506=CARTESIAN_POINT ( 'NONE',  ( -8.855408670957602979, -27.35725562635137820, 28.98632249208304401 ) ) ;
#12509=CARTESIAN_POINT ( 'NONE',  ( -16.50457296725825174, -19.04416526290807354, 16.51757249208304046 ) ) ;
#12512=CARTESIAN_POINT ( 'NONE',  ( -12.04416526290807887, -24.96867458239596260, 26.79492750791695954 ) ) ;
#12514=CARTESIAN_POINT ( 'NONE',  ( -7.955834737091903364, -25.71081734191518464, 18.26757249208304046 ) ) ;
#12533=CARTESIAN_POINT ( 'NONE',  ( -9.996306089212364299, -29.24501739517662813, 32.48242750791695244 ) ) ;
#12538=CARTESIAN_POINT ( 'NONE',  ( -12.31951028609536536, -25.35725562635139596, 34.23632249208304756 ) ) ;
#12539=CARTESIAN_POINT ( 'NONE',  ( -9.996306089212364299, -29.24501739517662813, 21.98242750791695599 ) ) ;
#12545=CARTESIAN_POINT ( 'NONE',  ( -12.48433729119798130, -25.64274437364855075, 27.01367750791695954 ) ) ;
#12555=FACE_OUTER_BOUND ( 'NONE', #17425, .T. ) ;
#12566=CARTESIAN_POINT ( 'NONE',  ( -19.95583473709191580, -22.49542703274176603, 34.66992750791694533 ) ) ;
#12569=VERTEX_POINT ( 'NONE', #1681 ) ;
#12570=CARTESIAN_POINT ( 'NONE',  ( -11.46040770435014977, -20.21908421996103655, 38.39257249208301914 ) ) ;
#12572=CARTESIAN_POINT ( 'NONE',  ( -15.96867458239599635, -21.04416526290806999, 37.51757249208305467 ) ) ;
#12589=CARTESIAN_POINT ( 'NONE',  ( -10.04416526290807710, -25.50457296725819489, 26.79492750791695954 ) ) ;
#12591=CARTESIAN_POINT ( 'NONE',  ( -20.04416526290809131, -22.82508104294699791, 26.14257249208303691 ) ) ;
#12593=CARTESIAN_POINT ( 'NONE',  ( -17.35725562635144215, -19.58745947852648683, 19.57617750791695954 ) ) ;
#12596=CARTESIAN_POINT ( 'NONE',  ( -11.21908421996108984, -20.46040770435011069, 25.91992750791695244 ) ) ;
#12598=CARTESIAN_POINT ( 'NONE',  ( -17.35725562635140307, -28.41254052147349185, 25.04882249208304401 ) ) ;
#12604=CLOSED_SHELL ( 'NONE', ( #6160, #19219, #15941, #17210, #14308 ) ) ;
#12606=CARTESIAN_POINT ( 'NONE',  ( -13.28918265808478694, -16.95583473709189093, 32.70507249208304756 ) ) ;
#12609=CARTESIAN_POINT ( 'NONE',  ( -17.51566270880201159, -22.35725562635141728, 24.38867750791696665 ) ) ;
#12611=CARTESIAN_POINT ( 'NONE',  ( -18.35725562635138886, -30.14459132904237393, 25.04882249208303691 ) ) ;
#12627=CARTESIAN_POINT ( 'NONE',  ( -21.99999999999999289, -23.83517299489739116, 34.45117750791695954 ) ) ;
#12631=CARTESIAN_POINT ( 'NONE',  ( -16.35725562635141372, -26.68048971390461332, 25.04882249208304401 ) ) ;
#12632=CARTESIAN_POINT ( 'NONE',  ( -18.64274437364853654, -29.97976432393976509, 12.57617750791695599 ) ) ;
#12637=CARTESIAN_POINT ( 'NONE',  ( -11.99999999999999289, -24.16482700510258752, 26.57617750791696309 ) ) ;
#12654=CARTESIAN_POINT ( 'NONE',  ( -17.35725562635144215, -19.58745947852648683, 35.32617750791695954 ) ) ;
#12656=EDGE_LOOP ( 'NONE', ( #4467, #5192, #13317 ) ) ;
#12658=CARTESIAN_POINT ( 'NONE',  ( -12.64274437364858628, -19.58745947852646552, 27.67382249208304046 ) ) ;
#12660=CARTESIAN_POINT ( 'NONE',  ( -17.07549068051208963, -26.31681416490115311, 30.51757249208304756 ) ) ;
#12676=CARTESIAN_POINT ( 'NONE',  ( -18.78091578003889950, -27.53959229564985378, 33.79492750791696665 ) ) ;
#12679=CARTESIAN_POINT ( 'NONE',  ( -13.82508104294702100, -18.95583473709188382, 27.45507249208304046 ) ) ;
#12681=CARTESIAN_POINT ( 'NONE',  ( -19.95583473709191580, -22.49542703274176603, 29.41992750791695599 ) ) ;
#12683=CARTESIAN_POINT ( 'NONE',  ( -17.35725562635144215, -19.58745947852648683, 30.07617750791695599 ) ) ;
#12685=CARTESIAN_POINT ( 'NONE',  ( -17.35725562635140307, -28.41254052147349185, 19.79882249208304046 ) ) ;
#12695=CARTESIAN_POINT ( 'NONE',  ( -14.03132541760401786, -21.04416526290806289, 25.48242750791696309 ) ) ;
#12698=CARTESIAN_POINT ( 'NONE',  ( -9.020235676060250896, -20.35725562635137820, 28.11132249208304046 ) ) ;
#12712=ADVANCED_BREP_SHAPE_REPRESENTATION ( '', ( #16836, #1791 ), #2725 ) ;
#12716=CARTESIAN_POINT ( 'NONE',  ( -7.999999999999996447, -24.16482700510256976, 31.82617750791695954 ) ) ;
#12720=CARTESIAN_POINT ( 'NONE',  ( -17.68048971390462754, -22.64274437364856496, 31.61132249208304401 ) ) ;
#12721=CARTESIAN_POINT ( 'NONE',  ( -11.64274437364854187, -30.14459132904234195, 37.95117750791695244 ) ) ;
#12728=CARTESIAN_POINT ( 'NONE',  ( -12.92450931948788906, -26.31681416490114245, 27.23242750791697020 ) ) ;
#12744=CARTESIAN_POINT ( 'NONE',  ( -10.04416526290807710, -25.50457296725819489, 32.04492750791695954 ) ) ;
#12748=CARTESIAN_POINT ( 'NONE',  ( -11.46040770435014977, -20.21908421996103655, 33.14257249208303335 ) ) ;
#12749=EDGE_CURVE ( 'NONE', #12569, #1158, #9966, .T. ) ;
#12752=CARTESIAN_POINT ( 'NONE',  ( -15.16482700510262482, -20.99999999999997513, 37.73632249208304756 ) ) ;
#12766=CARTESIAN_POINT ( 'NONE',  ( -10.75228648362910100, -26.64274437364854009, 27.01367750791695954 ) ) ;
#12768=CARTESIAN_POINT ( 'NONE',  ( -19.41254052147350961, -21.64274437364857562, 36.86132249208304046 ) ) ;
#12771=CARTESIAN_POINT ( 'NONE',  ( -13.49542703274178379, -19.04416526290806289, 25.48242750791694888 ) ) ;
#12773=CARTESIAN_POINT ( 'NONE',  ( -19.41254052147348830, -26.35725562635142083, 39.26367750791695954 ) ) ;
#12775=CARTESIAN_POINT ( 'NONE',  ( -13.49542703274174116, -28.95583473709188738, 19.14257249208303691 ) ) ;
#12786=CARTESIAN_POINT ( 'NONE',  ( -14.83517299489739649, -18.99999999999997868, -0.9863224920830417908 ) ) ;
#12788=CARTESIAN_POINT ( 'NONE',  ( -20.00369391078757886, -29.24501739517668142, 30.51757249208304401 ) ) ;
#12803=CARTESIAN_POINT ( 'NONE',  ( -13.28918265808478694, -16.95583473709189093, 6.455072492083038682 ) ) ;
#12809=CARTESIAN_POINT ( 'NONE',  ( -15.63902057219073605, -27.04416526290807710, 30.08007249208304401 ) ) ;
#12812=CARTESIAN_POINT ( 'NONE',  ( -12.95952864787955150, -17.04416526290805933, 30.73242750791696309 ) ) ;
#12835=CARTESIAN_POINT ( 'NONE',  ( -20.24501739517664234, -29.00369391078761439, 2.294927507916956433 ) ) ;
#12838=CARTESIAN_POINT ( 'NONE',  ( -10.75228648362912232, -21.35725562635138530, 33.36132249208304046 ) ) ;
#12842=CARTESIAN_POINT ( 'NONE',  ( -12.04416526290808420, -23.03132541760398766, 33.58007249208304756 ) ) ;
#12854=CARTESIAN_POINT ( 'NONE',  ( -9.955834737091912245, -22.82508104294696594, 31.60742750791695954 ) ) ;
#12864=CARTESIAN_POINT ( 'NONE',  ( -16.50457296725820555, -28.95583473709189448, 28.10742750791695954 ) ) ;
#12866=CARTESIAN_POINT ( 'NONE',  ( -14.83517299489735741, -28.99999999999998224, 29.86132249208304401 ) ) ;
#12871=CARTESIAN_POINT ( 'NONE',  ( -20.04416526290808065, -25.17491895705300209, 34.23242750791695954 ) ) ;
#12873=CARTESIAN_POINT ( 'NONE',  ( -14.83517299489739649, -18.99999999999997868, 30.51367750791695954 ) ) ;
#12887=CARTESIAN_POINT ( 'NONE',  ( -10.75228648362910100, -26.64274437364854009, 6.013677507916958653 ) ) ;
#12889=CARTESIAN_POINT ( 'NONE',  ( -12.95952864787948755, -30.95583473709188382, 29.64257249208304401 ) ) ;
#12903=CARTESIAN_POINT ( 'NONE',  ( -8.855408670957602979, -27.35725562635137820, 7.986322492083039570 ) ) ;
#12908=CARTESIAN_POINT ( 'NONE',  ( -12.48433729119798130, -25.64274437364855075, 6.013677507916959541 ) ) ;
#12909=CARTESIAN_POINT ( 'NONE',  ( -11.35725562635144925, -18.02023567606020293, 30.95117750791695954 ) ) ;
#12929=CARTESIAN_POINT ( 'NONE',  ( -20.97976432393977575, -20.35725562635143504, 8.638677507916955989 ) ) ;
#12932=CARTESIAN_POINT ( 'NONE',  ( -19.99999999999999645, -24.16482700510261949, 41.67382249208304046 ) ) ;
#12936=CARTESIAN_POINT ( 'NONE',  ( -13.64274437364857739, -21.31951028609534760, 38.17382249208304046 ) ) ;
#12944=CARTESIAN_POINT ( 'NONE',  ( -13.82508104294698192, -29.04416526290806644, 27.66992750791695244 ) ) ;
#12951=CARTESIAN_POINT ( 'NONE',  ( -18.35725562635138886, -30.14459132904237393, 35.54882249208304046 ) ) ;
#12952=CARTESIAN_POINT ( 'NONE',  ( -14.83517299489739649, -18.99999999999997868, 30.51367750791695954 ) ) ;
#12954=CARTESIAN_POINT ( 'NONE',  ( -16.50457296725825174, -19.04416526290807354, 32.26757249208304046 ) ) ;
#12961=CARTESIAN_POINT ( 'NONE',  ( -19.41254052147348830, -26.35725562635142083, 23.51367750791695954 ) ) ;
#12976=CARTESIAN_POINT ( 'NONE',  ( -19.24771351637089367, -21.35725562635142438, 3.388677507916958653 ) ) ;
#12978=CARTESIAN_POINT ( 'NONE',  ( -21.95583473709189803, -26.04047135212049469, 36.20507249208304046 ) ) ;
#12991=CARTESIAN_POINT ( 'NONE',  ( -8.044165262908093084, -21.95952864787946979, 2.080072492083039126 ) ) ;
#12999=CARTESIAN_POINT ( 'NONE',  ( -13.35725562635141195, -26.51566270880198672, 39.92382249208304756 ) ) ;
#13000=CARTESIAN_POINT ( 'NONE',  ( -20.97976432393977575, -20.35725562635143504, 29.63867750791695954 ) ) ;
#13022=CARTESIAN_POINT ( 'NONE',  ( -20.04416526290808065, -25.17491895705300209, 39.48242750791695244 ) ) ;
#13025=CARTESIAN_POINT ( 'NONE',  ( -17.99999999999999645, -24.16482700510260173, 10.17382249208304223 ) ) ;
#13030=CARTESIAN_POINT ( 'NONE',  ( -16.64274437364856496, -26.51566270880199738, 2.076177507916959986 ) ) ;
#13039=CARTESIAN_POINT ( 'NONE',  ( -19.41254052147348830, -26.35725562635142083, 28.76367750791695954 ) ) ;
#13041=CARTESIAN_POINT ( 'NONE',  ( -16.17491895705301275, -18.95583473709189803, 4.044927507916959541 ) ) ;
#13044=CARTESIAN_POINT ( 'NONE',  ( -17.35725562635140307, -28.41254052147349185, 9.298822492083040459 ) ) ;
#13045=CARTESIAN_POINT ( 'NONE',  ( -8.044165262908075320, -26.04047135212042718, 0.5449275079169564329 ) ) ;
#13049=CARTESIAN_POINT ( 'NONE',  ( -15.16482700510262482, -20.99999999999997513, 11.48632249208304223 ) ) ;
#13053=CARTESIAN_POINT ( 'NONE',  ( -19.99999999999999645, -23.83517299489738051, 34.45117750791696665 ) ) ;
#13058=CARTESIAN_POINT ( 'NONE',  ( -12.35725562635140307, -28.24771351637085459, 39.92382249208304046 ) ) ;
#13068=CARTESIAN_POINT ( 'NONE',  ( -9.999999999999994671, -24.16482700510257686, 0.3261775079169582647 ) ) ;
#13069=CARTESIAN_POINT ( 'NONE',  ( -20.04416526290808065, -25.17491895705300209, 2.732427507916957765 ) ) ;
#13071=CARTESIAN_POINT ( 'NONE',  ( -18.35725562635138886, -30.14459132904237393, 30.29882249208304401 ) ) ;
#13074=CARTESIAN_POINT ( 'NONE',  ( -17.07549068051210739, -21.68318583509881847, 35.10742750791696665 ) ) ;
#13075=CARTESIAN_POINT ( 'NONE',  ( -12.64274437364855252, -28.41254052147347053, 1.201177507916958431 ) ) ;
#13089=CARTESIAN_POINT ( 'NONE',  ( -7.955834737091903364, -25.71081734191518464, 7.767572492083039570 ) ) ;
#13094=CARTESIAN_POINT ( 'NONE',  ( -17.51566270880199738, -25.64274437364856496, 41.23632249208304756 ) ) ;
#13096=CARTESIAN_POINT ( 'NONE',  ( -9.020235676060220698, -27.64274437364852588, 32.26367750791695244 ) ) ;
#13119=CARTESIAN_POINT ( 'NONE',  ( -7.955834737091916686, -22.28918265808470522, 5.357427507916955989 ) ) ;
#13122=CARTESIAN_POINT ( 'NONE',  ( -17.99999999999999645, -24.16482700510260173, 4.923822492083043123 ) ) ;
#13127=CARTESIAN_POINT ( 'NONE',  ( -17.95583473709191580, -23.03132541760400898, 3.169927507916960874 ) ) ;
#13140=CARTESIAN_POINT ( 'NONE',  ( -12.64274437364855252, -28.41254052147347053, 22.20117750791695599 ) ) ;
#13143=CARTESIAN_POINT ( 'NONE',  ( -17.64274437364855430, -28.24771351637087236, 2.076177507916958209 ) ) ;
#13148=CARTESIAN_POINT ( 'NONE',  ( -14.83517299489734853, -30.99999999999998224, 40.36132249208304046 ) ) ;
#13149=CARTESIAN_POINT ( 'NONE',  ( -7.999999999999996447, -24.16482700510256976, 5.576177507916956877 ) ) ;
#13152=CARTESIAN_POINT ( 'NONE',  ( -17.68048971390462754, -22.64274437364856496, 5.361322492083044011 ) ) ;
#13157=CARTESIAN_POINT ( 'NONE',  ( -16.17491895705301275, -18.95583473709189803, 40.79492750791695954 ) ) ;
#13162=CARTESIAN_POINT ( 'NONE',  ( -17.35725562635140307, -28.41254052147349185, 35.54882249208304046 ) ) ;
#13173=CARTESIAN_POINT ( 'NONE',  ( -9.955834737091912245, -22.82508104294696594, 10.60742750791695777 ) ) ;
#13174=CARTESIAN_POINT ( 'NONE',  ( -13.64274437364856141, -26.68048971390460622, 37.95117750791695244 ) ) ;
#13177=CARTESIAN_POINT ( 'NONE',  ( -9.999999999999994671, -23.83517299489734143, 7.548822492083041347 ) ) ;
#13180=CARTESIAN_POINT ( 'NONE',  ( -16.64274437364856496, -26.51566270880199738, 38.82617750791695954 ) ) ;
#13181=CARTESIAN_POINT ( 'NONE',  ( -13.82508104294698015, -29.04416526290806289, 6.669927507916956877 ) ) ;
#13194=CARTESIAN_POINT ( 'NONE',  ( -9.996306089212364299, -29.24501739517662813, 37.73242750791695244 ) ) ;
#13195=CARTESIAN_POINT ( 'NONE',  ( -15.16482700510263371, -18.99999999999997868, 0.9863224920830410136 ) ) ;
#13198=CARTESIAN_POINT ( 'NONE',  ( -12.04416526290807887, -24.96867458239596260, 0.5449275079169599856 ) ) ;
#13199=CARTESIAN_POINT ( 'NONE',  ( -18.35725562635138886, -30.14459132904237393, 9.298822492083038682 ) ) ;
#13221=CARTESIAN_POINT ( 'NONE',  ( -14.83517299489740715, -16.99999999999997868, -0.9863224920830435671 ) ) ;
#13225=CARTESIAN_POINT ( 'NONE',  ( -17.51566270880199738, -25.64274437364856496, 4.486322492083042235 ) ) ;
#13228=CARTESIAN_POINT ( 'NONE',  ( -11.99999999999999289, -24.16482700510258752, 0.3261775079169599856 ) ) ;
#13239=CARTESIAN_POINT ( 'NONE',  ( -18.78091578003889950, -27.53959229564985378, 28.54492750791695954 ) ) ;
#13241=CARTESIAN_POINT ( 'NONE',  ( -18.53959229564986799, -20.21908421996107563, 8.857427507916957765 ) ) ;
#13244=CARTESIAN_POINT ( 'NONE',  ( -18.64274437364860049, -18.02023567606023491, 42.54882249208304046 ) ) ;
#13245=CARTESIAN_POINT ( 'NONE',  ( -7.955834737091916686, -22.28918265808470522, 5.357427507916955989 ) ) ;
#13248=CARTESIAN_POINT ( 'NONE',  ( -16.17491895705296656, -29.04416526290807710, 40.58007249208304046 ) ) ;
#13251=CARTESIAN_POINT ( 'NONE',  ( -10.27562634311943057, -22.24032068463715106, -4.119453415227824499E-17 ) ) ;
#13253=CARTESIAN_POINT ( 'NONE',  ( -19.41254052147348830, -26.35725562635142083, 39.26367750791695954 ) ) ;
#13257=CARTESIAN_POINT ( 'NONE',  ( -19.41254052147350961, -21.64274437364857562, 42.11132249208304046 ) ) ;
#13264=CARTESIAN_POINT ( 'NONE',  ( -19.24771351637089367, -21.35725562635142438, 3.388677507916958653 ) ) ;
#13266=CARTESIAN_POINT ( 'NONE',  ( -16.50457296725820555, -28.95583473709189448, 17.60742750791695599 ) ) ;
#13268=CARTESIAN_POINT ( 'NONE',  ( -16.50457296725825174, -19.04416526290807354, 6.017572492083042235 ) ) ;
#13270=CARTESIAN_POINT ( 'NONE',  ( -14.36097942780923731, -27.04416526290806999, 38.16992750791696665 ) ) ;
#13271=CARTESIAN_POINT ( 'NONE',  ( -12.35725562635143682, -19.75228648362908501, 9.951177507916959541 ) ) ;
#13283=CARTESIAN_POINT ( 'NONE',  ( -12.95952864787948755, -30.95583473709188382, 19.14257249208303691 ) ) ;
#13284=FILL_AREA_STYLE_COLOUR ( '', #16189 ) ;
#13288=CARTESIAN_POINT ( 'NONE',  ( -18.04416526290808775, -23.36097942780924441, 41.89257249208304046 ) ) ;
#13290=CARTESIAN_POINT ( 'NONE',  ( -14.83517299489734853, -30.99999999999998224, 8.861322492083038682 ) ) ;
#13312=VERTEX_POINT ( 'NONE', #9459 ) ;
#13313=CARTESIAN_POINT ( 'NONE',  ( -8.855408670957631401, -20.64274437364852943, 20.88867750791695954 ) ) ;
#13317=ORIENTED_EDGE ( 'NONE', *, *, #3894, .F. ) ;
#13318=CARTESIAN_POINT ( 'NONE',  ( -13.35725562635141195, -26.51566270880198672, 3.173822492083044011 ) ) ;
#13323=CARTESIAN_POINT ( 'NONE',  ( -12.92450931948788906, -26.31681416490114245, 6.232427507916960430 ) ) ;
#13329=PRODUCT_DEFINITION_SHAPE ( 'NONE', 'NONE',  #13627 ) ;
#13339=CARTESIAN_POINT ( 'NONE',  ( -18.53959229564986799, -20.21908421996107563, 3.607427507916956877 ) ) ;
#13347=CARTESIAN_POINT ( 'NONE',  ( -18.78091578003892081, -20.46040770435013556, 5.580072492083041347 ) ) ;
#13348=CARTESIAN_POINT ( 'NONE',  ( -12.95952864787955150, -17.04416526290805933, -0.7675724920830436782 ) ) ;
#13351=CARTESIAN_POINT ( 'NONE',  ( -17.07549068051208963, -26.31681416490115311, 4.267572492083044011 ) ) ;
#13354=CARTESIAN_POINT ( 'NONE',  ( -12.14758986593398404, -18.81472126757313390, 5.414424919715185431E-14 ) ) ;
#13356=CARTESIAN_POINT ( 'NONE',  ( -19.24771351637089367, -21.35725562635142438, 40.13867750791695954 ) ) ;
#13364=( NAMED_UNIT ( * ) SI_UNIT ( $, .STERADIAN. ) SOLID_ANGLE_UNIT ( ) );
#13369=CARTESIAN_POINT ( 'NONE',  ( -13.82508104294698192, -29.04416526290806644, 1.419927507916958209 ) ) ;
#13370=CARTESIAN_POINT ( 'NONE',  ( -18.53959229564986799, -20.21908421996107563, 14.10742750791695777 ) ) ;
#13372=CARTESIAN_POINT ( 'NONE',  ( -13.49542703274174116, -28.95583473709188738, 8.642572492083040459 ) ) ;
#13374=CARTESIAN_POINT ( 'NONE',  ( -16.17491895705301275, -18.95583473709189803, 4.044927507916959541 ) ) ;
#13386=CARTESIAN_POINT ( 'NONE',  ( -11.35725562635139418, -29.97976432393972601, 13.67382249208304046 ) ) ;
#13390=CARTESIAN_POINT ( 'NONE',  ( -13.35725562635142794, -21.48433729119796709, 20.45117750791696309 ) ) ;
#13392=CARTESIAN_POINT ( 'NONE',  ( -18.64274437364860049, -18.02023567606023491, 5.798822492083038682 ) ) ;
#13410=CARTESIAN_POINT ( 'NONE',  ( -20.97976432393977575, -20.35725562635143504, 19.13867750791695954 ) ) ;
#13415=CARTESIAN_POINT ( 'NONE',  ( -12.31951028609536536, -25.35725562635139596, 23.73632249208304401 ) ) ;
#13420=CARTESIAN_POINT ( 'NONE',  ( -17.99999999999999645, -23.83517299489736985, 2.951177507916960430 ) ) ;
#13433=CARTESIAN_POINT ( 'NONE',  ( -19.41254052147348830, -26.35725562635142083, 39.26367750791695954 ) ) ;
#13436=CARTESIAN_POINT ( 'NONE',  ( -15.16482700510259640, -28.99999999999998224, 17.38867750791695599 ) ) ;
#13440=CARTESIAN_POINT ( 'NONE',  ( -18.78091578003892081, -20.46040770435013556, 21.33007249208303691 ) ) ;
#13445=CARTESIAN_POINT ( 'NONE',  ( -12.92450931948790149, -21.68318583509881137, 6.892572492083043123 ) ) ;
#13469=CARTESIAN_POINT ( 'NONE',  ( -11.21908421996108629, -20.46040770435011069, 4.919927507916955989 ) ) ;
#13470=CARTESIAN_POINT ( 'NONE',  ( -17.64274437364855430, -28.24771351637087236, 17.82617750791695599 ) ) ;
#13472=CARTESIAN_POINT ( 'NONE',  ( -19.24771351637086880, -26.64274437364857206, 9.736322492083042235 ) ) ;
#13476=CARTESIAN_POINT ( 'NONE',  ( -16.35725562635142794, -21.31951028609535470, 40.57617750791696665 ) ) ;
#13479=CARTESIAN_POINT ( 'NONE',  ( -10.75228648362910100, -26.64274437364854009, 6.013677507916958653 ) ) ;
#13492=CARTESIAN_POINT ( 'NONE',  ( -20.24501739517669563, -18.99630608921239627, 21.33007249208303691 ) ) ;
#13497=CARTESIAN_POINT ( 'NONE',  ( -17.31681416490115311, -26.07549068051209318, 18.04492750791696309 ) ) ;
#13499=CARTESIAN_POINT ( 'NONE',  ( -16.71081734191520596, -31.04416526290808065, 3.830072492083039126 ) ) ;
#13519=CARTESIAN_POINT ( 'NONE',  ( -16.71081734191527346, -16.95583473709190159, 14.54492750791695421 ) ) ;
#13524=CARTESIAN_POINT ( 'NONE',  ( -17.68048971390462754, -22.64274437364856496, 21.11132249208304401 ) ) ;
#13530=CARTESIAN_POINT ( 'NONE',  ( -14.03132541760401786, -21.04416526290806289, 14.98242750791695954 ) ) ;
#13542=CARTESIAN_POINT ( 'NONE',  ( -10.75228648362910100, -26.64274437364854009, 11.26367750791695777 ) ) ;
#13545=CARTESIAN_POINT ( 'NONE',  ( -10.04416526290808953, -22.49542703274172695, 23.08007249208303335 ) ) ;
#13547=CARTESIAN_POINT ( 'NONE',  ( -15.16482700510262482, -20.99999999999997513, 16.73632249208304046 ) ) ;
#13550=CARTESIAN_POINT ( 'NONE',  ( -10.37592340745185382, -20.82129991144855907, 3.747711961066386859E-16 ) ) ;
#13558=FILL_AREA_STYLE ('',( #17982 ) ) ;
#13563=CARTESIAN_POINT ( 'NONE',  ( -14.83517299489739649, -18.99999999999997868, 14.76367750791695777 ) ) ;
#13565=CARTESIAN_POINT ( 'NONE',  ( -12.35725562635143682, -19.75228648362908501, 15.20117750791695777 ) ) ;
#13568=CARTESIAN_POINT ( 'NONE',  ( -17.64274437364858983, -19.75228648362910633, 5.798822492083041347 ) ) ;
#13570=CARTESIAN_POINT ( 'NONE',  ( -12.35725562635143682, -19.75228648362908501, -0.5488224920830419018 ) ) ;
#13572=CARTESIAN_POINT ( 'NONE',  ( -18.53959229564986799, -20.21908421996107563, 24.60742750791695954 ) ) ;
#13585=CARTESIAN_POINT ( 'NONE',  ( -18.35725562635138886, -30.14459132904237393, 25.04882249208303691 ) ) ;
#13590=CARTESIAN_POINT ( 'NONE',  ( -17.07549068051210739, -21.68318583509881847, 8.857427507916959541 ) ) ;
#13592=CARTESIAN_POINT ( 'NONE',  ( -8.044165262908093084, -21.95952864787946979, 2.080072492083039126 ) ) ;
#13598=STYLED_ITEM ( 'NONE', ( #17712 ), #12712 ) ;
#13603=CARTESIAN_POINT ( 'NONE',  ( -10.57758699569699523, -22.20123138602766133, 1.196196559315024355E-16 ) ) ;
#13612=CARTESIAN_POINT ( 'NONE',  ( -20.24501739517664234, -29.00369391078761439, 12.79492750791695599 ) ) ;
#13616=CARTESIAN_POINT ( 'NONE',  ( -16.35725562635141372, -26.68048971390461332, 19.79882249208304046 ) ) ;
#13621=CARTESIAN_POINT ( 'NONE',  ( -13.35725562635142794, -21.48433729119796709, 15.20117750791696132 ) ) ;
#13627=PRODUCT_DEFINITION ( 'UNKNOWN', '', #10149, #1397 ) ;
#13635=CARTESIAN_POINT ( 'NONE',  ( -19.24771351637089367, -21.35725562635142438, 40.13867750791695954 ) ) ;
#13637=CARTESIAN_POINT ( 'NONE',  ( -9.955834737091912245, -22.82508104294696594, 21.10742750791695599 ) ) ;
#13640=CARTESIAN_POINT ( 'NONE',  ( -19.99999999999999645, -24.16482700510261949, 15.42382249208304046 ) ) ;
#13644=CARTESIAN_POINT ( 'NONE',  ( -16.35725562635141372, -26.68048971390461332, 25.04882249208304401 ) ) ;
#13647=CARTESIAN_POINT ( 'NONE',  ( -10.15500167420339928, -22.00430890708279108, 4.586222366068608161E-17 ) ) ;
#13652=DIRECTION ( 'NONE',  ( -0.9863224920830415687, -5.704848896154130918E-15, -0.1648270051026189120 ) ) ;
#13662=CARTESIAN_POINT ( 'NONE',  ( -11.46040770435012668, -27.78091578003887463, 11.48242750791695954 ) ) ;
#13665=CARTESIAN_POINT ( 'NONE',  ( -12.35725562635140307, -28.24771351637085459, 18.92382249208304401 ) ) ;
#13668=CARTESIAN_POINT ( 'NONE',  ( -11.21908421996108629, -20.46040770435011069, 10.16992750791695244 ) ) ;
#13671=CARTESIAN_POINT ( 'NONE',  ( -12.35725562635143682, -19.75228648362908501, 15.20117750791695777 ) ) ;
#13685=CARTESIAN_POINT ( 'NONE',  ( -18.35725562635138886, -30.14459132904237393, 19.79882249208303691 ) ) ;
#13687=CARTESIAN_POINT ( 'NONE',  ( -19.41254052147350961, -21.64274437364857562, 5.361322492083041347 ) ) ;
#13690=CARTESIAN_POINT ( 'NONE',  ( -12.68318583509884157, -21.92450931948787485, 10.16992750791695954 ) ) ;
#13692=CARTESIAN_POINT ( 'NONE',  ( -13.28918265808478694, -16.95583473709189093, 16.95507249208304046 ) ) ;
#13712=CARTESIAN_POINT ( 'NONE',  ( -18.35725562635144925, -17.85540867095761186, 19.57617750791695954 ) ) ;
#13713=CARTESIAN_POINT ( 'NONE',  ( 0.000000000000000000, 0.000000000000000000, 0.000000000000000000 ) ) ;
#13716=CARTESIAN_POINT ( 'NONE',  ( -12.31951028609536536, -25.35725562635139596, 13.23632249208304223 ) ) ;
#13717=CARTESIAN_POINT ( 'NONE',  ( -21.99999999999999289, -23.83517299489739116, 8.201177507916955989 ) ) ;
#13721=CARTESIAN_POINT ( 'NONE',  ( -17.68048971390461688, -25.35725562635141372, 13.01367750791696132 ) ) ;
#13738=CARTESIAN_POINT ( 'NONE',  ( -10.04416526290807710, -25.50457296725819489, 16.29492750791695954 ) ) ;
#13741=CARTESIAN_POINT ( 'NONE',  ( -20.04416526290809131, -22.82508104294699791, 20.89257249208303691 ) ) ;
#13744=CARTESIAN_POINT ( 'NONE',  ( -14.03132541760400009, -26.95583473709189448, 19.14257249208304401 ) ) ;
#13764=CARTESIAN_POINT ( 'NONE',  ( -17.64274437364855430, -28.24771351637087236, 17.82617750791695599 ) ) ;
#13767=CARTESIAN_POINT ( 'NONE',  ( -19.95583473709190514, -25.50457296725822687, 20.45507249208304401 ) ) ;
#13770=CARTESIAN_POINT ( 'NONE',  ( -16.50457296725820555, -28.95583473709189448, 22.85742750791695954 ) ) ;
#13772=CARTESIAN_POINT ( 'NONE',  ( -19.99999999999999645, -23.83517299489738051, 18.70117750791695954 ) ) ;
#13785=CARTESIAN_POINT ( 'NONE',  ( -7.999999999999996447, -23.83517299489733432, 33.79882249208304046 ) ) ;
#13787=CARTESIAN_POINT ( 'NONE',  ( -19.24771351637086880, -26.64274437364857206, 9.736322492083042235 ) ) ;
#13789=CARTESIAN_POINT ( 'NONE',  ( -13.35725562635142794, -21.48433729119796709, 36.20117750791695954 ) ) ;
#13791=CARTESIAN_POINT ( 'NONE',  ( -8.044165262908093084, -21.95952864787946979, 23.08007249208303691 ) ) ;
#13811=CARTESIAN_POINT ( 'NONE',  ( -14.83517299489740715, -16.99999999999997868, 25.26367750791695954 ) ) ;
#13817=CARTESIAN_POINT ( 'NONE',  ( -17.51566270880199738, -25.64274437364856496, 20.23632249208304401 ) ) ;
#13818=CARTESIAN_POINT ( 'NONE',  ( -21.14459132904236327, -27.35725562635143149, 23.51367750791695599 ) ) ;
#13825=CARTESIAN_POINT ( 'NONE',  ( -11.95583473709191047, -23.36097942780921954, 15.85742750791696309 ) ) ;
#13843=CARTESIAN_POINT ( 'NONE',  ( -14.83517299489739649, -18.99999999999997868, 20.01367750791695954 ) ) ;
#13846=CARTESIAN_POINT ( 'NONE',  ( -10.58745947852648328, -26.35725562635138530, 18.48632249208304401 ) ) ;
#13848=CARTESIAN_POINT ( 'NONE',  ( -11.99999999999999289, -23.83517299489735564, 12.79882249208304223 ) ) ;
#13865=CARTESIAN_POINT ( 'NONE',  ( -10.75228648362910100, -26.64274437364854009, 16.51367750791695954 ) ) ;
#13867=CARTESIAN_POINT ( 'NONE',  ( -12.64274437364858628, -19.58745947852646552, 17.17382249208304401 ) ) ;
#13870=CARTESIAN_POINT ( 'NONE',  ( -19.99999999999999645, -23.83517299489738051, 13.45117750791695777 ) ) ;
#13872=CARTESIAN_POINT ( 'NONE',  ( -10.75228648362910100, -26.64274437364854009, 21.76367750791695599 ) ) ;
#13884=CARTESIAN_POINT ( 'NONE',  ( -13.28918265808478694, -16.95583473709189093, 27.45507249208304046 ) ) ;
#13885=CARTESIAN_POINT ( 'NONE',  ( -17.64274437364858983, -19.75228648362910633, 11.04882249208304046 ) ) ;
#13887=CARTESIAN_POINT ( 'NONE',  ( -14.83517299489738761, -20.99999999999997513, 30.51367750791696309 ) ) ;
#13889=CARTESIAN_POINT ( 'NONE',  ( -22.04416526290809486, -22.28918265808477628, 20.89257249208303691 ) ) ;
#13905=CARTESIAN_POINT ( 'NONE',  ( -20.00369391078762860, -18.75498260482333279, 35.10742750791695244 ) ) ;
#13909=CARTESIAN_POINT ( 'NONE',  ( -17.99999999999999645, -24.16482700510260173, 36.42382249208304756 ) ) ;
#13912=CARTESIAN_POINT ( 'NONE',  ( -7.999999999999996447, -24.16482700510256976, 21.32617750791695599 ) ) ;
#13916=CARTESIAN_POINT ( 'NONE',  ( -12.48433729119798130, -25.64274437364855075, 16.51367750791695954 ) ) ;
#13938=CARTESIAN_POINT ( 'NONE',  ( -16.17491895705301275, -18.95583473709189803, 25.04492750791695954 ) ) ;
#13941=CARTESIAN_POINT ( 'NONE',  ( -17.35725562635140307, -28.41254052147349185, 35.54882249208304046 ) ) ;
#13943=CARTESIAN_POINT ( 'NONE',  ( -17.99999999999999645, -24.16482700510260173, 20.67382249208304046 ) ) ;
#13962=CARTESIAN_POINT ( 'NONE',  ( -12.35725562635143682, -19.75228648362908501, 20.45117750791695954 ) ) ;
#13964=CARTESIAN_POINT ( 'NONE',  ( -13.49542703274174116, -28.95583473709188738, 13.89257249208303691 ) ) ;
#13966=CARTESIAN_POINT ( 'NONE',  ( -9.999999999999994671, -24.16482700510257686, 16.07617750791695954 ) ) ;
#13969=CARTESIAN_POINT ( 'NONE',  ( -13.49542703274178201, -19.04416526290806289, 14.98242750791695777 ) ) ;
#13971=CARTESIAN_POINT ( 'NONE',  ( -9.999999999999994671, -23.83517299489734143, 23.29882249208304046 ) ) ;
#13982=CARTESIAN_POINT ( 'NONE',  ( -17.04047135212050890, -17.04416526290807710, 27.01757249208303691 ) ) ;
#13985=CARTESIAN_POINT ( 'NONE',  ( -20.04416526290809131, -22.82508104294700502, 15.64257249208304223 ) ) ;
#13987=CARTESIAN_POINT ( 'NONE',  ( -15.96867458239597326, -26.95583473709190159, 28.10742750791695954 ) ) ;
#13989=CARTESIAN_POINT ( 'NONE',  ( -20.00369391078757886, -29.24501739517668142, 25.26757249208304401 ) ) ;
#14003=CARTESIAN_POINT ( 'NONE',  ( -9.754982604823348780, -18.99630608921234654, 25.91992750791695599 ) ) ;
#14008=CARTESIAN_POINT ( 'NONE',  ( -15.96867458239599635, -21.04416526290806999, 37.51757249208305467 ) ) ;
#14009=CARTESIAN_POINT ( 'NONE',  ( -16.71081734191527346, -16.95583473709190159, 14.54492750791695421 ) ) ;
#14014=CARTESIAN_POINT ( 'NONE',  ( -12.68318583509884157, -21.92450931948787485, 25.91992750791696309 ) ) ;
#14032=CARTESIAN_POINT ( 'NONE',  ( -17.35725562635144215, -19.58745947852648683, 30.07617750791695599 ) ) ;
#14036=CARTESIAN_POINT ( 'NONE',  ( -18.53959229564982536, -27.78091578003890660, 25.26757249208304401 ) ) ;
#14038=CARTESIAN_POINT ( 'NONE',  ( -15.96867458239599635, -21.04416526290806999, 32.26757249208305467 ) ) ;
#14056=CARTESIAN_POINT ( 'NONE',  ( -16.17491895705301275, -18.95583473709189803, 30.29492750791695244 ) ) ;
#14058=CARTESIAN_POINT ( 'NONE',  ( -10.75228648362912232, -21.35725562635138530, 12.36132249208304046 ) ) ;
#14062=CARTESIAN_POINT ( 'NONE',  ( -11.21908421996108629, -20.46040770435011069, 20.66992750791695244 ) ) ;
#14066=CARTESIAN_POINT ( 'NONE',  ( -15.16482700510259640, -28.99999999999998224, 33.13867750791696665 ) ) ;
#14068=CARTESIAN_POINT ( 'NONE',  ( -11.46040770435015332, -20.21908421996104011, 22.64257249208304046 ) ) ;
#14078=CARTESIAN_POINT ( 'NONE',  ( -8.044165262908093084, -21.95952864787946979, 28.33007249208304756 ) ) ;
#14080=CARTESIAN_POINT ( 'NONE',  ( -10.75228648362912232, -21.35725562635138530, 7.111322492083040459 ) ) ;
#14082=CARTESIAN_POINT ( 'NONE',  ( -11.95583473709191047, -23.36097942780921954, 31.60742750791695599 ) ) ;
#14086=CARTESIAN_POINT ( 'NONE',  ( -20.24501739517669563, -18.99630608921239627, 21.33007249208303691 ) ) ;
#14103=CARTESIAN_POINT ( 'NONE',  ( -8.044165262908075320, -26.04047135212042718, 26.79492750791695954 ) ) ;
#14109=CARTESIAN_POINT ( 'NONE',  ( -14.36097942780925685, -20.95583473709189093, 27.45507249208304756 ) ) ;
#14110=CARTESIAN_POINT ( 'NONE',  ( -7.955834737091916686, -22.28918265808470522, 15.85742750791695954 ) ) ;
#14116=CARTESIAN_POINT ( 'NONE',  ( -18.04416526290808420, -24.63902057219074493, 23.73242750791696665 ) ) ;
#14133=CARTESIAN_POINT ( 'NONE',  ( -12.64274437364855252, -28.41254052147347053, 27.45117750791695954 ) ) ;
#14137=CARTESIAN_POINT ( 'NONE',  ( -10.04416526290808953, -22.49542703274172695, 38.83007249208302625 ) ) ;
#14139=CARTESIAN_POINT ( 'NONE',  ( -11.95583473709190514, -24.63902057219072361, 39.26757249208304756 ) ) ;
#14157=CARTESIAN_POINT ( 'NONE',  ( -9.955834737091912245, -22.82508104294696594, 26.35742750791695954 ) ) ;
#14161=CARTESIAN_POINT ( 'NONE',  ( -16.50457296725825174, -19.04416526290807354, 37.51757249208304046 ) ) ;
#14163=CARTESIAN_POINT ( 'NONE',  ( -19.41254052147348830, -26.35725562635142083, 28.76367750791695954 ) ) ;
#14165=CARTESIAN_POINT ( 'NONE',  ( -9.955834737091912245, -22.82508104294696238, 26.35742750791695599 ) ) ;
#14167=CARTESIAN_POINT ( 'NONE',  ( -18.53959229564983247, -27.78091578003891016, 25.26757249208304401 ) ) ;
#14181=CARTESIAN_POINT ( 'NONE',  ( -12.68318583509884157, -21.92450931948787485, 25.91992750791696309 ) ) ;
#14183=CARTESIAN_POINT ( 'NONE',  ( -21.14459132904239169, -20.64274437364858628, 36.86132249208304046 ) ) ;
#14197=CARTESIAN_POINT ( 'NONE',  ( -8.855408670957631401, -20.64274437364852943, 36.63867750791695244 ) ) ;
#14202=CARTESIAN_POINT ( 'NONE',  ( -16.35725562635141372, -26.68048971390461332, 30.29882249208304401 ) ) ;
#14204=CARTESIAN_POINT ( 'NONE',  ( -7.955834737091916686, -22.28918265808470522, 21.10742750791695954 ) ) ;
#14209=CARTESIAN_POINT ( 'NONE',  ( -12.48433729119798130, -25.64274437364855075, 32.26367750791695954 ) ) ;
#14224=VERTEX_POINT ( 'NONE', #18060 ) ;
#14225=CARTESIAN_POINT ( 'NONE',  ( -10.58745947852649927, -21.64274437364853654, 36.63867750791695954 ) ) ;
#14229=CARTESIAN_POINT ( 'NONE',  ( -19.24771351637086880, -26.64274437364857206, 30.73632249208304401 ) ) ;
#14231=CARTESIAN_POINT ( 'NONE',  ( -13.35725562635141195, -26.51566270880198672, 34.67382249208304756 ) ) ;
#14246=CARTESIAN_POINT ( 'NONE',  ( -12.64274437364855252, -28.41254052147347053, 32.70117750791696665 ) ) ;
#14248=CARTESIAN_POINT ( 'NONE',  ( -10.75228648362912232, -21.35725562635138530, 38.61132249208304046 ) ) ;
#14251=CARTESIAN_POINT ( 'NONE',  ( -17.64274437364855430, -28.24771351637087236, 28.32617750791695954 ) ) ;
#14253=CARTESIAN_POINT ( 'NONE',  ( -18.78091578003889595, -27.53959229564985023, 33.79492750791695954 ) ) ;
#14255=CARTESIAN_POINT ( 'NONE',  ( -19.99999999999999645, -24.16482700510261949, 31.17382249208304046 ) ) ;
#14268=CARTESIAN_POINT ( 'NONE',  ( -13.49542703274178379, -19.04416526290806289, 4.482427507916957765 ) ) ;
#14271=CARTESIAN_POINT ( 'NONE',  ( -7.955834737091903364, -25.71081734191518464, 39.26757249208304756 ) ) ;
#14287=CARTESIAN_POINT ( 'NONE',  ( -22.04416526290807710, -25.71081734191525925, 39.48242750791695244 ) ) ;
#14292=CARTESIAN_POINT ( 'NONE',  ( -12.31951028609536536, -25.35725562635139596, 28.98632249208304401 ) ) ;
#14293=CARTESIAN_POINT ( 'NONE',  ( -20.00369391078762860, -18.75498260482333279, 24.60742750791696309 ) ) ;
#14308=ADVANCED_FACE ( 'NONE', ( #12555 ), #10884, .T. ) ;
#14315=CARTESIAN_POINT ( 'NONE',  ( -10.75228648362910100, -26.64274437364854009, 32.26367750791695954 ) ) ;
#14318=CARTESIAN_POINT ( 'NONE',  ( -16.50457296725825174, -19.04416526290807354, 32.26757249208304046 ) ) ;
#14323=CARTESIAN_POINT ( 'NONE',  ( -15.16482700510262482, -20.99999999999997513, 32.48632249208304756 ) ) ;
#14336=CARTESIAN_POINT ( 'NONE',  ( -19.95583473709191580, -22.49542703274176603, 29.41992750791695599 ) ) ;
#14339=CARTESIAN_POINT ( 'NONE',  ( -15.16482700510263371, -18.99999999999997868, 27.23632249208304046 ) ) ;
#14343=CARTESIAN_POINT ( 'NONE',  ( -14.83517299489739649, -18.99999999999997868, 25.26367750791695599 ) ) ;
#14345=CARTESIAN_POINT ( 'NONE',  ( -19.41254052147348830, -26.35725562635142083, 28.76367750791695954 ) ) ;
#14347=CARTESIAN_POINT ( 'NONE',  ( -10.58745947852648328, -26.35725562635138530, 39.48632249208304046 ) ) ;
#14358=CARTESIAN_POINT ( 'NONE',  ( -16.35725562635142794, -21.31951028609535470, 40.57617750791696665 ) ) ;
#14360=CARTESIAN_POINT ( 'NONE',  ( -7.955834737091903364, -25.71081734191518464, 34.01757249208303335 ) ) ;
#14375=CARTESIAN_POINT ( 'NONE',  ( -9.754982604823302594, -29.00369391078756465, 8.205072492083040459 ) ) ;
#14382=CARTESIAN_POINT ( 'NONE',  ( -11.99999999999999289, -23.83517299489735564, 39.04882249208304756 ) ) ;
#14383=CARTESIAN_POINT ( 'NONE',  ( -8.855408670957631401, -20.64274437364852943, 31.38867750791695599 ) ) ;
#14406=CARTESIAN_POINT ( 'NONE',  ( -11.64274437364854187, -30.14459132904234195, 1.201177507916956433 ) ) ;
#14411=CARTESIAN_POINT ( 'NONE',  ( -12.48433729119799196, -22.35725562635139596, 1.861322492083043123 ) ) ;
#14416=CARTESIAN_POINT ( 'NONE',  ( -15.63902057219073605, -27.04416526290807710, 35.33007249208304046 ) ) ;
#14428=CARTESIAN_POINT ( 'NONE',  ( -17.35725562635144215, -19.58745947852648683, 24.82617750791695954 ) ) ;
#14431=CARTESIAN_POINT ( 'NONE',  ( -19.41254052147348830, -26.35725562635142083, 7.763677507916958653 ) ) ;
#14435=CARTESIAN_POINT ( 'NONE',  ( -20.00369391078757886, -29.24501739517668142, 30.51757249208304401 ) ) ;
#14437=CARTESIAN_POINT ( 'NONE',  ( -11.46040770435012668, -27.78091578003887463, 37.73242750791694533 ) ) ;
#14439=CARTESIAN_POINT ( 'NONE',  ( -17.35725562635140307, -28.41254052147349185, 35.54882249208304046 ) ) ;
#14443=CARTESIAN_POINT ( 'NONE',  ( -14.83517299489739649, -18.99999999999997868, 35.76367750791695954 ) ) ;
#14445=CARTESIAN_POINT ( 'NONE',  ( -16.17491895705301275, -18.95583473709189448, 35.54492750791695954 ) ) ;
#14447=CARTESIAN_POINT ( 'NONE',  ( -20.04416526290809131, -22.82508104294700502, 41.89257249208303335 ) ) ;
#14460=CARTESIAN_POINT ( 'NONE',  ( -11.46040770435012668, -27.78091578003887463, 6.232427507916956877 ) ) ;
#14463=CARTESIAN_POINT ( 'NONE',  ( -7.999999999999996447, -23.83517299489733432, 33.79882249208304046 ) ) ;
#14476=CARTESIAN_POINT ( 'NONE',  ( -11.64274437364859693, -17.85540867095757989, 1.423822492083038904 ) ) ;
#14481=CARTESIAN_POINT ( 'NONE',  ( -17.95583473709191580, -23.03132541760400898, 8.419927507916959541 ) ) ;
#14482=CARTESIAN_POINT ( 'NONE',  ( -8.855408670957631401, -20.64274437364852943, 36.63867750791695244 ) ) ;
#14502=CARTESIAN_POINT ( 'NONE',  ( -11.46040770435012668, -27.78091578003887463, 37.73242750791694533 ) ) ;
#14506=CARTESIAN_POINT ( 'NONE',  ( -17.51566270880199738, -25.64274437364856496, 9.736322492083042235 ) ) ;
#14510=CARTESIAN_POINT ( 'NONE',  ( -16.35725562635142794, -21.31951028609535470, 9.076177507916959541 ) ) ;
#14520=CARTESIAN_POINT ( 'NONE',  ( -15.16482700510259640, -28.99999999999998224, 22.63867750791695954 ) ) ;
#14524=CARTESIAN_POINT ( 'NONE',  ( -13.82508104294698192, -29.04416526290806644, 6.669927507916955989 ) ) ;
#14528=CARTESIAN_POINT ( 'NONE',  ( -13.49542703274174116, -28.95583473709188738, 8.642572492083040459 ) ) ;
#14529=CARTESIAN_POINT ( 'NONE',  ( -16.17491895705301275, -18.95583473709189803, 40.79492750791695954 ) ) ;
#14531=CARTESIAN_POINT ( 'NONE',  ( -11.21908421996106320, -27.53959229564982181, 29.20507249208303335 ) ) ;
#14537=CARTESIAN_POINT ( 'NONE',  ( -18.53959229564986799, -20.21908421996107563, 29.85742750791695599 ) ) ;
#14541=CARTESIAN_POINT ( 'NONE',  ( -19.24771351637086880, -26.64274437364857206, 41.23632249208304046 ) ) ;
#14553=CARTESIAN_POINT ( 'NONE',  ( -14.83517299489739649, -18.99999999999997868, 4.263677507916958653 ) ) ;
#14554=CARTESIAN_POINT ( 'NONE',  ( -11.46040770435012668, -27.78091578003887463, 0.9824275079169582092 ) ) ;
#14556=CARTESIAN_POINT ( 'NONE',  ( -15.16482700510264436, -16.99999999999997868, 37.73632249208302625 ) ) ;
#14559=CARTESIAN_POINT ( 'NONE',  ( -17.51566270880201159, -22.35725562635141728, 29.63867750791695954 ) ) ;
#14561=CARTESIAN_POINT ( 'NONE',  ( -17.35725562635144215, -19.58745947852648683, 9.076177507916957765 ) ) ;
#14573=CARTESIAN_POINT ( 'NONE',  ( -21.95583473709189803, -26.04047135212049469, 9.955072492083038682 ) ) ;
#14580=CARTESIAN_POINT ( 'NONE',  ( -11.95583473709190514, -24.63902057219072361, 39.26757249208304756 ) ) ;
#14581=CARTESIAN_POINT ( 'NONE',  ( -16.71081734191527346, -16.95583473709190159, 35.54492750791695954 ) ) ;
#14604=CARTESIAN_POINT ( 'NONE',  ( -18.78091578003889950, -27.53959229564985378, 39.04492750791695954 ) ) ;
#14607=CARTESIAN_POINT ( 'NONE',  ( -17.95583473709190869, -24.96867458239598037, 4.705072492083043123 ) ) ;
#14612=CARTESIAN_POINT ( 'NONE',  ( -16.64274437364858272, -21.48433729119797420, 42.54882249208304756 ) ) ;
#14622=CARTESIAN_POINT ( 'NONE',  ( -17.64274437364855430, -28.24771351637087236, 28.32617750791695954 ) ) ;
#14624=CARTESIAN_POINT ( 'NONE',  ( -20.04416526290808065, -25.17491895705300209, 2.732427507916957765 ) ) ;
#14628=CARTESIAN_POINT ( 'NONE',  ( -11.21908421996106320, -27.53959229564982181, 2.955072492083040903 ) ) ;
#14629=CARTESIAN_POINT ( 'NONE',  ( -21.14459132904236327, -27.35725562635143149, 2.513677507916956433 ) ) ;
#14631=CARTESIAN_POINT ( 'NONE',  ( -17.64274437364858983, -19.75228648362910633, 42.54882249208304046 ) ) ;
#14638=CARTESIAN_POINT ( 'NONE',  ( -17.35725562635144215, -19.58745947852648683, 40.57617750791696665 ) ) ;
#14640=CARTESIAN_POINT ( 'NONE',  ( -15.16482700510263371, -18.99999999999997868, 37.73632249208303335 ) ) ;
#14650=CARTESIAN_POINT ( 'NONE',  ( -12.04416526290807887, -24.96867458239596260, 37.29492750791695954 ) ) ;
#14653=CARTESIAN_POINT ( 'NONE',  ( -18.78091578003892081, -20.46040770435013556, 10.83007249208303691 ) ) ;
#14655=CARTESIAN_POINT ( 'NONE',  ( -12.31951028609537602, -22.64274437364854364, 36.63867750791695244 ) ) ;
#14656=CARTESIAN_POINT ( 'NONE',  ( -16.50457296725820555, -28.95583473709189803, 1.857427507916957987 ) ) ;
#14668=CARTESIAN_POINT ( 'NONE',  ( -11.35725562635139418, -29.97976432393972601, 8.423822492083040459 ) ) ;
#14671=CARTESIAN_POINT ( 'NONE',  ( -9.955834737091903364, -25.17491895705295235, 2.517572492083040903 ) ) ;
#14674=CARTESIAN_POINT ( 'NONE',  ( -12.68318583509882380, -26.07549068051207541, 39.70507249208305467 ) ) ;
#14675=CARTESIAN_POINT ( 'NONE',  ( -9.996306089212364299, -29.24501739517662813, 27.23242750791696309 ) ) ;
#14698=CARTESIAN_POINT ( 'NONE',  ( -13.82508104294698192, -29.04416526290806644, 38.16992750791695244 ) ) ;
#14702=CARTESIAN_POINT ( 'NONE',  ( -19.41254052147350961, -21.64274437364857562, 42.11132249208304046 ) ) ;
#14707=CARTESIAN_POINT ( 'NONE',  ( -11.99999999999999289, -24.16482700510258752, 5.576177507916960430 ) ) ;
#14719=CARTESIAN_POINT ( 'NONE',  ( -12.35725562635143682, -19.75228648362908501, 20.45117750791695954 ) ) ;
#14723=CARTESIAN_POINT ( 'NONE',  ( -20.04416526290808065, -25.17491895705300209, 7.982427507916958653 ) ) ;
#14727=CARTESIAN_POINT ( 'NONE',  ( -11.46040770435014977, -20.21908421996103655, 1.642572492083041125 ) ) ;
#14728=CARTESIAN_POINT ( 'NONE',  ( -8.855408670957631401, -20.64274437364852943, 10.38867750791695599 ) ) ;
#14731=CARTESIAN_POINT ( 'NONE',  ( -11.95583473709190514, -24.63902057219072361, 2.517572492083043123 ) ) ;
#14736=CARTESIAN_POINT ( 'NONE',  ( -15.16482700510259640, -28.99999999999998224, 38.38867750791695954 ) ) ;
#14741=CARTESIAN_POINT ( 'NONE',  ( -19.95583473709190514, -25.50457296725823042, 36.20507249208304046 ) ) ;
#14754=CARTESIAN_POINT ( 'NONE',  ( -10.58745947852649927, -21.64274437364853654, -0.1113224920830418047 ) ) ;
#14755=CARTESIAN_POINT ( 'NONE',  ( -9.955834737091912245, -22.82508104294696594, 15.85742750791695777 ) ) ;
#14758=CARTESIAN_POINT ( 'NONE',  ( -15.16482700510264436, -16.99999999999997868, 42.98632249208304756 ) ) ;
#14761=CARTESIAN_POINT ( 'NONE',  ( -10.75228648362910100, -26.64274437364854009, 6.013677507916958653 ) ) ;
#14762=CARTESIAN_POINT ( 'NONE',  ( -20.04416526290808065, -25.17491895705300209, 2.732427507916958209 ) ) ;
#14777=CARTESIAN_POINT ( 'NONE',  ( -11.35725562635139418, -29.97976432393972601, 18.92382249208303691 ) ) ;
#14782=CARTESIAN_POINT ( 'NONE',  ( -12.48433729119798130, -25.64274437364855075, 0.7636775079169598746 ) ) ;
#14784=CARTESIAN_POINT ( 'NONE',  ( -20.97976432393977575, -20.35725562635143504, 40.13867750791695954 ) ) ;
#14794=CARTESIAN_POINT ( 'NONE',  ( -11.05206702929440254, -21.80946413714601562, 1.107186296610940179E-15 ) ) ;
#14805=CARTESIAN_POINT ( 'NONE',  ( -18.64274437364853654, -29.97976432393976509, 2.076177507916956433 ) ) ;
#14809=CARTESIAN_POINT ( 'NONE',  ( -12.92450931948790149, -21.68318583509881137, 1.642572492083043123 ) ) ;
#14813=CARTESIAN_POINT ( 'NONE',  ( -12.04416526290807887, -24.96867458239596260, 5.794927507916960430 ) ) ;
#14814=CARTESIAN_POINT ( 'NONE',  ( -15.00000000000001421, -18.99999999999997868, -4.336808689942017736E-16 ) ) ;
#14826=CARTESIAN_POINT ( 'NONE',  ( -9.955834737091912245, -22.82508104294696594, 5.357427507916956877 ) ) ;
#14829=CARTESIAN_POINT ( 'NONE',  ( -17.04047135212050890, -17.04416526290807710, 42.76757249208304046 ) ) ;
#14830=CARTESIAN_POINT ( 'NONE',  ( -21.95583473709191580, -21.95952864787954084, 3.169927507916957321 ) ) ;
#14832=CARTESIAN_POINT ( 'NONE',  ( -14.83517299489736985, -26.99999999999998579, 8.861322492083040459 ) ) ;
#14835=CARTESIAN_POINT ( 'NONE',  ( -13.51548992270003957, -18.19996206762383650, -8.139499971887964371E-17 ) ) ;
#14849=CARTESIAN_POINT ( 'NONE',  ( -19.41254052147348830, -26.35725562635142083, 2.513677507916958209 ) ) ;
#14851=CARTESIAN_POINT ( 'NONE',  ( -19.24771351637089367, -21.35725562635142438, 19.13867750791695954 ) ) ;
#14853=CARTESIAN_POINT ( 'NONE',  ( -10.58745947852648328, -26.35725562635138530, 2.736322492083041347 ) ) ;
#14855=CARTESIAN_POINT ( 'NONE',  ( -10.58745947852649927, -21.64274437364853654, 5.138677507916957765 ) ) ;
#14856=CARTESIAN_POINT ( 'NONE',  ( -10.58745947852649927, -21.64274437364853654, 5.138677507916957765 ) ) ;
#14870=CARTESIAN_POINT ( 'NONE',  ( -12.95952864787948755, -30.95583473709188382, 24.39257249208303691 ) ) ;
#14872=SURFACE_SIDE_STYLE ('',( #8884 ) ) ;
#14876=CARTESIAN_POINT ( 'NONE',  ( -14.36097942780923731, -27.04416526290806999, 17.16992750791696309 ) ) ;
#14878=CARTESIAN_POINT ( 'NONE',  ( -15.16482700510264436, -16.99999999999997868, 0.9863224920830391262 ) ) ;
#14899=CARTESIAN_POINT ( 'NONE',  ( -9.996306089212364299, -29.24501739517662813, 21.98242750791695599 ) ) ;
#14903=CARTESIAN_POINT ( 'NONE',  ( -11.99999999999999289, -23.83517299489735564, 23.29882249208304046 ) ) ;
#14910=CARTESIAN_POINT ( 'NONE',  ( -17.99999999999999645, -23.83517299489736985, 8.201177507916959541 ) ) ;
#14923=CARTESIAN_POINT ( 'NONE',  ( -18.78091578003889950, -27.53959229564985378, 39.04492750791695954 ) ) ;
#14925=CARTESIAN_POINT ( 'NONE',  ( -15.16482700510259640, -28.99999999999998224, 12.13867750791695777 ) ) ;
#14931=CARTESIAN_POINT ( 'NONE',  ( -9.955834737091903364, -25.17491895705294880, 7.767572492083041347 ) ) ;
#14934=CARTESIAN_POINT ( 'NONE',  ( -17.07549068051208963, -26.31681416490115311, 9.517572492083044011 ) ) ;
#14951=CARTESIAN_POINT ( 'NONE',  ( -9.999999999999994671, -24.16482700510257686, 5.576177507916958653 ) ) ;
#14952=CARTESIAN_POINT ( 'NONE',  ( -14.83517299489739649, -18.99999999999997868, 9.513677507916957765 ) ) ;
#14953=CARTESIAN_POINT ( 'NONE',  ( -17.04047135212050890, -17.04416526290807710, 42.76757249208304046 ) ) ;
#14955=CARTESIAN_POINT ( 'NONE',  ( -13.64274437364856141, -26.68048971390460622, 37.95117750791695244 ) ) ;
#14957=CARTESIAN_POINT ( 'NONE',  ( -9.955834737091912245, -22.82508104294696238, 5.357427507916956877 ) ) ;
#14969=CARTESIAN_POINT ( 'NONE',  ( -22.04416526290809486, -22.28918265808477628, 20.89257249208303691 ) ) ;
#14974=CARTESIAN_POINT ( 'NONE',  ( -12.92450931948788906, -26.31681416490114245, 11.48242750791695954 ) ) ;
#14976=CARTESIAN_POINT ( 'NONE',  ( -11.64274437364859693, -17.85540867095757989, 1.423822492083038904 ) ) ;
#14993=CARTESIAN_POINT ( 'NONE',  ( -9.020235676060220698, -27.64274437364852588, 11.26367750791695599 ) ) ;
#14998=CARTESIAN_POINT ( 'NONE',  ( -15.16482700510262482, -20.99999999999997513, 11.48632249208304223 ) ) ;
#15004=CARTESIAN_POINT ( 'NONE',  ( -14.83517299489738761, -20.99999999999997513, 20.01367750791696309 ) ) ;
#15017=CARTESIAN_POINT ( 'NONE',  ( -19.24771351637089367, -21.35725562635142438, 34.88867750791696665 ) ) ;
#15021=CARTESIAN_POINT ( 'NONE',  ( -16.50457296725820555, -28.95583473709189448, 17.60742750791695599 ) ) ;
#15026=CARTESIAN_POINT ( 'NONE',  ( -19.99999999999999645, -24.16482700510261949, 20.67382249208304401 ) ) ;
#15029=CARTESIAN_POINT ( 'NONE',  ( -17.31681416490117087, -21.92450931948788551, 10.83007249208304223 ) ) ;
#15049=CARTESIAN_POINT ( 'NONE',  ( -13.82508104294698192, -29.04416526290806644, 22.41992750791695244 ) ) ;
#15050=CARTESIAN_POINT ( 'NONE',  ( -17.64274437364855430, -28.24771351637087236, 12.57617750791695777 ) ) ;
#15052=CARTESIAN_POINT ( 'NONE',  ( -15.16482700510263371, -18.99999999999997868, 0.9863224920830410136 ) ) ;
#15055=CARTESIAN_POINT ( 'NONE',  ( -20.04416526290808065, -25.17491895705300209, 2.732427507916957765 ) ) ;
#15057=CARTESIAN_POINT ( 'NONE',  ( -19.24771351637089367, -21.35725562635142438, 24.38867750791695954 ) ) ;
#15073=CARTESIAN_POINT ( 'NONE',  ( -9.020235676060250896, -20.35725562635137820, 17.61132249208303335 ) ) ;
#15078=CARTESIAN_POINT ( 'NONE',  ( -17.51566270880201159, -22.35725562635141728, 13.88867750791695954 ) ) ;
#15080=CARTESIAN_POINT ( 'NONE',  ( -7.999999999999996447, -23.83517299489733432, 2.298822492083038682 ) ) ;
#15090=CARTESIAN_POINT ( 'NONE',  ( -10.71682923056184400, -22.10758631096295801, 1.196196559314993540E-16 ) ) ;
#15099=CARTESIAN_POINT ( 'NONE',  ( -18.64274437364853654, -29.97976432393976509, 12.57617750791695599 ) ) ;
#15104=CARTESIAN_POINT ( 'NONE',  ( -14.03132541760400009, -26.95583473709189448, 19.14257249208304401 ) ) ;
#15108=CARTESIAN_POINT ( 'NONE',  ( -17.07549068051210739, -21.68318583509881847, 14.10742750791695954 ) ) ;
#15122=CARTESIAN_POINT ( 'NONE',  ( -18.53959229564986799, -20.21908421996107563, 19.35742750791695599 ) ) ;
#15126=CARTESIAN_POINT ( 'NONE',  ( -14.83517299489735741, -28.99999999999998224, 19.36132249208304046 ) ) ;
#15129=CARTESIAN_POINT ( 'NONE',  ( -14.83517299489736985, -26.99999999999998579, 24.61132249208304756 ) ) ;
#15145=CARTESIAN_POINT ( 'NONE',  ( -19.95583473709191580, -22.49542703274176603, 24.16992750791694888 ) ) ;
#15147=CARTESIAN_POINT ( 'NONE',  ( -13.49542703274174116, -28.95583473709188738, 24.39257249208303335 ) ) ;
#15151=CARTESIAN_POINT ( 'NONE',  ( -17.95583473709191580, -23.03132541760400898, 39.91992750791695954 ) ) ;
#15154=CARTESIAN_POINT ( 'NONE',  ( -9.955834737091912245, -22.82508104294696238, 21.10742750791695599 ) ) ;
#15169=CARTESIAN_POINT ( 'NONE',  ( -9.754982604823302594, -29.00369391078756465, 13.45507249208303868 ) ) ;
#15171=CARTESIAN_POINT ( 'NONE',  ( -18.78091578003892792, -20.46040770435013556, 10.83007249208303868 ) ) ;
#15175=CARTESIAN_POINT ( 'NONE',  ( -15.63902057219076269, -20.95583473709189448, 14.54492750791695954 ) ) ;
#15177=CARTESIAN_POINT ( 'NONE',  ( -20.97976432393974022, -27.64274437364858628, 25.48632249208304401 ) ) ;
#15194=CARTESIAN_POINT ( 'NONE',  ( -15.16482700510258574, -30.99999999999998224, 17.38867750791695599 ) ) ;
#15201=CARTESIAN_POINT ( 'NONE',  ( -12.48433729119799196, -22.35725562635139596, 12.36132249208304401 ) ) ;
#15202=CARTESIAN_POINT ( 'NONE',  ( -18.35725562635144925, -17.85540867095761186, 3.826177507916956433 ) ) ;
#15206=CARTESIAN_POINT ( 'NONE',  ( -15.16482700510260706, -26.99999999999998579, 22.63867750791696309 ) ) ;
#15219=CARTESIAN_POINT ( 'NONE',  ( -19.95583473709191580, -22.49542703274176603, 34.66992750791694533 ) ) ;
#15222=CARTESIAN_POINT ( 'NONE',  ( -12.35725562635143682, -19.75228648362908501, 9.951177507916959541 ) ) ;
#15225=CARTESIAN_POINT ( 'NONE',  ( -19.24771351637086880, -26.64274437364857206, 20.23632249208304046 ) ) ;
#15228=CARTESIAN_POINT ( 'NONE',  ( -11.95583473709190514, -24.63902057219072361, 13.01757249208304401 ) ) ;
#15242=CARTESIAN_POINT ( 'NONE',  ( -17.35725562635144215, -19.58745947852648683, 14.32617750791695777 ) ) ;
#15245=CARTESIAN_POINT ( 'NONE',  ( -18.53959229564982536, -27.78091578003890660, 20.01757249208304046 ) ) ;
#15249=CARTESIAN_POINT ( 'NONE',  ( -9.955834737091912245, -22.82508104294696594, 10.60742750791695777 ) ) ;
#15251=CARTESIAN_POINT ( 'NONE',  ( -19.24771351637089367, -21.35725562635142438, 19.13867750791695954 ) ) ;
#15265=CARTESIAN_POINT ( 'NONE',  ( -9.996306089212408708, -18.75498260482328661, 38.39257249208304756 ) ) ;
#15266=CARTESIAN_POINT ( 'NONE',  ( -15.16482700510263371, -18.99999999999997868, 16.73632249208304401 ) ) ;
#15268=CARTESIAN_POINT ( 'NONE',  ( -13.35725562635142794, -21.48433729119796709, 9.951177507916961318 ) ) ;
#15270=CARTESIAN_POINT ( 'NONE',  ( -21.14459132904239169, -20.64274437364858628, 21.11132249208304046 ) ) ;
#15273=EDGE_LOOP ( 'NONE', ( #5, #8233, #19385, #1147, #953 ) ) ;
#15287=CARTESIAN_POINT ( 'NONE',  ( -22.04416526290807710, -25.71081734191525925, 13.23242750791695777 ) ) ;
#15292=CARTESIAN_POINT ( 'NONE',  ( -16.35725562635141372, -26.68048971390461332, 14.54882249208304401 ) ) ;
#15293=CARTESIAN_POINT ( 'NONE',  ( -18.35725562635144925, -17.85540867095761186, 14.32617750791695599 ) ) ;
#15298=CARTESIAN_POINT ( 'NONE',  ( -12.31951028609537602, -22.64274437364854364, 15.63867750791696309 ) ) ;
#15313=CARTESIAN_POINT ( 'NONE',  ( -10.58745947852649927, -21.64274437364853654, 20.88867750791695954 ) ) ;
#15316=CARTESIAN_POINT ( 'NONE',  ( -15.16482700510263371, -18.99999999999997868, 21.98632249208304401 ) ) ;
#15319=CARTESIAN_POINT ( 'NONE',  ( -15.63902057219073605, -27.04416526290807710, 14.33007249208304223 ) ) ;
#15337=CARTESIAN_POINT ( 'NONE',  ( -12.64274437364855252, -28.41254052147347053, 16.95117750791695954 ) ) ;
#15340=CARTESIAN_POINT ( 'NONE',  ( -18.53959229564982536, -27.78091578003890660, 25.26757249208304401 ) ) ;
#15343=CARTESIAN_POINT ( 'NONE',  ( -20.04416526290808065, -25.17491895705300209, 13.23242750791695777 ) ) ;
#15345=CARTESIAN_POINT ( 'NONE',  ( -17.64274437364855430, -28.24771351637087236, 12.57617750791695777 ) ) ;
#15361=CARTESIAN_POINT ( 'NONE',  ( -7.999999999999996447, -23.83517299489733432, 39.04882249208302625 ) ) ;
#15365=CARTESIAN_POINT ( 'NONE',  ( -10.75228648362912232, -21.35725562635138530, 12.36132249208304046 ) ) ;
#15367=CARTESIAN_POINT ( 'NONE',  ( -12.04416526290807887, -24.96867458239596260, 32.04492750791695954 ) ) ;
#15369=CARTESIAN_POINT ( 'NONE',  ( -20.00369391078757886, -29.24501739517668142, 14.76757249208304046 ) ) ;
#15391=CARTESIAN_POINT ( 'NONE',  ( -21.14459132904236327, -27.35725562635143149, 28.76367750791696309 ) ) ;
#15395=CARTESIAN_POINT ( 'NONE',  ( -17.51566270880199738, -25.64274437364856496, 35.98632249208304756 ) ) ;
#15396=CARTESIAN_POINT ( 'NONE',  ( -11.64274437364854187, -30.14459132904234195, 11.70117750791695777 ) ) ;
#15400=CARTESIAN_POINT ( 'NONE',  ( -13.35725562635142794, -21.48433729119796709, 9.951177507916961318 ) ) ;
#15422=CARTESIAN_POINT ( 'NONE',  ( -10.58745947852649927, -21.64274437364853654, 26.13867750791695599 ) ) ;
#15425=CARTESIAN_POINT ( 'NONE',  ( -9.955834737091903364, -25.17491895705294880, 18.26757249208304401 ) ) ;
#15427=CARTESIAN_POINT ( 'NONE',  ( -17.68048971390462754, -22.64274437364856496, 15.86132249208304401 ) ) ;
#15440=CARTESIAN_POINT ( 'NONE',  ( -10.04416526290807710, -25.50457296725819489, 21.54492750791695599 ) ) ;
#15442=CARTESIAN_POINT ( 'NONE',  ( -10.04416526290808953, -22.49542703274172695, 23.08007249208303335 ) ) ;
#15444=CARTESIAN_POINT ( 'NONE',  ( -18.78091578003889950, -27.53959229564985378, 12.79492750791695421 ) ) ;
#15446=CARTESIAN_POINT ( 'NONE',  ( -19.99999999999999645, -23.83517299489738051, 23.95117750791695954 ) ) ;
#15448=CARTESIAN_POINT ( 'NONE',  ( -16.17491895705296656, -29.04416526290807354, 30.08007249208304401 ) ) ;
#15457=CARTESIAN_POINT ( 'NONE',  ( -20.00369391078757886, -29.24501739517668142, 25.26757249208304401 ) ) ;
#15458=CARTESIAN_POINT ( 'NONE',  ( -17.35725562635140307, -28.41254052147349185, 9.298822492083040459 ) ) ;
#15460=CARTESIAN_POINT ( 'NONE',  ( -17.07549068051210739, -21.68318583509881847, 24.60742750791696309 ) ) ;
#15463=CARTESIAN_POINT ( 'NONE',  ( -17.04047135212050890, -17.04416526290807710, 16.51757249208304046 ) ) ;
#15481=CARTESIAN_POINT ( 'NONE',  ( -13.28918265808472299, -31.04416526290805933, 27.66992750791695954 ) ) ;
#15485=CARTESIAN_POINT ( 'NONE',  ( -17.31681416490117087, -21.92450931948788551, 37.08007249208304756 ) ) ;
#15486=CARTESIAN_POINT ( 'NONE',  ( -9.020235676060220698, -27.64274437364852588, 11.26367750791695599 ) ) ;
#15492=CARTESIAN_POINT ( 'NONE',  ( -17.07549068051210739, -21.68318583509881847, 29.85742750791696309 ) ) ;
#15509=CARTESIAN_POINT ( 'NONE',  ( -19.99999999999999645, -23.83517299489738051, 29.20117750791695599 ) ) ;
#15514=CARTESIAN_POINT ( 'NONE',  ( -16.17491895705296656, -29.04416526290807710, 35.33007249208301914 ) ) ;
#15516=CARTESIAN_POINT ( 'NONE',  ( -11.99999999999999289, -23.83517299489735564, 39.04882249208304756 ) ) ;
#15536=CARTESIAN_POINT ( 'NONE',  ( -19.24771351637089367, -21.35725562635142438, 29.63867750791695599 ) ) ;
#15538=CARTESIAN_POINT ( 'NONE',  ( -16.50457296725825174, -19.04416526290807354, 16.51757249208304046 ) ) ;
#15540=CARTESIAN_POINT ( 'NONE',  ( -12.64274437364855252, -28.41254052147347053, 22.20117750791695599 ) ) ;
#15543=CARTESIAN_POINT ( 'NONE',  ( -9.955834737091912245, -22.82508104294696238, 31.60742750791695954 ) ) ;
#15545=CARTESIAN_POINT ( 'NONE',  ( -16.17491895705296656, -29.04416526290807354, 24.83007249208304401 ) ) ;
#15555=CARTESIAN_POINT ( 'NONE',  ( -11.64274437364859693, -17.85540867095757989, 27.67382249208304401 ) ) ;
#15558=CARTESIAN_POINT ( 'NONE',  ( -9.999999999999994671, -23.83517299489734143, 7.548822492083041347 ) ) ;
#15559=CARTESIAN_POINT ( 'NONE',  ( -17.95583473709191580, -23.03132541760400898, 34.66992750791696665 ) ) ;
#15561=CARTESIAN_POINT ( 'NONE',  ( -9.020235676060250896, -20.35725562635137820, 22.86132249208304046 ) ) ;
#15577=CARTESIAN_POINT ( 'NONE',  ( -12.95952864787955150, -17.04416526290805933, 25.48242750791696309 ) ) ;
#15581=CARTESIAN_POINT ( 'NONE',  ( -12.04416526290808420, -23.03132541760398766, 33.58007249208304756 ) ) ;
#15582=CARTESIAN_POINT ( 'NONE',  ( -9.996306089212364299, -29.24501739517662813, 16.73242750791695954 ) ) ;
#15587=CARTESIAN_POINT ( 'NONE',  ( -17.99999999999999645, -23.83517299489736985, 23.95117750791696309 ) ) ;
#15602=CARTESIAN_POINT ( 'NONE',  ( -11.46040770435012668, -27.78091578003887463, 27.23242750791694888 ) ) ;
#15606=CARTESIAN_POINT ( 'NONE',  ( -13.49542703274174116, -28.95583473709188738, 29.64257249208303691 ) ) ;
#15607=CARTESIAN_POINT ( 'NONE',  ( -17.99999999999999645, -24.16482700510260173, 36.42382249208304756 ) ) ;
#15625=CARTESIAN_POINT ( 'NONE',  ( -19.99999999999999645, -23.83517299489738051, 29.20117750791695599 ) ) ;
#15627=CARTESIAN_POINT ( 'NONE',  ( -9.955834737091903364, -25.17491895705294880, 34.01757249208303335 ) ) ;
#15630=CARTESIAN_POINT ( 'NONE',  ( -15.16482700510259640, -28.99999999999998224, 17.38867750791695599 ) ) ;
#15633=CARTESIAN_POINT ( 'NONE',  ( -11.46040770435012490, -27.78091578003888173, 37.73242750791695954 ) ) ;
#15635=CARTESIAN_POINT ( 'NONE',  ( -9.955834737091903364, -25.17491895705295235, 23.51757249208304046 ) ) ;
#15647=CARTESIAN_POINT ( 'NONE',  ( -11.64274437364859693, -17.85540867095757989, 38.17382249208303335 ) ) ;
#15651=CARTESIAN_POINT ( 'NONE',  ( -14.03132541760401786, -21.04416526290806289, 30.73242750791696309 ) ) ;
#15653=CARTESIAN_POINT ( 'NONE',  ( -8.044165262908093084, -21.95952864787946979, 28.33007249208304756 ) ) ;
#15672=CARTESIAN_POINT ( 'NONE',  ( -18.35725562635144925, -17.85540867095761186, 30.07617750791695599 ) ) ;
#15677=CARTESIAN_POINT ( 'NONE',  ( -12.04416526290808420, -23.03132541760398766, 28.33007249208304756 ) ) ;
#15678=CARTESIAN_POINT ( 'NONE',  ( -12.95952864787955150, -17.04416526290805933, 14.98242750791695777 ) ) ;
#15684=CARTESIAN_POINT ( 'NONE',  ( -17.99999999999999645, -23.83517299489736985, 29.20117750791695954 ) ) ;
#15702=CARTESIAN_POINT ( 'NONE',  ( -18.53959229564986799, -20.21908421996107563, 35.10742750791694533 ) ) ;
#15706=CARTESIAN_POINT ( 'NONE',  ( -10.04416526290808953, -22.49542703274172695, 33.58007249208304046 ) ) ;
#15709=CARTESIAN_POINT ( 'NONE',  ( -16.64274437364858272, -21.48433729119797420, 26.79882249208304401 ) ) ;
#15730=CARTESIAN_POINT ( 'NONE',  ( -10.58745947852649927, -21.64274437364853654, 26.13867750791695599 ) ) ;
#15733=CARTESIAN_POINT ( 'NONE',  ( -20.04416526290809131, -22.82508104294699791, 31.39257249208304046 ) ) ;
#15735=CARTESIAN_POINT ( 'NONE',  ( -12.35725562635143682, -19.75228648362908501, 36.20117750791695954 ) ) ;
#15737=CARTESIAN_POINT ( 'NONE',  ( -17.64274437364855430, -28.24771351637087236, 38.82617750791695954 ) ) ;
#15739=CARTESIAN_POINT ( 'NONE',  ( -18.78091578003892792, -20.46040770435013556, 21.33007249208304046 ) ) ;
#15750=CARTESIAN_POINT ( 'NONE',  ( -17.68048971390461688, -25.35725562635141372, 28.76367750791696309 ) ) ;
#15753=CARTESIAN_POINT ( 'NONE',  ( -8.855408670957602979, -27.35725562635137820, 39.48632249208304046 ) ) ;
#15768=CARTESIAN_POINT ( 'NONE',  ( -20.24501739517664234, -29.00369391078761439, 39.04492750791695954 ) ) ;
#15772=CARTESIAN_POINT ( 'NONE',  ( -15.16482700510262482, -20.99999999999997513, 27.23632249208304046 ) ) ;
#15773=CARTESIAN_POINT ( 'NONE',  ( -21.99999999999999289, -23.83517299489739116, 29.20117750791695244 ) ) ;
#15794=CARTESIAN_POINT ( 'NONE',  ( -10.04416526290807710, -25.50457296725819489, 26.79492750791695954 ) ) ;
#15798=CARTESIAN_POINT ( 'NONE',  ( -13.82508104294702100, -18.95583473709188382, 37.95507249208304756 ) ) ;
#15800=CARTESIAN_POINT ( 'NONE',  ( -17.68048971390462754, -22.64274437364856496, 31.61132249208304401 ) ) ;
#15816=CARTESIAN_POINT ( 'NONE',  ( -12.35725562635143682, -19.75228648362908501, 36.20117750791695954 ) ) ;
#15819=CARTESIAN_POINT ( 'NONE',  ( -12.35725562635140307, -28.24771351637085459, 29.42382249208304401 ) ) ;
#15821=CARTESIAN_POINT ( 'NONE',  ( -19.24771351637089367, -21.35725562635142438, 34.88867750791696665 ) ) ;
#15823=CARTESIAN_POINT ( 'NONE',  ( -13.49542703274178201, -19.04416526290806289, 35.98242750791695954 ) ) ;
#15825=CARTESIAN_POINT ( 'NONE',  ( -20.04416526290809131, -22.82508104294700502, 26.14257249208304046 ) ) ;
#15839=CARTESIAN_POINT ( 'NONE',  ( -15.16482700510260706, -26.99999999999998579, 38.38867750791695954 ) ) ;
#15841=CARTESIAN_POINT ( 'NONE',  ( -21.14459132904239169, -20.64274437364858628, 31.61132249208303691 ) ) ;
#15856=AXIS2_PLACEMENT_3D ( 'NONE', #11170, #8156, #17263 ) ;
#15860=CARTESIAN_POINT ( 'NONE',  ( -15.16482700510258574, -30.99999999999998224, 38.38867750791694533 ) ) ;
#15864=CARTESIAN_POINT ( 'NONE',  ( -17.68048971390462754, -22.64274437364856496, 42.11132249208304756 ) ) ;
#15865=CARTESIAN_POINT ( 'NONE',  ( -11.64274437364854187, -30.14459132904234195, 27.45117750791696309 ) ) ;
#15885=CARTESIAN_POINT ( 'NONE',  ( -21.99999999999999289, -23.83517299489739116, 8.201177507916955989 ) ) ;
#15887=VERTEX_POINT ( 'NONE', #19141 ) ;
#15888=CARTESIAN_POINT ( 'NONE',  ( -18.53959229564982536, -27.78091578003890660, 30.51757249208304401 ) ) ;
#15891=CARTESIAN_POINT ( 'NONE',  ( -14.83517299489736985, -26.99999999999998579, 29.86132249208304756 ) ) ;
#15900=CARTESIAN_POINT ( 'NONE',  ( -12.35725562635143682, -19.75228648362908501, 30.95117750791695954 ) ) ;
#15904=CARTESIAN_POINT ( 'NONE',  ( -14.83517299489739649, -18.99999999999997868, 9.513677507916957765 ) ) ;
#15909=CARTESIAN_POINT ( 'NONE',  ( -13.49542703274178379, -19.04416526290806289, 30.73242750791695599 ) ) ;
#15911=CARTESIAN_POINT ( 'NONE',  ( -19.99999999999999645, -24.16482700510261949, 36.42382249208304046 ) ) ;
#15916=CARTESIAN_POINT ( 'NONE',  ( -10.75228648362910100, -26.64274437364854009, 27.01367750791695954 ) ) ;
#15918=CARTESIAN_POINT ( 'NONE',  ( -13.82508104294698015, -29.04416526290806289, 27.66992750791695599 ) ) ;
#15930=CARTESIAN_POINT ( 'NONE',  ( -19.41254052147348830, -26.35725562635142083, 2.513677507916958209 ) ) ;
#15932=CARTESIAN_POINT ( 'NONE',  ( -21.95583473709189803, -26.04047135212049469, 30.95507249208304401 ) ) ;
#15941=ADVANCED_FACE ( 'NONE', ( #11672 ), #518, .T. ) ;
#15950=CARTESIAN_POINT ( 'NONE',  ( -15.16482700510264436, -16.99999999999997868, 6.236322492083039570 ) ) ;
#15957=CARTESIAN_POINT ( 'NONE',  ( -17.68048971390461688, -25.35725562635141372, 7.763677507916960430 ) ) ;
#15958=CARTESIAN_POINT ( 'NONE',  ( -16.71081734191527346, -16.95583473709190159, 30.29492750791696665 ) ) ;
#15983=CARTESIAN_POINT ( 'NONE',  ( -11.35725562635144925, -18.02023567606020293, 4.701177507916955989 ) ) ;
#15987=CARTESIAN_POINT ( 'NONE',  ( -12.92450931948790149, -21.68318583509881137, 6.892572492083043123 ) ) ;
#15993=CARTESIAN_POINT ( 'NONE',  ( -17.31681416490115311, -26.07549068051209318, 2.294927507916959986 ) ) ;
#16005=CARTESIAN_POINT ( 'NONE',  ( -14.83517299489739649, -18.99999999999997868, 25.26367750791695599 ) ) ;
#16007=CARTESIAN_POINT ( 'NONE',  ( -10.04416526290807710, -25.50457296725819489, 5.794927507916955989 ) ) ;
#16012=CARTESIAN_POINT ( 'NONE',  ( -19.99999999999999645, -24.16482700510261949, 4.923822492083040459 ) ) ;
#16014=CARTESIAN_POINT ( 'NONE',  ( -7.999999999999996447, -24.16482700510256976, 0.3261775079169564884 ) ) ;
#16016=CARTESIAN_POINT ( 'NONE',  ( -12.35725562635140307, -28.24771351637085459, 34.67382249208304046 ) ) ;
#16020=CARTESIAN_POINT ( 'NONE',  ( -19.24771351637089367, -21.35725562635142438, 24.38867750791695954 ) ) ;
#16022=CARTESIAN_POINT ( 'NONE',  ( -14.83517299489739649, -18.99999999999997868, 41.01367750791696665 ) ) ;
#16024=CARTESIAN_POINT ( 'NONE',  ( -18.78091578003892792, -20.46040770435013556, 42.33007249208303335 ) ) ;
#16034=CARTESIAN_POINT ( 'NONE',  ( -11.99999999999999289, -24.16482700510258752, 37.07617750791695954 ) ) ;
#16036=CARTESIAN_POINT ( 'NONE',  ( -13.28918265808478694, -16.95583473709189093, 27.45507249208304046 ) ) ;
#16038=CARTESIAN_POINT ( 'NONE',  ( -14.03132541760401786, -21.04416526290806289, 25.48242750791696309 ) ) ;
#16039=CARTESIAN_POINT ( 'NONE',  ( -11.46040770435012490, -27.78091578003888173, 6.232427507916957765 ) ) ;
#16048=CARTESIAN_POINT ( 'NONE',  ( -18.64274437364860049, -18.02023567606023491, 5.798822492083038682 ) ) ;
#16052=CARTESIAN_POINT ( 'NONE',  ( -17.51566270880201159, -22.35725562635141728, 3.388677507916959986 ) ) ;
#16053=CARTESIAN_POINT ( 'NONE',  ( -11.35725562635144925, -18.02023567606020293, 36.20117750791695244 ) ) ;
#16073=CARTESIAN_POINT ( 'NONE',  ( -15.16482700510258574, -30.99999999999998224, 1.638677507916956433 ) ) ;
#16076=CARTESIAN_POINT ( 'NONE',  ( -12.35725562635140307, -28.24771351637085459, 39.92382249208304046 ) ) ;
#16077=EDGE_CURVE ( 'NONE', #18550, #13312, #1142, .T. ) ;
#16080=CARTESIAN_POINT ( 'NONE',  ( -14.36097942780923731, -27.04416526290806999, 6.669927507916960430 ) ) ;
#16090=CARTESIAN_POINT ( 'NONE',  ( -17.64274437364855430, -28.24771351637087236, 23.07617750791695954 ) ) ;
#16092=( GEOMETRIC_REPRESENTATION_CONTEXT ( 3 ) GLOBAL_UNCERTAINTY_ASSIGNED_CONTEXT ( ( #9637 ) ) GLOBAL_UNIT_ASSIGNED_CONTEXT ( ( #16512, #4264, #13364 ) ) REPRESENTATION_CONTEXT ( 'NONE', 'WORKASPACE' ) );
#16095=CARTESIAN_POINT ( 'NONE',  ( -10.04416526290807710, -25.50457296725819489, 0.5449275079169579872 ) ) ;
#16099=CARTESIAN_POINT ( 'NONE',  ( -18.78091578003892081, -20.46040770435013556, 10.83007249208303691 ) ) ;
#16100=CARTESIAN_POINT ( 'NONE',  ( -14.83517299489739649, -18.99999999999997868, 41.01367750791696665 ) ) ;
#16102=CARTESIAN_POINT ( 'NONE',  ( -15.63902057219073605, -27.04416526290807710, 3.830072492083042679 ) ) ;
#16112=CARTESIAN_POINT ( 'NONE',  ( -19.41254052147350961, -21.64274437364857562, 36.86132249208304046 ) ) ;
#16122=CARTESIAN_POINT ( 'NONE',  ( -19.99999999999999645, -23.83517299489738051, 2.951177507916958209 ) ) ;
#16123=CARTESIAN_POINT ( 'NONE',  ( -15.63902057219076269, -20.95583473709189448, 40.79492750791695244 ) ) ;
#16125=CARTESIAN_POINT ( 'NONE',  ( -18.64274437364860049, -18.02023567606023491, 42.54882249208304046 ) ) ;
#16127=CARTESIAN_POINT ( 'NONE',  ( -13.35725562635142794, -21.48433729119796709, 36.20117750791695954 ) ) ;
#16129=CARTESIAN_POINT ( 'NONE',  ( -11.46040770435012490, -27.78091578003888173, 0.9824275079169582092 ) ) ;
#16142=CARTESIAN_POINT ( 'NONE',  ( -11.35725562635139418, -29.97976432393972601, 3.173822492083039126 ) ) ;
#16149=CARTESIAN_POINT ( 'NONE',  ( -14.03132541760401786, -21.04416526290806289, -0.7675724920830402365 ) ) ;
#16150=CARTESIAN_POINT ( 'NONE',  ( -15.16482700510258574, -30.99999999999998224, 38.38867750791694533 ) ) ;
#16170=CARTESIAN_POINT ( 'NONE',  ( -15.16482700510258574, -30.99999999999998224, 6.888677507916956877 ) ) ;
#16174=CARTESIAN_POINT ( 'NONE',  ( -14.83517299489735741, -28.99999999999998224, 40.36132249208304046 ) ) ;
#16178=CARTESIAN_POINT ( 'NONE',  ( -17.95583473709190869, -24.96867458239598037, 41.45507249208304046 ) ) ;
#16189=COLOUR_RGB ( '', 0.31764706, 0.68627451, 0.89019608) ;
#16190=CARTESIAN_POINT ( 'NONE',  ( -11.21908421996108629, -20.46040770435011069, 31.16992750791695599 ) ) ;
#16192=CARTESIAN_POINT ( 'NONE',  ( -13.82508104294698192, -29.04416526290806644, 1.419927507916958209 ) ) ;
#16195=CARTESIAN_POINT ( 'NONE',  ( -11.35725562635139418, -29.97976432393972601, 39.92382249208304046 ) ) ;
#16196=CARTESIAN_POINT ( 'NONE',  ( -12.95952864787955150, -17.04416526290805933, 9.732427507916955989 ) ) ;
#16198=CARTESIAN_POINT ( 'NONE',  ( -12.92450931948790149, -21.68318583509881137, 1.642572492083043123 ) ) ;
#16208=CARTESIAN_POINT ( 'NONE',  ( -9.999999999999994671, -23.83517299489734143, 39.04882249208304046 ) ) ;
#16215=FACE_OUTER_BOUND ( 'NONE', #4541, .T. ) ;
#16216=CARTESIAN_POINT ( 'NONE',  ( -15.16482700510259640, -28.99999999999998224, 1.638677507916958431 ) ) ;
#16218=CARTESIAN_POINT ( 'NONE',  ( -18.53959229564982536, -27.78091578003890660, 9.517572492083042235 ) ) ;
#16222=CARTESIAN_POINT ( 'NONE',  ( -12.64274437364855252, -28.41254052147347053, 1.201177507916958431 ) ) ;
#16223=CARTESIAN_POINT ( 'NONE',  ( -18.53959229564986799, -20.21908421996107563, 3.607427507916957321 ) ) ;
#16235=CARTESIAN_POINT ( 'NONE',  ( -20.97976432393974022, -27.64274437364858628, 14.98632249208303868 ) ) ;
#16241=CARTESIAN_POINT ( 'NONE',  ( -15.16482700510260706, -26.99999999999998579, 1.638677507916960208 ) ) ;
#16242=CARTESIAN_POINT ( 'NONE',  ( -20.97976432393974022, -27.64274437364858628, 4.486322492083039570 ) ) ;
#16264=CARTESIAN_POINT ( 'NONE',  ( -19.95583473709191580, -22.49542703274176603, 39.91992750791695954 ) ) ;
#16269=CARTESIAN_POINT ( 'NONE',  ( -11.95583473709190514, -24.63902057219072361, 2.517572492083043123 ) ) ;
#16274=CARTESIAN_POINT ( 'NONE',  ( -16.35725562635142794, -21.31951028609535470, 3.826177507916959986 ) ) ;
#16275=VECTOR ( 'NONE', #17253, 1000.000000000000000 ) ;
#16285=CARTESIAN_POINT ( 'NONE',  ( -12.35725562635143682, -19.75228648362908501, 25.70117750791695599 ) ) ;
#16287=CARTESIAN_POINT ( 'NONE',  ( -12.35725562635143682, -19.75228648362908501, 4.701177507916957765 ) ) ;
#16292=CARTESIAN_POINT ( 'NONE',  ( -18.53959229564982536, -27.78091578003890660, 4.267572492083038682 ) ) ;
#16293=CARTESIAN_POINT ( 'NONE',  ( -16.71081734191527346, -16.95583473709190159, 4.044927507916956877 ) ) ;
#16294=CIRCLE ( 'NONE', #9731, 1.000000000000000000 ) ;
#16298=CARTESIAN_POINT ( 'NONE',  ( -13.35725562635141195, -26.51566270880198672, 3.173822492083044011 ) ) ;
#16302=CARTESIAN_POINT ( 'NONE',  ( -11.42876933740184775, -19.36634849019432991, 1.100789300500590883E-12 ) ) ;
#16310=CARTESIAN_POINT ( 'NONE',  ( -18.78091578003892792, -20.46040770435013556, 37.08007249208304046 ) ) ;
#16323=CARTESIAN_POINT ( 'NONE',  ( -17.64274437364855430, -28.24771351637087236, 7.326177507916957765 ) ) ;
#16324=CARTESIAN_POINT ( 'NONE',  ( -18.78091578003889950, -27.53959229564985378, 18.04492750791695954 ) ) ;
#16326=CARTESIAN_POINT ( 'NONE',  ( -20.97976432393974022, -27.64274437364858628, 41.23632249208304046 ) ) ;
#16329=CARTESIAN_POINT ( 'NONE',  ( -19.41254052147348830, -26.35725562635142083, 2.513677507916958209 ) ) ;
#16330=CARTESIAN_POINT ( 'NONE',  ( -10.75228648362910100, -26.64274437364854009, 11.26367750791695777 ) ) ;
#16345=CARTESIAN_POINT ( 'NONE',  ( -11.64274437364859693, -17.85540867095757989, 22.42382249208304046 ) ) ;
#16349=CARTESIAN_POINT ( 'NONE',  ( -12.31951028609537602, -22.64274437364854364, 20.88867750791696309 ) ) ;
#16351=CARTESIAN_POINT ( 'NONE',  ( -17.04047135212050890, -17.04416526290807710, 6.017572492083039570 ) ) ;
#16371=CARTESIAN_POINT ( 'NONE',  ( -8.855408670957631401, -20.64274437364852943, 10.38867750791695599 ) ) ;
#16375=CARTESIAN_POINT ( 'NONE',  ( -13.64274437364857739, -21.31951028609534760, 22.42382249208304401 ) ) ;
#16380=CARTESIAN_POINT ( 'NONE',  ( -14.36097942780923731, -27.04416526290806999, 1.419927507916959986 ) ) ;
#16393=CARTESIAN_POINT ( 'NONE',  ( -12.35725562635143682, -19.75228648362908501, 15.20117750791695777 ) ) ;
#16396=CARTESIAN_POINT ( 'NONE',  ( -9.999999999999994671, -23.83517299489734143, 7.548822492083041347 ) ) ;
#16398=CARTESIAN_POINT ( 'NONE',  ( -15.63902057219073605, -27.04416526290807710, 9.080072492083042235 ) ) ;
#16401=CARTESIAN_POINT ( 'NONE',  ( -10.24659852207731170, -22.21293927426971493, 2.322403871605816317E-12 ) ) ;
#16416=CARTESIAN_POINT ( 'NONE',  ( -14.83517299489739649, -18.99999999999997868, 9.513677507916957765 ) ) ;
#16417=CARTESIAN_POINT ( 'NONE',  ( -13.82508104294698192, -29.04416526290806644, 17.16992750791694888 ) ) ;
#16419=CARTESIAN_POINT ( 'NONE',  ( -9.999999999999994671, -23.83517299489734143, 2.298822492083040903 ) ) ;
#16421=CARTESIAN_POINT ( 'NONE',  ( -17.51566270880201159, -22.35725562635141728, 40.13867750791696665 ) ) ;
#16424=CARTESIAN_POINT ( 'NONE',  ( -19.41254052147348830, -26.35725562635142083, 2.513677507916958209 ) ) ;
#16437=CARTESIAN_POINT ( 'NONE',  ( -20.00369391078757886, -29.24501739517668142, 20.01757249208303691 ) ) ;
#16442=CARTESIAN_POINT ( 'NONE',  ( -13.64274437364856141, -26.68048971390460622, 11.70117750791696132 ) ) ;
#16444=CARTESIAN_POINT ( 'NONE',  ( -17.04047135212043784, -30.95583473709190159, 38.60742750791695954 ) ) ;
#16455=CARTESIAN_POINT ( 'NONE',  ( -10.31147837279037738, -22.25502639194775512, -4.119453415160654225E-17 ) ) ;
#16467=CARTESIAN_POINT ( 'NONE',  ( -11.35725562635144925, -18.02023567606020293, 15.20117750791695599 ) ) ;
#16471=CARTESIAN_POINT ( 'NONE',  ( -15.96867458239599635, -21.04416526290806999, 11.26757249208304579 ) ) ;
#16475=CARTESIAN_POINT ( 'NONE',  ( -17.31681416490115311, -26.07549068051209318, 23.29492750791696309 ) ) ;
#16490=CARTESIAN_POINT ( 'NONE',  ( -13.49542703274178379, -19.04416526290806289, 35.98242750791696665 ) ) ;
#16492=CARTESIAN_POINT ( 'NONE',  ( -17.64274437364855430, -28.24771351637087236, 23.07617750791695954 ) ) ;
#16498=CARTESIAN_POINT ( 'NONE',  ( -10.58745947852648328, -26.35725562635138530, 23.73632249208304046 ) ) ;
#16501=CARTESIAN_POINT ( 'NONE',  ( -17.68048971390462754, -22.64274437364856496, 10.61132249208304401 ) ) ;
#16504=CARTESIAN_POINT ( 'NONE',  ( -10.14701344837433616, -21.92759952878850527, -1.842058582387526229E-17 ) ) ;
#16506=CARTESIAN_POINT ( 'NONE',  ( -19.95583473709191580, -22.49542703274176603, 39.91992750791695954 ) ) ;
#16512=( LENGTH_UNIT ( ) NAMED_UNIT ( * ) SI_UNIT ( .MILLI., .METRE. ) );
#16517=CARTESIAN_POINT ( 'NONE',  ( -12.35725562635143682, -19.75228648362908501, -0.5488224920830419018 ) ) ;
#16518=CARTESIAN_POINT ( 'NONE',  ( -18.53959229564986799, -20.21908421996107563, 8.857427507916957765 ) ) ;
#16520=CARTESIAN_POINT ( 'NONE',  ( -19.99999999999999645, -24.16482700510261949, 10.17382249208304046 ) ) ;
#16522=CARTESIAN_POINT ( 'NONE',  ( -18.53959229564986799, -20.21908421996107563, 3.607427507916956877 ) ) ;
#16524=CARTESIAN_POINT ( 'NONE',  ( -18.78091578003889595, -27.53959229564985023, 18.04492750791695599 ) ) ;
#16535=CARTESIAN_POINT ( 'NONE',  ( -16.71081734191520596, -31.04416526290808065, 24.83007249208304046 ) ) ;
#16537=CARTESIAN_POINT ( 'NONE',  ( -10.75228648362912232, -21.35725562635138530, 1.861322492083040903 ) ) ;
#16540=CARTESIAN_POINT ( 'NONE',  ( -14.36097942780923731, -27.04416526290806999, 11.91992750791695954 ) ) ;
#16542=CARTESIAN_POINT ( 'NONE',  ( -15.16482700510264436, -16.99999999999997868, 6.236322492083039570 ) ) ;
#16553=CARTESIAN_POINT ( 'NONE',  ( -11.71628366038622104, -21.20848088107547014, 1.651559915991179495E-16 ) ) ;
#16564=CARTESIAN_POINT ( 'NONE',  ( -7.955834737091916686, -22.28918265808470522, 10.60742750791695599 ) ) ;
#16569=CARTESIAN_POINT ( 'NONE',  ( -15.96867458239599635, -21.04416526290806999, 16.51757249208304046 ) ) ;
#16574=CARTESIAN_POINT ( 'NONE',  ( -12.04416526290807887, -24.96867458239596260, 21.54492750791695954 ) ) ;
#16588=CARTESIAN_POINT ( 'NONE',  ( -20.04416526290808065, -25.17491895705300209, 34.23242750791695954 ) ) ;
#16590=CARTESIAN_POINT ( 'NONE',  ( -11.46040770435012668, -27.78091578003887463, 11.48242750791695954 ) ) ;
#16595=CARTESIAN_POINT ( 'NONE',  ( -13.49542703274174116, -28.95583473709188738, 24.39257249208303335 ) ) ;
#16600=CARTESIAN_POINT ( 'NONE',  ( -15.16482700510262482, -20.99999999999997513, 21.98632249208304046 ) ) ;
#16620=CARTESIAN_POINT ( 'NONE',  ( -20.04416526290808065, -25.17491895705300209, 23.73242750791694888 ) ) ;
#16621=CARTESIAN_POINT ( 'NONE',  ( -12.64274437364855252, -28.41254052147347053, 11.70117750791695777 ) ) ;
#16623=CARTESIAN_POINT ( 'NONE',  ( -16.50457296725825174, -19.04416526290807354, 21.76757249208304401 ) ) ;
#16626=CARTESIAN_POINT ( 'NONE',  ( -16.50457296725820555, -28.95583473709189448, 1.857427507916957765 ) ) ;
#16628=CARTESIAN_POINT ( 'NONE',  ( -15.16482700510259640, -28.99999999999998224, 12.13867750791695777 ) ) ;
#16644=CARTESIAN_POINT ( 'NONE',  ( -11.64274437364859693, -17.85540867095757989, 17.17382249208304046 ) ) ;
#16646=CARTESIAN_POINT ( 'NONE',  ( -10.75228648362912232, -21.35725562635138530, 17.61132249208304401 ) ) ;
#16649=CARTESIAN_POINT ( 'NONE',  ( -15.16482700510260706, -26.99999999999998579, 17.38867750791695954 ) ) ;
#16651=CARTESIAN_POINT ( 'NONE',  ( -22.04416526290809486, -22.28918265808477628, 10.39257249208303691 ) ) ;
#16668=CARTESIAN_POINT ( 'NONE',  ( -8.044165262908075320, -26.04047135212042718, 11.04492750791695777 ) ) ;
#16674=CARTESIAN_POINT ( 'NONE',  ( -17.31681416490117087, -21.92450931948788551, 21.33007249208304401 ) ) ;
#16675=CARTESIAN_POINT ( 'NONE',  ( -13.28918265808472299, -31.04416526290805933, 6.669927507916955989 ) ) ;
#16679=CARTESIAN_POINT ( 'NONE',  ( -15.16482700510260706, -26.99999999999998579, 17.38867750791695954 ) ) ;
#16691=CARTESIAN_POINT ( 'NONE',  ( -16.50457296725820555, -28.95583473709189448, 38.60742750791694533 ) ) ;
#16695=CARTESIAN_POINT ( 'NONE',  ( -13.49542703274178379, -19.04416526290806289, 20.23242750791696309 ) ) ;
#16698=CARTESIAN_POINT ( 'NONE',  ( -10.75228648362912232, -21.35725562635138530, 12.36132249208304046 ) ) ;
#16700=CARTESIAN_POINT ( 'NONE',  ( -16.35725562635141372, -26.68048971390461332, 14.54882249208304401 ) ) ;
#16717=CARTESIAN_POINT ( 'NONE',  ( -16.17491895705301275, -18.95583473709189803, 14.54492750791695421 ) ) ;
#16719=CARTESIAN_POINT ( 'NONE',  ( -19.99999999999999645, -24.16482700510261949, 25.92382249208304401 ) ) ;
#16722=CARTESIAN_POINT ( 'NONE',  ( -17.64274437364855430, -28.24771351637087236, 12.57617750791695777 ) ) ;
#16725=CARTESIAN_POINT ( 'NONE',  ( -16.17491895705301275, -18.95583473709189448, 19.79492750791695954 ) ) ;
#16738=CARTESIAN_POINT ( 'NONE',  ( -7.955834737091903364, -25.71081734191518464, 28.76757249208303691 ) ) ;
#16740=CARTESIAN_POINT ( 'NONE',  ( -19.99999999999999645, -24.16482700510261949, 4.923822492083040459 ) ) ;
#16742=CARTESIAN_POINT ( 'NONE',  ( -15.63902057219076269, -20.95583473709189448, 19.79492750791695954 ) ) ;
#16744=CARTESIAN_POINT ( 'NONE',  ( -20.24501739517669563, -18.99630608921239627, 16.08007249208304046 ) ) ;
#16763=CARTESIAN_POINT ( 'NONE',  ( -14.83517299489740715, -16.99999999999997868, 9.513677507916955989 ) ) ;
#16768=CARTESIAN_POINT ( 'NONE',  ( -15.63902057219073605, -27.04416526290807710, 19.58007249208304046 ) ) ;
#16769=CARTESIAN_POINT ( 'NONE',  ( -14.83517299489740715, -16.99999999999997868, 20.01367750791695954 ) ) ;
#16774=CARTESIAN_POINT ( 'NONE',  ( -12.68318583509884157, -21.92450931948787485, 15.41992750791695954 ) ) ;
#16790=CARTESIAN_POINT ( 'NONE',  ( -20.04416526290808065, -25.17491895705300209, 18.48242750791695954 ) ) ;
#16793=CARTESIAN_POINT ( 'NONE',  ( -9.955834737091903364, -25.17491895705294880, 13.01757249208304223 ) ) ;
#16796=CARTESIAN_POINT ( 'NONE',  ( -12.04416526290808420, -23.03132541760398766, 12.58007249208304401 ) ) ;
#16814=CARTESIAN_POINT ( 'NONE',  ( -13.49542703274178379, -19.04416526290806289, 20.23242750791696309 ) ) ;
#16818=CARTESIAN_POINT ( 'NONE',  ( -16.17491895705296656, -29.04416526290807710, 14.33007249208304046 ) ) ;
#16821=CARTESIAN_POINT ( 'NONE',  ( -13.82508104294698192, -29.04416526290806644, 22.41992750791695244 ) ) ;
#16823=CARTESIAN_POINT ( 'NONE',  ( -18.78091578003889595, -27.53959229564985023, 12.79492750791695599 ) ) ;
#16835=CARTESIAN_POINT ( 'NONE',  ( -18.64274437364860049, -18.02023567606023491, 32.04882249208304046 ) ) ;
#16836=MANIFOLD_SOLID_BREP ( 'Cavity1', #12604 ) ;
#16838=CARTESIAN_POINT ( 'NONE',  ( -15.16482700510263371, -18.99999999999997868, 11.48632249208304046 ) ) ;
#16841=CARTESIAN_POINT ( 'NONE',  ( -12.92450931948788906, -26.31681416490114245, 27.23242750791697020 ) ) ;
#16843=CARTESIAN_POINT ( 'NONE',  ( -9.996306089212408708, -18.75498260482328661, 22.64257249208304046 ) ) ;
#16861=CARTESIAN_POINT ( 'NONE',  ( -11.35725562635144925, -18.02023567606020293, 25.70117750791695599 ) ) ;
#16865=CARTESIAN_POINT ( 'NONE',  ( -15.16482700510262482, -20.99999999999997513, 32.48632249208304756 ) ) ;
#16866=CARTESIAN_POINT ( 'NONE',  ( -9.020235676060220698, -27.64274437364852588, 21.76367750791695954 ) ) ;
#16870=CARTESIAN_POINT ( 'NONE',  ( -11.95583473709191047, -23.36097942780921954, 10.60742750791695954 ) ) ;
#16879=CARTESIAN_POINT ( 'NONE',  ( 0.000000000000000000, 0.000000000000000000, 0.000000000000000000 ) ) ;
#16887=CARTESIAN_POINT ( 'NONE',  ( -19.24771351637089367, -21.35725562635142438, 24.38867750791695954 ) ) ;
#16891=CARTESIAN_POINT ( 'NONE',  ( -9.999999999999994671, -23.83517299489734143, 12.79882249208304046 ) ) ;
#16893=CARTESIAN_POINT ( 'NONE',  ( -14.03132541760400009, -26.95583473709189448, 13.89257249208304401 ) ) ;
#16912=CARTESIAN_POINT ( 'NONE',  ( -10.75228648362910100, -26.64274437364854009, 21.76367750791695599 ) ) ;
#16916=CARTESIAN_POINT ( 'NONE',  ( -18.78091578003892081, -20.46040770435013556, 21.33007249208303691 ) ) ;
#16919=CARTESIAN_POINT ( 'NONE',  ( -13.82508104294698192, -29.04416526290806644, 17.16992750791694888 ) ) ;
#16922=CARTESIAN_POINT ( 'NONE',  ( -13.82508104294698015, -29.04416526290806289, 22.41992750791695599 ) ) ;
#16925=CARTESIAN_POINT ( 'NONE',  ( -12.35725562635140307, -28.24771351637085459, 29.42382249208304401 ) ) ;
#16936=CARTESIAN_POINT ( 'NONE',  ( -15.16482700510264436, -16.99999999999997868, 27.23632249208303691 ) ) ;
#16940=CARTESIAN_POINT ( 'NONE',  ( -19.24771351637086880, -26.64274437364857206, 14.98632249208304046 ) ) ;
#16942=CARTESIAN_POINT ( 'NONE',  ( -12.68318583509884157, -21.92450931948787485, 36.41992750791695954 ) ) ;
#16944=CARTESIAN_POINT ( 'NONE',  ( -20.97976432393974022, -27.64274437364858628, 14.98632249208303868 ) ) ;
#16964=CARTESIAN_POINT ( 'NONE',  ( -22.04416526290807710, -25.71081734191525925, 23.73242750791695954 ) ) ;
#16969=CARTESIAN_POINT ( 'NONE',  ( -17.07549068051208963, -26.31681416490115311, 35.76757249208304756 ) ) ;
#16970=CARTESIAN_POINT ( 'NONE',  ( -15.16482700510258574, -30.99999999999998224, 22.63867750791695954 ) ) ;
#16974=CARTESIAN_POINT ( 'NONE',  ( -14.03132541760401786, -21.04416526290806289, 30.73242750791696309 ) ) ;
#16993=CARTESIAN_POINT ( 'NONE',  ( -13.49542703274178379, -19.04416526290806289, 25.48242750791694888 ) ) ;
#16996=CARTESIAN_POINT ( 'NONE',  ( -15.16482700510263371, -18.99999999999997868, 32.48632249208304046 ) ) ;
#16997=CARTESIAN_POINT ( 'NONE',  ( -16.35725562635141372, -26.68048971390461332, 19.79882249208304046 ) ) ;
#17013=CARTESIAN_POINT ( 'NONE',  ( -19.41254052147348830, -26.35725562635142083, 18.26367750791695599 ) ) ;
#17015=CARTESIAN_POINT ( 'NONE',  ( -17.35725562635140307, -28.41254052147349185, 14.54882249208304046 ) ) ;
#17016=( BOUNDED_SURFACE ( )  B_SPLINE_SURFACE ( 3, 2, ( 
 ( #4174, #2889, #16517, #2785, #14754, #8764, #13068, #1328, #10522, #1219, #17897, #13369, #7493, #7298, #19361, #10231, #14849, #5835, #16122, #11799, #13264, #19266, #3080, #4565, #14553, #4469, #1124, #13469, #19066, #10421, #14951, #17793, #52, #4366, #1422, #7104, #10325, #1524, #16323, #19167, #8865, #5638, #8961, #5738, #7398, #4269, #5929, #2691, #16416, #2981, #17597, #8667, #7200, #13173, #3478, #9255, #10817, #13662, #1814, #244, #4860, #18090, #18293, #9346, #10619, #7597, #3379, #18389, #11014, #10723, #15242, #16717, #13563, #3284, #5054, #9161, #6425, #7901, #2005, #7794, #13865, #4773, #15337, #346, #4662, #6332, #13764, #12298, #17013, #12484, #536, #12392, #9061, #7995, #144, #4958, #9452, #16814, #13962, #1915, #441, #6519, #10914, #15440, #16912, #6228, #18485, #15049, #1627, #12193, #6130, #18194, #12092, #16620, #3187, #15145, #1713, #7696, #18581, #9640, #17376, #3764, #5334, #8189, #15730, #14157, #18762, #12589, #12766, #3858, #5147, #2107, #17292, #12864, #6620, #5427, #8091, #910, #15625, #14336, #15536, #727, #9734, #14056, #12952, #15909, #6705, #6986, #8368, #2290, #11107, #6891, #8276, #17200, #14246, #17105, #9820, #2194, #3669, #12676, #5518, #18678, #5244, #11197, #3952, #817, #6801, #18865, #629, #11296, #15816, #2383, #11385, #9914, #2471, #18951, #8461, #14437, #1011, #11480, #3570, #9543, #2666, #4720, #1399, #2866, #8647, #8554, #9210, #17769, #8845, #14529, #16100 ),
 ( #1307, #13348, #1100, #7082, #19148, #4343, #16014, #13045, #7280, #1770, #5616, #4246, #19044, #11578, #10300, #17576, #14629, #10676, #7376, #14830, #1193, #4154, #15202, #16293, #19342, #10104, #7176, #5908, #10008, #13245, #13149, #11874, #18142, #5718, #17468, #16675, #3238, #11677, #17668, #19243, #10205, #7752, #13717, #4043, #2572, #11777, #5811, #294, #6279, #16196, #2763, #8737, #14728, #6381, #9592, #397, #15486, #17057, #15396, #12250, #9308, #8137, #12632, #6475, #18628, #10766, #5195, #11153, #9497, #12343, #15293, #14009, #17151, #15678, #18342, #2056, #1963, #14110, #18247, #3712, #769, #15582, #9686, #489, #3340, #2248, #8237, #4912, #7949, #7852, #2149, #9401, #1866, #10965, #685, #8047, #16769, #3429, #6668, #580, #18438, #14204, #13912, #12442, #16866, #12539, #10871, #5007, #16970, #3530, #4819, #6573, #13818, #3622, #18540, #5107, #11061, #14293, #1053, #5384, #2337, #11342, #8692, #3901, #860, #7030, #17334, #8322, #9871, #14675, #15865, #6839, #2425, #7129, #3998, #9956, #2613, #3813, #15773, #8408, #13000, #5282, #17244, #15958, #10148, #12812, #12909, #18810, #14383, #19001, #959, #6939, #13096, #10058, #11524, #18905, #9780, #17619, #5567, #17518, #5469, #11434, #4098, #18718, #2523, #17428, #8597, #14581, #8505, #6753, #16053, #19095, #14482, #1152, #5665, #11629, #4196, #2719, #12721, #11240, #16150, #16444, #3012, #3217, #4497, #6061, #8989, #8890, #14784, #18020, #8796, #10452, #12024 ),
 ( #14878, #7628, #14976, #5863, #1452, #13592, #15080, #11823, #1549, #4397, #7525, #10253, #10357, #13499, #4595, #10553, #16242, #7325, #1654, #7425, #81, #17819, #13392, #16351, #16542, #2815, #3110, #9091, #1353, #19193, #177, #6163, #4296, #12123, #5760, #18118, #13290, #4690, #13199, #2916, #19388, #11722, #10648, #16651, #5961, #9189, #1251, #11932, #19293, #7230, #17719, #17925, #11131, #7729, #9477, #4798, #4886, #8022, #6548, #5083, #10747, #1839, #9566, #15369, #16944, #371, #7926, #6359, #10941, #16744, #4984, #15463, #3314, #13692, #2031, #11040, #18221, #17038, #268, #12514, #7823, #18515, #6254, #12322, #1943, #12220, #5170, #8113, #18318, #18606, #559, #13889, #15270, #14086, #660, #10849, #17129, #9284, #3595, #16843, #15561, #13791, #3405, #3692, #9374, #2129, #6646, #465, #6451, #3508, #12611, #13989, #15177, #12420, #18418, #1744, #6917, #5547, #840, #17404, #5361, #16036, #11321, #9936, #12698, #15653, #4070, #17223, #7109, #6821, #2224, #12889, #3978, #9845, #13071, #12788, #18701, #15932, #11603, #17315, #15841, #3879, #8216, #2405, #5643, #9759, #7010, #8485, #2596, #8387, #14463, #14360, #2498, #935, #5263, #18888, #5450, #11410, #17600, #19069, #1127, #12978, #9662, #8577, #14183, #11503, #10038, #1035, #14556, #18978, #17494, #748, #6731, #11218, #3792, #14271, #15753, #2315, #8298, #18786, #19364, #7301, #7600, #8964, #16326, #4272, #3083, #9064, #19269, #149, #16125, #14953, #14758 ),
 ( #15052, #10234, #5741, #5932, #1630, #11903, #16419, #17796, #14853, #17902, #1426, #55, #1331, #4474, #5838, #10525, #11802, #10425, #7204, #10128, #17995, #11701, #13568, #13268, #2694, #7401, #2984, #4369, #6134, #10330, #13177, #1527, #12095, #2894, #8868, #13372, #8670, #7496, #4177, #16218, #13472, #6040, #16520, #11997, #4568, #14653, #1222, #19170, #17694, #2790, #8767, #10819, #14058, #2109, #9546, #2007, #18093, #11016, #3190, #13964, #18489, #16818, #17015, #1917, #18391, #3573, #6334, #5057, #7903, #3287, #18295, #15538, #12487, #9259, #13867, #1817, #12394, #7699, #7796, #10917, #9454, #7998, #13665, #4775, #8093, #4863, #443, #15245, #3382, #13767, #6428, #246, #4961, #16916, #6230, #16623, #3480, #538, #1718, #6521, #9164, #15442, #10725, #633, #10622, #348, #9349, #15147, #6623, #4665, #12300, #15340, #12195, #18196, #16719, #12591, #11387, #5522, #729, #6708, #14339, #12679, #6988, #8556, #18583, #11111, #6894, #8370, #912, #14531, #15819, #17381, #12866, #819, #18681, #9916, #5246, #2385, #3954, #15733, #5149, #9642, #8463, #12954, #6804, #18953, #17107, #11482, #17470, #9824, #11199, #15627, #18867, #4046, #16016, #17202, #5429, #2294, #14439, #3671, #10012, #1103, #15911, #2575, #12768, #2197, #8192, #14161, #3767, #8278, #9736, #2475, #14248, #18764, #11298, #1013, #5337, #17294, #3860, #2962, #4345, #13248, #29, #2765, #4249, #11679, #7379, #7179, #17671, #10207, #14631, #4450, #17771 ),
 ( #1402, #5721, #2669, #16198, #9042, #8742, #1197, #14731, #7472, #10303, #16298, #8941, #4156, #16102, #1309, #13351, #5619, #17579, #2868, #10503, #13152, #19245, #8649, #19150, #19344, #7282, #5815, #13445, #10404, #11877, #11779, #10107, #17970, #5910, #17875, #8847, #14832, #16398, #19046, #14934, #1506, #6017, #11977, #4544, #16501, #15029, #3064, #7084, #13049, #11581, #3166, #3366, #18466, #16796, #13848, #15228, #12282, #9330, #18275, #16893, #12175, #15319, #16700, #7977, #3266, #1896, #4647, #7579, #15427, #9143, #5035, #18174, #13547, #4842, #7882, #1796, #10996, #4752, #10601, #424, #3557, #9236, #7778, #13744, #126, #328, #16997, #1695, #18374, #6408, #13943, #6311, #12373, #10798, #4941, #10898, #16600, #3460, #9434, #1991, #9526, #1605, #12465, #517, #6110, #6505, #12076, #18074, #15129, #7676, #13644, #228, #6212, #10705, #3744, #2455, #5312, #713, #15709, #8440, #9900, #6694, #11274, #18661, #9806, #5135, #5228, #8351, #6871, #5412, #11091, #2177, #15891, #2277, #17274, #12660, #8263, #11182, #3840, #17087, #15800, #2366, #3653, #14038, #14323, #11366, #18568, #17361, #608, #12842, #8167, #18843, #8075, #17180, #14231, #6604, #5498, #14416, #9717, #18930, #891, #799, #15607, #991, #6967, #6787, #11463, #12572, #12752, #18748, #12936, #3930, #17454, #4024, #15516, #14139, #2089, #9622, #17553, #7354, #1284, #5594, #1381, #10180, #4225, #16178, #4134, #4323, #8626, #11556, #14612, #11960, #7156 ),
 ( #7452, #5792, #2846, #2746, #7261, #11752, #13228, #5890, #1177, #17752, #5701, #16380, #11660, #10280, #13030, #15993, #4425, #10087, #13420, #13127, #2554, #19223, #16274, #8718, #6, #19126, #19028, #8828, #17952, #17650, #14707, #14813, #8536, #13323, #5994, #16080, #19323, #11850, #2943, #17853, #10387, #8919, #14910, #1484, #2644, #9987, #14510, #1081, #7060, #7953, #15400, #7856, #4524, #16870, #9018, #402, #4917, #3242, #3433, #7757, #4823, #9406, #12150, #10876, #13721, #9119, #4724, #1970, #18346, #15108, #298, #7655, #18252, #13530, #13621, #16774, #15298, #13825, #107, #10581, #13916, #10681, #6286, #1678, #16679, #206, #12256, #6090, #10771, #3344, #12054, #3044, #9312, #6385, #7553, #12348, #15004, #493, #4626, #6194, #18052, #1870, #18149, #16574, #9215, #6479, #12446, #1581, #15206, #10482, #1774, #16475, #3141, #14116, #15587, #3627, #18723, #18546, #9597, #2155, #6578, #16038, #9691, #14014, #10041, #18634, #12637, #5202, #12545, #12728, #17066, #586, #8143, #1226, #690, #5113, #6674, #19072, #15684, #2254, #14559, #15492, #8052, #11158, #5287, #16974, #9504, #8242, #2699, #11066, #17156, #3718, #14209, #11246, #775, #6759, #5646, #2598, #4074, #17249, #2061, #10131, #8579, #1132, #7111, #13074, #11606, #10971, #17602, #4179, #16127, #8673, #14655, #18443, #7207, #5011, #3534, #7303, #14955, #13270, #7604, #9167, #13180, #11703, #7499, #8968, #1529, #15151, #16421, #17997, #13476, #1428, #19271 ),
 ( #10237, #9067, #13570, #7405, #151, #17696, #6136, #12099, #10428, #1333, #16222, #59, #18095, #16626, #5842, #2986, #16329, #15055, #19172, #4667, #1721, #16522, #10624, #13374, #4276, #3192, #10529, #2793, #14855, #5743, #8770, #1633, #14761, #11804, #17799, #6042, #4374, #11999, #4570, #19366, #4476, #3085, #10333, #2896, #8870, #5936, #11908, #17904, #9351, #8000, #10727, #13668, #2111, #15249, #5152, #4865, #248, #4963, #2011, #7905, #11113, #18297, #16722, #15444, #9644, #15343, #13870, #1922, #6232, #445, #3674, #7798, #5060, #6525, #636, #6430, #12490, #3384, #13966, #18396, #3291, #10919, #12396, #16919, #15630, #17109, #18585, #11018, #7701, #6626, #12198, #3577, #8095, #3483, #12593, #9458, #540, #18200, #18492, #14062, #17020, #12302, #9549, #4777, #9261, #10823, #15540, #16821, #1819, #13770, #350, #6337, #12961, #11487, #17204, #8281, #16020, #2387, #3957, #6806, #14343, #12771, #17384, #11201, #11390, #2478, #3770, #731, #15916, #17475, #5249, #4050, #6711, #18957, #14251, #5526, #14163, #18766, #8374, #12681, #11586, #14537, #5339, #5623, #6992, #915, #2296, #1108, #7088, #17299, #17584, #18683, #10017, #11301, #6898, #2579, #9919, #9741, #3862, #8559, #18870, #12871, #13053, #9827, #15821, #5434, #8467, #822, #14443, #1018, #15735, #19051, #4160, #10111, #2202, #8195, #10309, #2874, #4253, #10409, #14736, #11683, #1315, #18080, #13253, #10211, #5820, #16506, #13356, #19349, #11982, #13157, #5725 ) ),
 .UNSPECIFIED., .T., .F., .F. ) 
 B_SPLINE_SURFACE_WITH_KNOTS ( ( 4, 3, 4 ),
 ( 3, 2, 2, 2, 2, 2, 2, 2, 2, 2, 2, 2, 2, 2, 2, 2, 2, 2, 2, 2, 2, 2, 2, 2, 2, 2, 2, 2, 2, 2, 2, 2, 2, 2, 2, 2, 2, 2, 2, 2, 2, 2, 2, 2, 2, 2, 2, 2, 2, 2, 2, 2, 2, 2, 2, 2, 2, 2, 2, 2, 2, 2, 2, 2, 2, 2, 2, 2, 2, 2, 2, 2, 2, 2, 2, 2, 2, 2, 2, 2, 2, 2, 2, 2, 2, 2, 2, 2, 2, 2, 2, 2, 2, 2, 2, 2, 3 ),
 ( 0.000000000000000000, 0.5000000000000000000, 1.000000000000000000 ),
 ( 0.000000000000000000, 0.01041666666666666609, 0.02083333333333333218, 0.03125000000000000000, 0.04166666666666666435, 0.05208333333333333565, 0.06250000000000000000, 0.07291666666666667129, 0.08333333333333332871, 0.09375000000000000000, 0.1041666666666666713, 0.1145833333333333287, 0.1250000000000000000, 0.1354166666666666574, 0.1458333333333333426, 0.1562500000000000000, 0.1666666666666666574, 0.1770833333333333426, 0.1875000000000000000, 0.1979166666666666574, 0.2083333333333333426, 0.2187500000000000000, 0.2291666666666666574, 0.2395833333333333426, 0.2500000000000000000, 0.2604166666666666852, 0.2708333333333333148, 0.2812500000000000000, 0.2916666666666666852, 0.3020833333333333148, 0.3125000000000000000, 0.3229166666666666852, 0.3333333333333333148, 0.3437500000000000000, 0.3541666666666666852, 0.3645833333333333148, 0.3750000000000000000, 0.3854166666666666852, 0.3958333333333333148, 0.4062500000000000000, 0.4166666666666666852, 0.4270833333333333148, 0.4375000000000000000, 0.4479166666666666852, 0.4583333333333333148, 0.4687500000000000000, 0.4791666666666666852, 0.4895833333333333148, 0.5000000000000000000, 0.5104166666666666297, 0.5208333333333333703, 0.5312500000000000000, 0.5416666666666666297, 0.5520833333333333703, 0.5625000000000000000, 0.5729166666666666297, 0.5833333333333333703, 0.5937500000000000000, 0.6041666666666666297, 0.6145833333333333703, 0.6250000000000000000, 0.6354166666666666297, 0.6458333333333333703, 0.6562500000000000000, 0.6666666666666666297, 0.6770833333333333703, 0.6875000000000000000, 0.6979166666666666297, 0.7083333333333333703, 0.7187500000000000000, 0.7291666666666666297, 0.7395833333333333703, 0.7500000000000000000, 0.7604166666666666297, 0.7708333333333333703, 0.7812500000000000000, 0.7916666666666666297, 0.8020833333333333703, 0.8125000000000000000, 0.8229166666666666297, 0.8333333333333333703, 0.8437500000000000000, 0.8541666666666666297, 0.8645833333333333703, 0.8750000000000000000, 0.8854166666666666297, 0.8958333333333333703, 0.9062500000000000000, 0.9166666666666666297, 0.9270833333333333703, 0.9375000000000000000, 0.9479166666666666297, 0.9583333333333333703, 0.9687500000000000000, 0.9791666666666666297, 0.9895833333333333703, 1.000000000000000000 ),
 .UNSPECIFIED. ) 
 GEOMETRIC_REPRESENTATION_ITEM ( )  RATIONAL_B_SPLINE_SURFACE ( (
 ( 1.000000000000000000, 0.9659258262890683122, 1.000000000000000000, 0.9659258262890683122, 1.000000000000000000, 0.9659258262890683122, 1.000000000000000000, 0.9659258262890683122, 1.000000000000000000, 0.9659258262890683122, 1.000000000000000000, 0.9659258262890683122, 1.000000000000000000, 0.9659258262890683122, 1.000000000000000000, 0.9659258262890683122, 1.000000000000000000, 0.9659258262890683122, 1.000000000000000000, 0.9659258262890683122, 1.000000000000000000, 0.9659258262890683122, 1.000000000000000000, 0.9659258262890683122, 1.000000000000000000, 0.9659258262890683122, 1.000000000000000000, 0.9659258262890683122, 1.000000000000000000, 0.9659258262890683122, 1.000000000000000000, 0.9659258262890683122, 1.000000000000000000, 0.9659258262890683122, 1.000000000000000000, 0.9659258262890683122, 1.000000000000000000, 0.9659258262890683122, 1.000000000000000000, 0.9659258262890683122, 1.000000000000000000, 0.9659258262890683122, 1.000000000000000000, 0.9659258262890683122, 1.000000000000000000, 0.9659258262890683122, 1.000000000000000000, 0.9659258262890683122, 1.000000000000000000, 0.9659258262890683122, 1.000000000000000000, 0.9659258262890683122, 1.000000000000000000, 0.9659258262890683122, 1.000000000000000000, 0.9659258262890683122, 1.000000000000000000, 0.9659258262890683122, 1.000000000000000000, 0.9659258262890683122, 1.000000000000000000, 0.9659258262890683122, 1.000000000000000000, 0.9659258262890683122, 1.000000000000000000, 0.9659258262890683122, 1.000000000000000000, 0.9659258262890683122, 1.000000000000000000, 0.9659258262890683122, 1.000000000000000000, 0.9659258262890683122, 1.000000000000000000, 0.9659258262890683122, 1.000000000000000000, 0.9659258262890683122, 1.000000000000000000, 0.9659258262890683122, 1.000000000000000000, 0.9659258262890683122, 1.000000000000000000, 0.9659258262890683122, 1.000000000000000000, 0.9659258262890683122, 1.000000000000000000, 0.9659258262890683122, 1.000000000000000000, 0.9659258262890683122, 1.000000000000000000, 0.9659258262890683122, 1.000000000000000000, 0.9659258262890683122, 1.000000000000000000, 0.9659258262890683122, 1.000000000000000000, 0.9659258262890683122, 1.000000000000000000, 0.9659258262890683122, 1.000000000000000000, 0.9659258262890683122, 1.000000000000000000, 0.9659258262890683122, 1.000000000000000000, 0.9659258262890683122, 1.000000000000000000, 0.9659258262890683122, 1.000000000000000000, 0.9659258262890683122, 1.000000000000000000, 0.9659258262890683122, 1.000000000000000000, 0.9659258262890683122, 1.000000000000000000, 0.9659258262890683122, 1.000000000000000000, 0.9659258262890683122, 1.000000000000000000, 0.9659258262890683122, 1.000000000000000000, 0.9659258262890683122, 1.000000000000000000, 0.9659258262890683122, 1.000000000000000000, 0.9659258262890683122, 1.000000000000000000, 0.9659258262890683122, 1.000000000000000000, 0.9659258262890683122, 1.000000000000000000, 0.9659258262890683122, 1.000000000000000000, 0.9659258262890683122, 1.000000000000000000, 0.9659258262890683122, 1.000000000000000000, 0.9659258262890683122, 1.000000000000000000, 0.9659258262890683122, 1.000000000000000000, 0.9659258262890683122, 1.000000000000000000, 0.9659258262890683122, 1.000000000000000000, 0.9659258262890683122, 1.000000000000000000, 0.9659258262890683122, 1.000000000000000000, 0.9659258262890683122, 1.000000000000000000, 0.9659258262890683122, 1.000000000000000000, 0.9659258262890683122, 1.000000000000000000, 0.9659258262890683122, 1.000000000000000000, 0.9659258262890683122, 1.000000000000000000, 0.9659258262890683122, 1.000000000000000000, 0.9659258262890683122, 1.000000000000000000, 0.9659258262890683122, 1.000000000000000000, 0.9659258262890683122, 1.000000000000000000, 0.9659258262890683122, 1.000000000000000000, 0.9659258262890683122, 1.000000000000000000, 0.9659258262890683122, 1.000000000000000000, 0.9659258262890683122, 1.000000000000000000, 0.9659258262890683122, 1.000000000000000000, 0.9659258262890683122, 1.000000000000000000, 0.9659258262890683122, 1.000000000000000000, 0.9659258262890683122, 1.000000000000000000, 0.9659258262890683122, 1.000000000000000000, 0.9659258262890683122, 1.000000000000000000, 0.9659258262890683122, 1.000000000000000000, 0.9659258262890683122, 1.000000000000000000, 0.9659258262890683122, 1.000000000000000000, 0.9659258262890683122, 1.000000000000000000),
 ( 0.3333333333333333703, 0.3219752754296894559, 0.3333333333333333703, 0.3219752754296894559, 0.3333333333333333703, 0.3219752754296894559, 0.3333333333333333703, 0.3219752754296894559, 0.3333333333333333703, 0.3219752754296894559, 0.3333333333333333703, 0.3219752754296894559, 0.3333333333333333703, 0.3219752754296894559, 0.3333333333333333703, 0.3219752754296894559, 0.3333333333333333703, 0.3219752754296894559, 0.3333333333333333703, 0.3219752754296894559, 0.3333333333333333703, 0.3219752754296894559, 0.3333333333333333703, 0.3219752754296894559, 0.3333333333333333703, 0.3219752754296894559, 0.3333333333333333703, 0.3219752754296894559, 0.3333333333333333703, 0.3219752754296894559, 0.3333333333333333703, 0.3219752754296894559, 0.3333333333333333703, 0.3219752754296894559, 0.3333333333333333703, 0.3219752754296894559, 0.3333333333333333703, 0.3219752754296894559, 0.3333333333333333703, 0.3219752754296894559, 0.3333333333333333703, 0.3219752754296894559, 0.3333333333333333703, 0.3219752754296894559, 0.3333333333333333703, 0.3219752754296894559, 0.3333333333333333703, 0.3219752754296894559, 0.3333333333333333703, 0.3219752754296894559, 0.3333333333333333703, 0.3219752754296894559, 0.3333333333333333703, 0.3219752754296894559, 0.3333333333333333703, 0.3219752754296894559, 0.3333333333333333703, 0.3219752754296894559, 0.3333333333333333703, 0.3219752754296894559, 0.3333333333333333703, 0.3219752754296894559, 0.3333333333333333703, 0.3219752754296894559, 0.3333333333333333703, 0.3219752754296894559, 0.3333333333333333703, 0.3219752754296894559, 0.3333333333333333703, 0.3219752754296894559, 0.3333333333333333703, 0.3219752754296894559, 0.3333333333333333703, 0.3219752754296894559, 0.3333333333333333703, 0.3219752754296894559, 0.3333333333333333703, 0.3219752754296894559, 0.3333333333333333703, 0.3219752754296894559, 0.3333333333333333703, 0.3219752754296894559, 0.3333333333333333703, 0.3219752754296894559, 0.3333333333333333703, 0.3219752754296894559, 0.3333333333333333703, 0.3219752754296894559, 0.3333333333333333703, 0.3219752754296894559, 0.3333333333333333703, 0.3219752754296894559, 0.3333333333333333703, 0.3219752754296894559, 0.3333333333333333703, 0.3219752754296894559, 0.3333333333333333703, 0.3219752754296894559, 0.3333333333333333703, 0.3219752754296894559, 0.3333333333333333703, 0.3219752754296894559, 0.3333333333333333703, 0.3219752754296894559, 0.3333333333333333703, 0.3219752754296894559, 0.3333333333333333703, 0.3219752754296894559, 0.3333333333333333703, 0.3219752754296894559, 0.3333333333333333703, 0.3219752754296894559, 0.3333333333333333703, 0.3219752754296894559, 0.3333333333333333703, 0.3219752754296894559, 0.3333333333333333703, 0.3219752754296894559, 0.3333333333333333703, 0.3219752754296894559, 0.3333333333333333703, 0.3219752754296894559, 0.3333333333333333703, 0.3219752754296894559, 0.3333333333333333703, 0.3219752754296894559, 0.3333333333333333703, 0.3219752754296894559, 0.3333333333333333703, 0.3219752754296894559, 0.3333333333333333703, 0.3219752754296894559, 0.3333333333333333703, 0.3219752754296894559, 0.3333333333333333703, 0.3219752754296894559, 0.3333333333333333703, 0.3219752754296894559, 0.3333333333333333703, 0.3219752754296894559, 0.3333333333333333703, 0.3219752754296894559, 0.3333333333333333703, 0.3219752754296894559, 0.3333333333333333703, 0.3219752754296894559, 0.3333333333333333703, 0.3219752754296894559, 0.3333333333333333703, 0.3219752754296894559, 0.3333333333333333703, 0.3219752754296894559, 0.3333333333333333703, 0.3219752754296894559, 0.3333333333333333703, 0.3219752754296894559, 0.3333333333333333703, 0.3219752754296894559, 0.3333333333333333703, 0.3219752754296894559, 0.3333333333333333703, 0.3219752754296894559, 0.3333333333333333703, 0.3219752754296894559, 0.3333333333333333703, 0.3219752754296894559, 0.3333333333333333703, 0.3219752754296894559, 0.3333333333333333703, 0.3219752754296894559, 0.3333333333333333703, 0.3219752754296894559, 0.3333333333333333703, 0.3219752754296894559, 0.3333333333333333703, 0.3219752754296894559, 0.3333333333333333703, 0.3219752754296894559, 0.3333333333333333703, 0.3219752754296894559, 0.3333333333333333703, 0.3219752754296894559, 0.3333333333333333703, 0.3219752754296894559, 0.3333333333333333703, 0.3219752754296894559, 0.3333333333333333703, 0.3219752754296894559, 0.3333333333333333703, 0.3219752754296894559, 0.3333333333333333703, 0.3219752754296894559, 0.3333333333333333703),
 ( 0.3333333333333333703, 0.3219752754296894559, 0.3333333333333333703, 0.3219752754296894559, 0.3333333333333333703, 0.3219752754296894559, 0.3333333333333333703, 0.3219752754296894559, 0.3333333333333333703, 0.3219752754296894559, 0.3333333333333333703, 0.3219752754296894559, 0.3333333333333333703, 0.3219752754296894559, 0.3333333333333333703, 0.3219752754296894559, 0.3333333333333333703, 0.3219752754296894559, 0.3333333333333333703, 0.3219752754296894559, 0.3333333333333333703, 0.3219752754296894559, 0.3333333333333333703, 0.3219752754296894559, 0.3333333333333333703, 0.3219752754296894559, 0.3333333333333333703, 0.3219752754296894559, 0.3333333333333333703, 0.3219752754296894559, 0.3333333333333333703, 0.3219752754296894559, 0.3333333333333333703, 0.3219752754296894559, 0.3333333333333333703, 0.3219752754296894559, 0.3333333333333333703, 0.3219752754296894559, 0.3333333333333333703, 0.3219752754296894559, 0.3333333333333333703, 0.3219752754296894559, 0.3333333333333333703, 0.3219752754296894559, 0.3333333333333333703, 0.3219752754296894559, 0.3333333333333333703, 0.3219752754296894559, 0.3333333333333333703, 0.3219752754296894559, 0.3333333333333333703, 0.3219752754296894559, 0.3333333333333333703, 0.3219752754296894559, 0.3333333333333333703, 0.3219752754296894559, 0.3333333333333333703, 0.3219752754296894559, 0.3333333333333333703, 0.3219752754296894559, 0.3333333333333333703, 0.3219752754296894559, 0.3333333333333333703, 0.3219752754296894559, 0.3333333333333333703, 0.3219752754296894559, 0.3333333333333333703, 0.3219752754296894559, 0.3333333333333333703, 0.3219752754296894559, 0.3333333333333333703, 0.3219752754296894559, 0.3333333333333333703, 0.3219752754296894559, 0.3333333333333333703, 0.3219752754296894559, 0.3333333333333333703, 0.3219752754296894559, 0.3333333333333333703, 0.3219752754296894559, 0.3333333333333333703, 0.3219752754296894559, 0.3333333333333333703, 0.3219752754296894559, 0.3333333333333333703, 0.3219752754296894559, 0.3333333333333333703, 0.3219752754296894559, 0.3333333333333333703, 0.3219752754296894559, 0.3333333333333333703, 0.3219752754296894559, 0.3333333333333333703, 0.3219752754296894559, 0.3333333333333333703, 0.3219752754296894559, 0.3333333333333333703, 0.3219752754296894559, 0.3333333333333333703, 0.3219752754296894559, 0.3333333333333333703, 0.3219752754296894559, 0.3333333333333333703, 0.3219752754296894559, 0.3333333333333333703, 0.3219752754296894559, 0.3333333333333333703, 0.3219752754296894559, 0.3333333333333333703, 0.3219752754296894559, 0.3333333333333333703, 0.3219752754296894559, 0.3333333333333333703, 0.3219752754296894559, 0.3333333333333333703, 0.3219752754296894559, 0.3333333333333333703, 0.3219752754296894559, 0.3333333333333333703, 0.3219752754296894559, 0.3333333333333333703, 0.3219752754296894559, 0.3333333333333333703, 0.3219752754296894559, 0.3333333333333333703, 0.3219752754296894559, 0.3333333333333333703, 0.3219752754296894559, 0.3333333333333333703, 0.3219752754296894559, 0.3333333333333333703, 0.3219752754296894559, 0.3333333333333333703, 0.3219752754296894559, 0.3333333333333333703, 0.3219752754296894559, 0.3333333333333333703, 0.3219752754296894559, 0.3333333333333333703, 0.3219752754296894559, 0.3333333333333333703, 0.3219752754296894559, 0.3333333333333333703, 0.3219752754296894559, 0.3333333333333333703, 0.3219752754296894559, 0.3333333333333333703, 0.3219752754296894559, 0.3333333333333333703, 0.3219752754296894559, 0.3333333333333333703, 0.3219752754296894559, 0.3333333333333333703, 0.3219752754296894559, 0.3333333333333333703, 0.3219752754296894559, 0.3333333333333333703, 0.3219752754296894559, 0.3333333333333333703, 0.3219752754296894559, 0.3333333333333333703, 0.3219752754296894559, 0.3333333333333333703, 0.3219752754296894559, 0.3333333333333333703, 0.3219752754296894559, 0.3333333333333333703, 0.3219752754296894559, 0.3333333333333333703, 0.3219752754296894559, 0.3333333333333333703, 0.3219752754296894559, 0.3333333333333333703, 0.3219752754296894559, 0.3333333333333333703, 0.3219752754296894559, 0.3333333333333333703, 0.3219752754296894559, 0.3333333333333333703, 0.3219752754296894559, 0.3333333333333333703, 0.3219752754296894559, 0.3333333333333333703, 0.3219752754296894559, 0.3333333333333333703, 0.3219752754296894559, 0.3333333333333333703, 0.3219752754296894559, 0.3333333333333333703, 0.3219752754296894559, 0.3333333333333333703, 0.3219752754296894559, 0.3333333333333333703),
 ( 1.000000000000000000, 0.9659258262890683122, 1.000000000000000000, 0.9659258262890683122, 1.000000000000000000, 0.9659258262890683122, 1.000000000000000000, 0.9659258262890683122, 1.000000000000000000, 0.9659258262890683122, 1.000000000000000000, 0.9659258262890683122, 1.000000000000000000, 0.9659258262890683122, 1.000000000000000000, 0.9659258262890683122, 1.000000000000000000, 0.9659258262890683122, 1.000000000000000000, 0.9659258262890683122, 1.000000000000000000, 0.9659258262890683122, 1.000000000000000000, 0.9659258262890683122, 1.000000000000000000, 0.9659258262890683122, 1.000000000000000000, 0.9659258262890683122, 1.000000000000000000, 0.9659258262890683122, 1.000000000000000000, 0.9659258262890683122, 1.000000000000000000, 0.9659258262890683122, 1.000000000000000000, 0.9659258262890683122, 1.000000000000000000, 0.9659258262890683122, 1.000000000000000000, 0.9659258262890683122, 1.000000000000000000, 0.9659258262890683122, 1.000000000000000000, 0.9659258262890683122, 1.000000000000000000, 0.9659258262890683122, 1.000000000000000000, 0.9659258262890683122, 1.000000000000000000, 0.9659258262890683122, 1.000000000000000000, 0.9659258262890683122, 1.000000000000000000, 0.9659258262890683122, 1.000000000000000000, 0.9659258262890683122, 1.000000000000000000, 0.9659258262890683122, 1.000000000000000000, 0.9659258262890683122, 1.000000000000000000, 0.9659258262890683122, 1.000000000000000000, 0.9659258262890683122, 1.000000000000000000, 0.9659258262890683122, 1.000000000000000000, 0.9659258262890683122, 1.000000000000000000, 0.9659258262890683122, 1.000000000000000000, 0.9659258262890683122, 1.000000000000000000, 0.9659258262890683122, 1.000000000000000000, 0.9659258262890683122, 1.000000000000000000, 0.9659258262890683122, 1.000000000000000000, 0.9659258262890683122, 1.000000000000000000, 0.9659258262890683122, 1.000000000000000000, 0.9659258262890683122, 1.000000000000000000, 0.9659258262890683122, 1.000000000000000000, 0.9659258262890683122, 1.000000000000000000, 0.9659258262890683122, 1.000000000000000000, 0.9659258262890683122, 1.000000000000000000, 0.9659258262890683122, 1.000000000000000000, 0.9659258262890683122, 1.000000000000000000, 0.9659258262890683122, 1.000000000000000000, 0.9659258262890683122, 1.000000000000000000, 0.9659258262890683122, 1.000000000000000000, 0.9659258262890683122, 1.000000000000000000, 0.9659258262890683122, 1.000000000000000000, 0.9659258262890683122, 1.000000000000000000, 0.9659258262890683122, 1.000000000000000000, 0.9659258262890683122, 1.000000000000000000, 0.9659258262890683122, 1.000000000000000000, 0.9659258262890683122, 1.000000000000000000, 0.9659258262890683122, 1.000000000000000000, 0.9659258262890683122, 1.000000000000000000, 0.9659258262890683122, 1.000000000000000000, 0.9659258262890683122, 1.000000000000000000, 0.9659258262890683122, 1.000000000000000000, 0.9659258262890683122, 1.000000000000000000, 0.9659258262890683122, 1.000000000000000000, 0.9659258262890683122, 1.000000000000000000, 0.9659258262890683122, 1.000000000000000000, 0.9659258262890683122, 1.000000000000000000, 0.9659258262890683122, 1.000000000000000000, 0.9659258262890683122, 1.000000000000000000, 0.9659258262890683122, 1.000000000000000000, 0.9659258262890683122, 1.000000000000000000, 0.9659258262890683122, 1.000000000000000000, 0.9659258262890683122, 1.000000000000000000, 0.9659258262890683122, 1.000000000000000000, 0.9659258262890683122, 1.000000000000000000, 0.9659258262890683122, 1.000000000000000000, 0.9659258262890683122, 1.000000000000000000, 0.9659258262890683122, 1.000000000000000000, 0.9659258262890683122, 1.000000000000000000, 0.9659258262890683122, 1.000000000000000000, 0.9659258262890683122, 1.000000000000000000, 0.9659258262890683122, 1.000000000000000000, 0.9659258262890683122, 1.000000000000000000, 0.9659258262890683122, 1.000000000000000000, 0.9659258262890683122, 1.000000000000000000, 0.9659258262890683122, 1.000000000000000000, 0.9659258262890683122, 1.000000000000000000, 0.9659258262890683122, 1.000000000000000000, 0.9659258262890683122, 1.000000000000000000, 0.9659258262890683122, 1.000000000000000000, 0.9659258262890683122, 1.000000000000000000, 0.9659258262890683122, 1.000000000000000000, 0.9659258262890683122, 1.000000000000000000, 0.9659258262890683122, 1.000000000000000000, 0.9659258262890683122, 1.000000000000000000),
 ( 0.3333333333333333703, 0.3219752754296894559, 0.3333333333333333703, 0.3219752754296894559, 0.3333333333333333703, 0.3219752754296894559, 0.3333333333333333703, 0.3219752754296894559, 0.3333333333333333703, 0.3219752754296894559, 0.3333333333333333703, 0.3219752754296894559, 0.3333333333333333703, 0.3219752754296894559, 0.3333333333333333703, 0.3219752754296894559, 0.3333333333333333703, 0.3219752754296894559, 0.3333333333333333703, 0.3219752754296894559, 0.3333333333333333703, 0.3219752754296894559, 0.3333333333333333703, 0.3219752754296894559, 0.3333333333333333703, 0.3219752754296894559, 0.3333333333333333703, 0.3219752754296894559, 0.3333333333333333703, 0.3219752754296894559, 0.3333333333333333703, 0.3219752754296894559, 0.3333333333333333703, 0.3219752754296894559, 0.3333333333333333703, 0.3219752754296894559, 0.3333333333333333703, 0.3219752754296894559, 0.3333333333333333703, 0.3219752754296894559, 0.3333333333333333703, 0.3219752754296894559, 0.3333333333333333703, 0.3219752754296894559, 0.3333333333333333703, 0.3219752754296894559, 0.3333333333333333703, 0.3219752754296894559, 0.3333333333333333703, 0.3219752754296894559, 0.3333333333333333703, 0.3219752754296894559, 0.3333333333333333703, 0.3219752754296894559, 0.3333333333333333703, 0.3219752754296894559, 0.3333333333333333703, 0.3219752754296894559, 0.3333333333333333703, 0.3219752754296894559, 0.3333333333333333703, 0.3219752754296894559, 0.3333333333333333703, 0.3219752754296894559, 0.3333333333333333703, 0.3219752754296894559, 0.3333333333333333703, 0.3219752754296894559, 0.3333333333333333703, 0.3219752754296894559, 0.3333333333333333703, 0.3219752754296894559, 0.3333333333333333703, 0.3219752754296894559, 0.3333333333333333703, 0.3219752754296894559, 0.3333333333333333703, 0.3219752754296894559, 0.3333333333333333703, 0.3219752754296894559, 0.3333333333333333703, 0.3219752754296894559, 0.3333333333333333703, 0.3219752754296894559, 0.3333333333333333703, 0.3219752754296894559, 0.3333333333333333703, 0.3219752754296894559, 0.3333333333333333703, 0.3219752754296894559, 0.3333333333333333703, 0.3219752754296894559, 0.3333333333333333703, 0.3219752754296894559, 0.3333333333333333703, 0.3219752754296894559, 0.3333333333333333703, 0.3219752754296894559, 0.3333333333333333703, 0.3219752754296894559, 0.3333333333333333703, 0.3219752754296894559, 0.3333333333333333703, 0.3219752754296894559, 0.3333333333333333703, 0.3219752754296894559, 0.3333333333333333703, 0.3219752754296894559, 0.3333333333333333703, 0.3219752754296894559, 0.3333333333333333703, 0.3219752754296894559, 0.3333333333333333703, 0.3219752754296894559, 0.3333333333333333703, 0.3219752754296894559, 0.3333333333333333703, 0.3219752754296894559, 0.3333333333333333703, 0.3219752754296894559, 0.3333333333333333703, 0.3219752754296894559, 0.3333333333333333703, 0.3219752754296894559, 0.3333333333333333703, 0.3219752754296894559, 0.3333333333333333703, 0.3219752754296894559, 0.3333333333333333703, 0.3219752754296894559, 0.3333333333333333703, 0.3219752754296894559, 0.3333333333333333703, 0.3219752754296894559, 0.3333333333333333703, 0.3219752754296894559, 0.3333333333333333703, 0.3219752754296894559, 0.3333333333333333703, 0.3219752754296894559, 0.3333333333333333703, 0.3219752754296894559, 0.3333333333333333703, 0.3219752754296894559, 0.3333333333333333703, 0.3219752754296894559, 0.3333333333333333703, 0.3219752754296894559, 0.3333333333333333703, 0.3219752754296894559, 0.3333333333333333703, 0.3219752754296894559, 0.3333333333333333703, 0.3219752754296894559, 0.3333333333333333703, 0.3219752754296894559, 0.3333333333333333703, 0.3219752754296894559, 0.3333333333333333703, 0.3219752754296894559, 0.3333333333333333703, 0.3219752754296894559, 0.3333333333333333703, 0.3219752754296894559, 0.3333333333333333703, 0.3219752754296894559, 0.3333333333333333703, 0.3219752754296894559, 0.3333333333333333703, 0.3219752754296894559, 0.3333333333333333703, 0.3219752754296894559, 0.3333333333333333703, 0.3219752754296894559, 0.3333333333333333703, 0.3219752754296894559, 0.3333333333333333703, 0.3219752754296894559, 0.3333333333333333703, 0.3219752754296894559, 0.3333333333333333703, 0.3219752754296894559, 0.3333333333333333703, 0.3219752754296894559, 0.3333333333333333703, 0.3219752754296894559, 0.3333333333333333703, 0.3219752754296894559, 0.3333333333333333703, 0.3219752754296894559, 0.3333333333333333703, 0.3219752754296894559, 0.3333333333333333703),
 ( 0.3333333333333333703, 0.3219752754296894559, 0.3333333333333333703, 0.3219752754296894559, 0.3333333333333333703, 0.3219752754296894559, 0.3333333333333333703, 0.3219752754296894559, 0.3333333333333333703, 0.3219752754296894559, 0.3333333333333333703, 0.3219752754296894559, 0.3333333333333333703, 0.3219752754296894559, 0.3333333333333333703, 0.3219752754296894559, 0.3333333333333333703, 0.3219752754296894559, 0.3333333333333333703, 0.3219752754296894559, 0.3333333333333333703, 0.3219752754296894559, 0.3333333333333333703, 0.3219752754296894559, 0.3333333333333333703, 0.3219752754296894559, 0.3333333333333333703, 0.3219752754296894559, 0.3333333333333333703, 0.3219752754296894559, 0.3333333333333333703, 0.3219752754296894559, 0.3333333333333333703, 0.3219752754296894559, 0.3333333333333333703, 0.3219752754296894559, 0.3333333333333333703, 0.3219752754296894559, 0.3333333333333333703, 0.3219752754296894559, 0.3333333333333333703, 0.3219752754296894559, 0.3333333333333333703, 0.3219752754296894559, 0.3333333333333333703, 0.3219752754296894559, 0.3333333333333333703, 0.3219752754296894559, 0.3333333333333333703, 0.3219752754296894559, 0.3333333333333333703, 0.3219752754296894559, 0.3333333333333333703, 0.3219752754296894559, 0.3333333333333333703, 0.3219752754296894559, 0.3333333333333333703, 0.3219752754296894559, 0.3333333333333333703, 0.3219752754296894559, 0.3333333333333333703, 0.3219752754296894559, 0.3333333333333333703, 0.3219752754296894559, 0.3333333333333333703, 0.3219752754296894559, 0.3333333333333333703, 0.3219752754296894559, 0.3333333333333333703, 0.3219752754296894559, 0.3333333333333333703, 0.3219752754296894559, 0.3333333333333333703, 0.3219752754296894559, 0.3333333333333333703, 0.3219752754296894559, 0.3333333333333333703, 0.3219752754296894559, 0.3333333333333333703, 0.3219752754296894559, 0.3333333333333333703, 0.3219752754296894559, 0.3333333333333333703, 0.3219752754296894559, 0.3333333333333333703, 0.3219752754296894559, 0.3333333333333333703, 0.3219752754296894559, 0.3333333333333333703, 0.3219752754296894559, 0.3333333333333333703, 0.3219752754296894559, 0.3333333333333333703, 0.3219752754296894559, 0.3333333333333333703, 0.3219752754296894559, 0.3333333333333333703, 0.3219752754296894559, 0.3333333333333333703, 0.3219752754296894559, 0.3333333333333333703, 0.3219752754296894559, 0.3333333333333333703, 0.3219752754296894559, 0.3333333333333333703, 0.3219752754296894559, 0.3333333333333333703, 0.3219752754296894559, 0.3333333333333333703, 0.3219752754296894559, 0.3333333333333333703, 0.3219752754296894559, 0.3333333333333333703, 0.3219752754296894559, 0.3333333333333333703, 0.3219752754296894559, 0.3333333333333333703, 0.3219752754296894559, 0.3333333333333333703, 0.3219752754296894559, 0.3333333333333333703, 0.3219752754296894559, 0.3333333333333333703, 0.3219752754296894559, 0.3333333333333333703, 0.3219752754296894559, 0.3333333333333333703, 0.3219752754296894559, 0.3333333333333333703, 0.3219752754296894559, 0.3333333333333333703, 0.3219752754296894559, 0.3333333333333333703, 0.3219752754296894559, 0.3333333333333333703, 0.3219752754296894559, 0.3333333333333333703, 0.3219752754296894559, 0.3333333333333333703, 0.3219752754296894559, 0.3333333333333333703, 0.3219752754296894559, 0.3333333333333333703, 0.3219752754296894559, 0.3333333333333333703, 0.3219752754296894559, 0.3333333333333333703, 0.3219752754296894559, 0.3333333333333333703, 0.3219752754296894559, 0.3333333333333333703, 0.3219752754296894559, 0.3333333333333333703, 0.3219752754296894559, 0.3333333333333333703, 0.3219752754296894559, 0.3333333333333333703, 0.3219752754296894559, 0.3333333333333333703, 0.3219752754296894559, 0.3333333333333333703, 0.3219752754296894559, 0.3333333333333333703, 0.3219752754296894559, 0.3333333333333333703, 0.3219752754296894559, 0.3333333333333333703, 0.3219752754296894559, 0.3333333333333333703, 0.3219752754296894559, 0.3333333333333333703, 0.3219752754296894559, 0.3333333333333333703, 0.3219752754296894559, 0.3333333333333333703, 0.3219752754296894559, 0.3333333333333333703, 0.3219752754296894559, 0.3333333333333333703, 0.3219752754296894559, 0.3333333333333333703, 0.3219752754296894559, 0.3333333333333333703, 0.3219752754296894559, 0.3333333333333333703, 0.3219752754296894559, 0.3333333333333333703, 0.3219752754296894559, 0.3333333333333333703, 0.3219752754296894559, 0.3333333333333333703, 0.3219752754296894559, 0.3333333333333333703),
 ( 1.000000000000000000, 0.9659258262890683122, 1.000000000000000000, 0.9659258262890683122, 1.000000000000000000, 0.9659258262890683122, 1.000000000000000000, 0.9659258262890683122, 1.000000000000000000, 0.9659258262890683122, 1.000000000000000000, 0.9659258262890683122, 1.000000000000000000, 0.9659258262890683122, 1.000000000000000000, 0.9659258262890683122, 1.000000000000000000, 0.9659258262890683122, 1.000000000000000000, 0.9659258262890683122, 1.000000000000000000, 0.9659258262890683122, 1.000000000000000000, 0.9659258262890683122, 1.000000000000000000, 0.9659258262890683122, 1.000000000000000000, 0.9659258262890683122, 1.000000000000000000, 0.9659258262890683122, 1.000000000000000000, 0.9659258262890683122, 1.000000000000000000, 0.9659258262890683122, 1.000000000000000000, 0.9659258262890683122, 1.000000000000000000, 0.9659258262890683122, 1.000000000000000000, 0.9659258262890683122, 1.000000000000000000, 0.9659258262890683122, 1.000000000000000000, 0.9659258262890683122, 1.000000000000000000, 0.9659258262890683122, 1.000000000000000000, 0.9659258262890683122, 1.000000000000000000, 0.9659258262890683122, 1.000000000000000000, 0.9659258262890683122, 1.000000000000000000, 0.9659258262890683122, 1.000000000000000000, 0.9659258262890683122, 1.000000000000000000, 0.9659258262890683122, 1.000000000000000000, 0.9659258262890683122, 1.000000000000000000, 0.9659258262890683122, 1.000000000000000000, 0.9659258262890683122, 1.000000000000000000, 0.9659258262890683122, 1.000000000000000000, 0.9659258262890683122, 1.000000000000000000, 0.9659258262890683122, 1.000000000000000000, 0.9659258262890683122, 1.000000000000000000, 0.9659258262890683122, 1.000000000000000000, 0.9659258262890683122, 1.000000000000000000, 0.9659258262890683122, 1.000000000000000000, 0.9659258262890683122, 1.000000000000000000, 0.9659258262890683122, 1.000000000000000000, 0.9659258262890683122, 1.000000000000000000, 0.9659258262890683122, 1.000000000000000000, 0.9659258262890683122, 1.000000000000000000, 0.9659258262890683122, 1.000000000000000000, 0.9659258262890683122, 1.000000000000000000, 0.9659258262890683122, 1.000000000000000000, 0.9659258262890683122, 1.000000000000000000, 0.9659258262890683122, 1.000000000000000000, 0.9659258262890683122, 1.000000000000000000, 0.9659258262890683122, 1.000000000000000000, 0.9659258262890683122, 1.000000000000000000, 0.9659258262890683122, 1.000000000000000000, 0.9659258262890683122, 1.000000000000000000, 0.9659258262890683122, 1.000000000000000000, 0.9659258262890683122, 1.000000000000000000, 0.9659258262890683122, 1.000000000000000000, 0.9659258262890683122, 1.000000000000000000, 0.9659258262890683122, 1.000000000000000000, 0.9659258262890683122, 1.000000000000000000, 0.9659258262890683122, 1.000000000000000000, 0.9659258262890683122, 1.000000000000000000, 0.9659258262890683122, 1.000000000000000000, 0.9659258262890683122, 1.000000000000000000, 0.9659258262890683122, 1.000000000000000000, 0.9659258262890683122, 1.000000000000000000, 0.9659258262890683122, 1.000000000000000000, 0.9659258262890683122, 1.000000000000000000, 0.9659258262890683122, 1.000000000000000000, 0.9659258262890683122, 1.000000000000000000, 0.9659258262890683122, 1.000000000000000000, 0.9659258262890683122, 1.000000000000000000, 0.9659258262890683122, 1.000000000000000000, 0.9659258262890683122, 1.000000000000000000, 0.9659258262890683122, 1.000000000000000000, 0.9659258262890683122, 1.000000000000000000, 0.9659258262890683122, 1.000000000000000000, 0.9659258262890683122, 1.000000000000000000, 0.9659258262890683122, 1.000000000000000000, 0.9659258262890683122, 1.000000000000000000, 0.9659258262890683122, 1.000000000000000000, 0.9659258262890683122, 1.000000000000000000, 0.9659258262890683122, 1.000000000000000000, 0.9659258262890683122, 1.000000000000000000, 0.9659258262890683122, 1.000000000000000000, 0.9659258262890683122, 1.000000000000000000, 0.9659258262890683122, 1.000000000000000000, 0.9659258262890683122, 1.000000000000000000, 0.9659258262890683122, 1.000000000000000000, 0.9659258262890683122, 1.000000000000000000, 0.9659258262890683122, 1.000000000000000000, 0.9659258262890683122, 1.000000000000000000, 0.9659258262890683122, 1.000000000000000000, 0.9659258262890683122, 1.000000000000000000, 0.9659258262890683122, 1.000000000000000000, 0.9659258262890683122, 1.000000000000000000) ) ) 
 REPRESENTATION_ITEM ( '' )  SURFACE ( )  );
#17020=CARTESIAN_POINT ( 'NONE',  ( -10.58745947852649927, -21.64274437364853654, 20.88867750791695954 ) ) ;
#17022=CARTESIAN_POINT ( 'NONE',  ( -9.999999999999994671, -24.16482700510257686, 26.57617750791695954 ) ) ;
#17024=CARTESIAN_POINT ( 'NONE',  ( -19.41254052147350961, -21.64274437364857562, 26.36132249208304401 ) ) ;
#17033=CARTESIAN_POINT ( 'NONE',  ( -21.95583473709189803, -26.04047135212049469, 36.20507249208304046 ) ) ;
#17035=CARTESIAN_POINT ( 'NONE',  ( -14.83517299489735741, -28.99999999999998224, 8.861322492083040459 ) ) ;
#17036=CARTESIAN_POINT ( 'NONE',  ( -17.95583473709191580, -23.03132541760400898, 29.41992750791696665 ) ) ;
#17038=CARTESIAN_POINT ( 'NONE',  ( -8.044165262908093084, -21.95952864787946979, 17.83007249208304046 ) ) ;
#17052=CARTESIAN_POINT ( 'NONE',  ( -21.14459132904236327, -27.35725562635143149, 34.01367750791695244 ) ) ;
#17056=CARTESIAN_POINT ( 'NONE',  ( -14.83517299489736985, -26.99999999999998579, 35.11132249208304756 ) ) ;
#17057=CARTESIAN_POINT ( 'NONE',  ( -9.996306089212364299, -29.24501739517662813, 11.48242750791695777 ) ) ;
#17066=CARTESIAN_POINT ( 'NONE',  ( -13.64274437364856141, -26.68048971390460622, 27.45117750791696309 ) ) ;
#17082=CARTESIAN_POINT ( 'NONE',  ( -17.35725562635144215, -19.58745947852648683, 24.82617750791695954 ) ) ;
#17085=CARTESIAN_POINT ( 'NONE',  ( -18.78091578003892081, -20.46040770435013556, 26.58007249208304401 ) ) ;
#17087=CARTESIAN_POINT ( 'NONE',  ( -18.04416526290808775, -23.36097942780924441, 31.39257249208304401 ) ) ;
#17105=CARTESIAN_POINT ( 'NONE',  ( -13.82508104294698192, -29.04416526290806644, 32.91992750791695954 ) ) ;
#17107=CARTESIAN_POINT ( 'NONE',  ( -12.64274437364858628, -19.58745947852646552, 32.92382249208304046 ) ) ;
#17109=CARTESIAN_POINT ( 'NONE',  ( -16.50457296725820555, -28.95583473709189448, 17.60742750791695599 ) ) ;
#17112=CARTESIAN_POINT ( 'NONE',  ( -19.95583473709191225, -22.49542703274176603, 29.41992750791695599 ) ) ;
#17114=CARTESIAN_POINT ( 'NONE',  ( -16.50457296725825174, -19.04416526290807354, 27.01757249208304046 ) ) ;
#17123=CARTESIAN_POINT ( 'NONE',  ( -17.04047135212050890, -17.04416526290807710, 37.51757249208304046 ) ) ;
#17127=CARTESIAN_POINT ( 'NONE',  ( -16.35725562635142794, -21.31951028609535470, 35.32617750791695244 ) ) ;
#17129=CARTESIAN_POINT ( 'NONE',  ( -15.16482700510264436, -16.99999999999997868, 21.98632249208304046 ) ) ;
#17143=CARTESIAN_POINT ( 'NONE',  ( -20.97976432393977575, -20.35725562635143504, 24.38867750791695954 ) ) ;
#17148=CARTESIAN_POINT ( 'NONE',  ( -17.51566270880199738, -25.64274437364856496, 25.48632249208304401 ) ) ;
#17151=CARTESIAN_POINT ( 'NONE',  ( -14.83517299489740715, -16.99999999999997868, 14.76367750791695777 ) ) ;
#17156=CARTESIAN_POINT ( 'NONE',  ( -11.99999999999999289, -24.16482700510258752, 31.82617750791696309 ) ) ;
#17161=ORIENTED_EDGE ( 'NONE', *, *, #16077, .T. ) ;
#17174=CARTESIAN_POINT ( 'NONE',  ( -20.04416526290808065, -25.17491895705300209, 23.73242750791694888 ) ) ;
#17177=CARTESIAN_POINT ( 'NONE',  ( -19.95583473709190514, -25.50457296725822687, 25.70507249208304756 ) ) ;
#17180=CARTESIAN_POINT ( 'NONE',  ( -12.68318583509882380, -26.07549068051207541, 34.45507249208304046 ) ) ;
#17200=CARTESIAN_POINT ( 'NONE',  ( -11.46040770435012668, -27.78091578003887463, 32.48242750791695954 ) ) ;
#17202=CARTESIAN_POINT ( 'NONE',  ( -13.49542703274174116, -28.95583473709188738, 34.89257249208304046 ) ) ;
#17204=CARTESIAN_POINT ( 'NONE',  ( -19.99999999999999645, -23.83517299489738051, 23.95117750791695954 ) ) ;
#17207=CARTESIAN_POINT ( 'NONE',  ( -19.95583473709191225, -22.49542703274176603, 34.66992750791695244 ) ) ;
#17209=CARTESIAN_POINT ( 'NONE',  ( -10.04416526290808598, -22.49542703274172695, 28.33007249208304401 ) ) ;
#17210=ADVANCED_FACE ( 'NONE', ( #9031 ), #119, .F. ) ;
#17221=CARTESIAN_POINT ( 'NONE',  ( -15.16482700510260706, -26.99999999999998579, 27.88867750791696309 ) ) ;
#17223=CARTESIAN_POINT ( 'NONE',  ( -7.955834737091903364, -25.71081734191518464, 28.76757249208303691 ) ) ;
#17239=CARTESIAN_POINT ( 'NONE',  ( -18.35725562635144925, -17.85540867095761186, 35.32617750791695244 ) ) ;
#17243=CARTESIAN_POINT ( 'NONE',  ( -12.68318583509882380, -26.07549068051207541, 34.45507249208304046 ) ) ;
#17244=CARTESIAN_POINT ( 'NONE',  ( -18.35725562635144925, -17.85540867095761186, 30.07617750791695599 ) ) ;
#17249=CARTESIAN_POINT ( 'NONE',  ( -17.31681416490115311, -26.07549068051209318, 33.79492750791695954 ) ) ;
#17253=DIRECTION ( 'NONE',  ( 6.216479319370943891E-15, -1.000000000000000000, 0.000000000000000000 ) ) ;
#17263=DIRECTION ( 'NONE',  ( 0.1648270051026194671, 0.000000000000000000, -0.9863224920830413467 ) ) ;
#17267=CARTESIAN_POINT ( 'NONE',  ( -10.75228648362910100, -26.64274437364854009, 37.51367750791695954 ) ) ;
#17271=CARTESIAN_POINT ( 'NONE',  ( -18.53959229564982536, -27.78091578003890660, 35.76757249208302625 ) ) ;
#17274=CARTESIAN_POINT ( 'NONE',  ( -16.35725562635141372, -26.68048971390461332, 30.29882249208304401 ) ) ;
#17292=CARTESIAN_POINT ( 'NONE',  ( -15.16482700510259640, -28.99999999999998224, 27.88867750791695954 ) ) ;
#17294=CARTESIAN_POINT ( 'NONE',  ( -11.21908421996106320, -27.53959229564982181, 39.70507249208304046 ) ) ;
#17299=CARTESIAN_POINT ( 'NONE',  ( -9.955834737091912245, -22.82508104294696594, 31.60742750791695954 ) ) ;
#17302=CARTESIAN_POINT ( 'NONE',  ( -12.35725562635143682, -19.75228648362908501, 30.95117750791695954 ) ) ;
#17304=CARTESIAN_POINT ( 'NONE',  ( -12.64274437364858628, -19.58745947852646552, 22.42382249208304401 ) ) ;
#17313=CARTESIAN_POINT ( 'NONE',  ( -9.999999999999994671, -24.16482700510257686, 0.3261775079169582647 ) ) ;
#17315=CARTESIAN_POINT ( 'NONE',  ( -22.04416526290809486, -22.28918265808477628, 31.39257249208304401 ) ) ;
#17328=CARTESIAN_POINT ( 'NONE',  ( -13.28918265808472299, -31.04416526290805933, 38.16992750791695954 ) ) ;
#17333=CARTESIAN_POINT ( 'NONE',  ( -11.99999999999999289, -24.16482700510258752, 0.3261775079169599856 ) ) ;
#17334=CARTESIAN_POINT ( 'NONE',  ( -7.999999999999996447, -24.16482700510256976, 26.57617750791695954 ) ) ;
#17353=CARTESIAN_POINT ( 'NONE',  ( -21.95583473709191580, -21.95952864787954084, 3.169927507916957321 ) ) ;
#17356=COLOUR_RGB ( '', 0.31764706, 0.68627451, 0.89019608) ;
#17358=CARTESIAN_POINT ( 'NONE',  ( -11.21908421996106320, -27.53959229564982181, 29.20507249208303335 ) ) ;
#17361=CARTESIAN_POINT ( 'NONE',  ( -12.92450931948790149, -21.68318583509881137, 33.14257249208304756 ) ) ;
#17369=CARTESIAN_POINT ( 'NONE',  ( -15.16482700510259640, -28.99999999999998224, 33.13867750791696665 ) ) ;
#17376=CARTESIAN_POINT ( 'NONE',  ( -14.83517299489739649, -18.99999999999997868, 25.26367750791695599 ) ) ;
#17381=CARTESIAN_POINT ( 'NONE',  ( -13.49542703274174116, -28.95583473709188738, 29.64257249208303691 ) ) ;
#17384=CARTESIAN_POINT ( 'NONE',  ( -12.35725562635143682, -19.75228648362908501, 25.70117750791695599 ) ) ;
#17387=CARTESIAN_POINT ( 'NONE',  ( -10.75228648362910100, -26.64274437364854009, 27.01367750791695954 ) ) ;
#17402=CARTESIAN_POINT ( 'NONE',  ( -19.95583473709191580, -22.49542703274176603, 3.169927507916957321 ) ) ;
#17404=CARTESIAN_POINT ( 'NONE',  ( -17.04047135212050890, -17.04416526290807710, 27.01757249208303691 ) ) ;
#17422=CARTESIAN_POINT ( 'NONE',  ( -8.855408670957602979, -27.35725562635137820, 2.736322492083039126 ) ) ;
#17425=EDGE_LOOP ( 'NONE', ( #8027, #6467, #11973 ) ) ;
#17426=CARTESIAN_POINT ( 'NONE',  ( -17.31681416490115311, -26.07549068051209318, 7.544927507916959541 ) ) ;
#17428=CARTESIAN_POINT ( 'NONE',  ( -20.00369391078762860, -18.75498260482333279, 35.10742750791695244 ) ) ;
#17447=CARTESIAN_POINT ( 'NONE',  ( -19.99999999999999645, -23.83517299489738051, 39.70117750791695954 ) ) ;
#17450=CARTESIAN_POINT ( 'NONE',  ( -15.63902057219073605, -27.04416526290807710, 9.080072492083042235 ) ) ;
#17454=CARTESIAN_POINT ( 'NONE',  ( -12.48433729119799196, -22.35725562635139596, 38.61132249208304046 ) ) ;
#17462=CARTESIAN_POINT ( 'NONE',  ( -10.58745947852649927, -21.64274437364853654, 31.38867750791696309 ) ) ;
#17466=UNCERTAINTY_MEASURE_WITH_UNIT (LENGTH_MEASURE( 1.000000000000000082E-05 ), #7519, 'distance_accuracy_value', 'NONE');
#17467=CARTESIAN_POINT ( 'NONE',  ( -11.21908421996106320, -27.53959229564982181, 8.205072492083036906 ) ) ;
#17468=CARTESIAN_POINT ( 'NONE',  ( -11.64274437364854187, -30.14459132904234195, 6.451177507916957765 ) ) ;
#17470=CARTESIAN_POINT ( 'NONE',  ( -10.75228648362912232, -21.35725562635138530, 33.36132249208304046 ) ) ;
#17475=CARTESIAN_POINT ( 'NONE',  ( -11.46040770435012668, -27.78091578003887463, 27.23242750791694888 ) ) ;
#17479=CARTESIAN_POINT ( 'NONE',  ( -9.955834737091903364, -25.17491895705295235, 39.26757249208304046 ) ) ;
#17491=CARTESIAN_POINT ( 'NONE',  ( -17.64274437364855430, -28.24771351637087236, 7.326177507916957765 ) ) ;
#17494=CARTESIAN_POINT ( 'NONE',  ( -11.64274437364859693, -17.85540867095757989, 38.17382249208303335 ) ) ;
#17497=CARTESIAN_POINT ( 'NONE',  ( -18.78091578003889595, -27.53959229564985023, 7.544927507916957765 ) ) ;
#17511=CARTESIAN_POINT ( 'NONE',  ( -18.35725562635138886, -30.14459132904237393, 4.048822492083038682 ) ) ;
#17517=CARTESIAN_POINT ( 'NONE',  ( -12.04416526290807887, -24.96867458239596260, 5.794927507916960430 ) ) ;
#17518=CARTESIAN_POINT ( 'NONE',  ( -20.24501739517664234, -29.00369391078761439, 33.79492750791695244 ) ) ;
#17544=CARTESIAN_POINT ( 'NONE',  ( -11.35725562635144925, -18.02023567606020293, -0.5488224920830435671 ) ) ;
#17548=CARTESIAN_POINT ( 'NONE',  ( -11.21908421996106320, -27.53959229564982181, 39.70507249208304046 ) ) ;
#17553=CARTESIAN_POINT ( 'NONE',  ( -13.35725562635141195, -26.51566270880198672, 39.92382249208304756 ) ) ;
#17567=CARTESIAN_POINT ( 'NONE',  ( -18.53959229564986799, -20.21908421996107563, 29.85742750791695599 ) ) ;
#17570=CARTESIAN_POINT ( 'NONE',  ( -11.21908421996108629, -20.46040770435011069, 4.919927507916955989 ) ) ;
#17574=CARTESIAN_POINT ( 'NONE',  ( -19.99999999999999645, -24.16482700510261949, 10.17382249208304046 ) ) ;
#17576=CARTESIAN_POINT ( 'NONE',  ( -20.24501739517664234, -29.00369391078761439, 2.294927507916956433 ) ) ;
#17579=CARTESIAN_POINT ( 'NONE',  ( -17.95583473709190869, -24.96867458239598037, 4.705072492083043123 ) ) ;
#17584=CARTESIAN_POINT ( 'NONE',  ( -9.999999999999994671, -24.16482700510257686, 31.82617750791696309 ) ) ;
#17588=CARTESIAN_POINT ( 'NONE',  ( -17.64274437364858983, -19.75228648362910633, 37.29882249208303335 ) ) ;
#17597=CARTESIAN_POINT ( 'NONE',  ( -12.35725562635143682, -19.75228648362908501, 9.951177507916959541 ) ) ;
#17598=CARTESIAN_POINT ( 'NONE',  ( -19.99999999999999645, -23.83517299489738051, 8.201177507916957765 ) ) ;
#17600=CARTESIAN_POINT ( 'NONE',  ( -18.35725562635138886, -30.14459132904237393, 35.54882249208304046 ) ) ;
#17602=CARTESIAN_POINT ( 'NONE',  ( -14.83517299489738761, -20.99999999999997513, 35.76367750791695954 ) ) ;
#17613=CARTESIAN_POINT ( 'NONE',  ( -21.95583473709191580, -21.95952864787954084, 39.91992750791695954 ) ) ;
#17618=CARTESIAN_POINT ( 'NONE',  ( -16.64274437364858272, -21.48433729119797420, 42.54882249208304756 ) ) ;
#17619=CARTESIAN_POINT ( 'NONE',  ( -17.04047135212043784, -30.95583473709190159, 33.35742750791695244 ) ) ;
#17640=CARTESIAN_POINT ( 'NONE',  ( -9.754982604823348780, -18.99630608921234654, 4.919927507916955989 ) ) ;
#17645=CARTESIAN_POINT ( 'NONE',  ( -18.04416526290808775, -23.36097942780924441, 5.142572492083044011 ) ) ;
#17650=CARTESIAN_POINT ( 'NONE',  ( -11.95583473709191047, -23.36097942780921954, 5.357427507916959541 ) ) ;
#17651=DIRECTION ( 'NONE',  ( 0.9863224920830413467, 5.275954983314436132E-15, 0.1648270051026190230 ) ) ;
#17660=CARTESIAN_POINT ( 'NONE',  ( -18.78091578003889950, -27.53959229564985378, 23.29492750791695954 ) ) ;
#17663=CARTESIAN_POINT ( 'NONE',  ( -18.78091578003889950, -27.53959229564985378, 2.294927507916958209 ) ) ;
#17667=CARTESIAN_POINT ( 'NONE',  ( -7.955834737091903364, -25.71081734191518464, 39.26757249208304756 ) ) ;
#17668=CARTESIAN_POINT ( 'NONE',  ( -18.64274437364853654, -29.97976432393976509, 7.326177507916955989 ) ) ;
#17671=CARTESIAN_POINT ( 'NONE',  ( -19.41254052147350961, -21.64274437364857562, 42.11132249208304046 ) ) ;
#17680=CARTESIAN_POINT ( 'NONE',  ( -18.53959229564983247, -27.78091578003891016, 35.76757249208303335 ) ) ;
#17692=CARTESIAN_POINT ( 'NONE',  ( -18.53959229564986799, -20.21908421996107563, 3.607427507916956877 ) ) ;
#17694=CARTESIAN_POINT ( 'NONE',  ( -15.16482700510263371, -18.99999999999997868, 11.48632249208304046 ) ) ;
#17696=CARTESIAN_POINT ( 'NONE',  ( -9.955834737091912245, -22.82508104294696594, 0.1074275079169582509 ) ) ;
#17710=CARTESIAN_POINT ( 'NONE',  ( -20.97976432393977575, -20.35725562635143504, 40.13867750791695954 ) ) ;
#17712=PRESENTATION_STYLE_ASSIGNMENT (( #1444 ) ) ;
#17714=CARTESIAN_POINT ( 'NONE',  ( -14.83517299489735741, -28.99999999999998224, 3.611322492083041347 ) ) ;
#17718=CARTESIAN_POINT ( 'NONE',  ( -11.95583473709191047, -23.36097942780921954, 0.1074275079169599995 ) ) ;
#17719=CARTESIAN_POINT ( 'NONE',  ( -11.64274437364859693, -17.85540867095757989, 11.92382249208304046 ) ) ;
#17740=CARTESIAN_POINT ( 'NONE',  ( -8.855408670957631401, -20.64274437364852943, 5.138677507916955989 ) ) ;
#17745=CARTESIAN_POINT ( 'NONE',  ( -15.16482700510262482, -20.99999999999997513, 6.236322492083043123 ) ) ;
#17752=CARTESIAN_POINT ( 'NONE',  ( -12.92450931948788906, -26.31681416490114245, 0.9824275079169599856 ) ) ;
#17763=CARTESIAN_POINT ( 'NONE',  ( -14.83517299489739649, -18.99999999999997868, 30.51367750791695954 ) ) ;
#17765=CARTESIAN_POINT ( 'NONE',  ( -19.99999999999999645, -23.83517299489738051, 8.201177507916957765 ) ) ;
#17768=CARTESIAN_POINT ( 'NONE',  ( -13.82508104294702100, -18.95583473709188382, 1.205072492083041125 ) ) ;
#17769=CARTESIAN_POINT ( 'NONE',  ( -18.53959229564986799, -20.21908421996107563, 40.35742750791696665 ) ) ;
#17771=CARTESIAN_POINT ( 'NONE',  ( -15.16482700510263371, -18.99999999999997868, 42.98632249208304046 ) ) ;
#17793=CARTESIAN_POINT ( 'NONE',  ( -10.04416526290807710, -25.50457296725819489, 5.794927507916955989 ) ) ;
#17794=CARTESIAN_POINT ( 'NONE',  ( -10.75228648362910100, -26.64274437364854009, 11.26367750791695777 ) ) ;
#17796=CARTESIAN_POINT ( 'NONE',  ( -9.955834737091903364, -25.17491895705294880, 2.517572492083040903 ) ) ;
#17799=CARTESIAN_POINT ( 'NONE',  ( -12.64274437364855252, -28.41254052147347053, 6.451177507916959541 ) ) ;
#17801=CARTESIAN_POINT ( 'NONE',  ( -10.58745947852649927, -21.64274437364853654, 10.38867750791695777 ) ) ;
#17812=CARTESIAN_POINT ( 'NONE',  ( -9.020235676060250896, -20.35725562635137820, 22.86132249208304046 ) ) ;
#17817=CARTESIAN_POINT ( 'NONE',  ( -12.68318583509884157, -21.92450931948787485, 20.66992750791696665 ) ) ;
#17819=CARTESIAN_POINT ( 'NONE',  ( -20.24501739517669563, -18.99630608921239627, 5.580072492083037794 ) ) ;
#17829=CARTESIAN_POINT ( 'NONE',  ( -12.07460121177581236, -20.93486186128575000, -1.847635612033976164E-16 ) ) ;
#17841=CARTESIAN_POINT ( 'NONE',  ( -21.99999999999999289, -23.83517299489739116, 13.45117750791695777 ) ) ;
#17846=CARTESIAN_POINT ( 'NONE',  ( -15.96867458239599635, -21.04416526290806999, 6.017572492083043123 ) ) ;
#17853=CARTESIAN_POINT ( 'NONE',  ( -17.31681416490115311, -26.07549068051209318, 7.544927507916959541 ) ) ;
#17865=CARTESIAN_POINT ( 'NONE',  ( -15.16482700510259640, -28.99999999999998224, 38.38867750791695954 ) ) ;
#17867=CARTESIAN_POINT ( 'NONE',  ( -19.95583473709191580, -22.49542703274176603, 8.419927507916955989 ) ) ;
#17871=CARTESIAN_POINT ( 'NONE',  ( -12.64274437364858628, -19.58745947852646552, 6.673822492083040459 ) ) ;
#17875=CARTESIAN_POINT ( 'NONE',  ( -13.35725562635141195, -26.51566270880198672, 8.423822492083042235 ) ) ;
#17897=CARTESIAN_POINT ( 'NONE',  ( -12.64274437364855252, -28.41254052147347053, 1.201177507916958431 ) ) ;
#17899=CARTESIAN_POINT ( 'NONE',  ( -10.04416526290807710, -25.50457296725819489, 16.29492750791695954 ) ) ;
#17902=CARTESIAN_POINT ( 'NONE',  ( -11.21908421996106320, -27.53959229564982181, 2.955072492083040903 ) ) ;
#17904=CARTESIAN_POINT ( 'NONE',  ( -16.17491895705301275, -18.95583473709189803, 9.294927507916954212 ) ) ;
#17906=CARTESIAN_POINT ( 'NONE',  ( -9.967509313853890163, -23.17922740248042857, 0.1652515419773398775 ) ) ;
#17918=CARTESIAN_POINT ( 'NONE',  ( -17.04047135212050890, -17.04416526290807710, 16.51757249208304046 ) ) ;
#17923=CARTESIAN_POINT ( 'NONE',  ( -13.64274437364856141, -26.68048971390460622, 22.20117750791696309 ) ) ;
#17925=CARTESIAN_POINT ( 'NONE',  ( -9.996306089212408708, -18.75498260482328661, 12.14257249208303691 ) ) ;
#17943=CARTESIAN_POINT ( 'NONE',  ( -17.04047135212043784, -30.95583473709190159, 22.85742750791695599 ) ) ;
#17947=CARTESIAN_POINT ( 'NONE',  ( -15.96867458239599635, -21.04416526290806999, 21.76757249208304756 ) ) ;
#17952=CARTESIAN_POINT ( 'NONE',  ( -12.31951028609537602, -22.64274437364854364, 5.138677507916959541 ) ) ;
#17965=CARTESIAN_POINT ( 'NONE',  ( -19.41254052147348830, -26.35725562635142083, 13.01367750791695777 ) ) ;
#17968=CARTESIAN_POINT ( 'NONE',  ( -10.04416526290808953, -22.49542703274172695, 12.58007249208304046 ) ) ;
#17970=CARTESIAN_POINT ( 'NONE',  ( -12.31951028609536536, -25.35725562635139596, 7.986322492083044011 ) ) ;
#17980=CARTESIAN_POINT ( 'NONE',  ( -11.21337592062047328, -21.65370470877428133, 1.651559915991179248E-16 ) ) ;
#17982=FILL_AREA_STYLE_COLOUR ( '', #17356 ) ;
#17992=CARTESIAN_POINT ( 'NONE',  ( -19.95583473709191580, -22.49542703274176603, 8.419927507916955989 ) ) ;
#17995=CARTESIAN_POINT ( 'NONE',  ( -19.41254052147350961, -21.64274437364857562, 5.361322492083041347 ) ) ;
#17997=CARTESIAN_POINT ( 'NONE',  ( -17.07549068051210739, -21.68318583509881847, 40.35742750791696665 ) ) ;
#18000=CARTESIAN_POINT ( 'NONE',  ( -20.04416526290808065, -25.17491895705300209, 13.23242750791695777 ) ) ;
#18013=CARTESIAN_POINT ( 'NONE',  ( -7.955834737091903364, -25.71081734191518464, 18.26757249208304046 ) ) ;
#18018=CARTESIAN_POINT ( 'NONE',  ( -14.03132541760401786, -21.04416526290806289, 9.732427507916959541 ) ) ;
#18020=CARTESIAN_POINT ( 'NONE',  ( -20.00369391078762860, -18.75498260482333279, 40.35742750791695954 ) ) ;
#18043=CARTESIAN_POINT ( 'NONE',  ( -14.83517299489740715, -16.99999999999997868, 20.01367750791695954 ) ) ;
#18045=DIRECTION ( 'NONE',  ( -0.1648270051026182181, 0.000000000000000000, 0.9863224920830415687 ) ) ;
#18048=CARTESIAN_POINT ( 'NONE',  ( -17.95583473709190869, -24.96867458239598037, 20.45507249208304401 ) ) ;
#18052=CARTESIAN_POINT ( 'NONE',  ( -12.31951028609537602, -22.64274437364854364, 20.88867750791696309 ) ) ;
#18060=CARTESIAN_POINT ( 'NONE',  ( -10.31147837279037738, -22.25502639194775512, -4.119453415160654225E-17 ) ) ;
#18064=CARTESIAN_POINT ( 'NONE',  ( -19.99999999999999645, -23.83517299489738051, 39.70117750791695954 ) ) ;
#18066=CARTESIAN_POINT ( 'NONE',  ( -13.49542703274178379, -19.04416526290806289, 9.732427507916959541 ) ) ;
#18071=CARTESIAN_POINT ( 'NONE',  ( -20.04416526290809131, -22.82508104294699791, 15.64257249208304223 ) ) ;
#18074=CARTESIAN_POINT ( 'NONE',  ( -14.03132541760400009, -26.95583473709189448, 24.39257249208304046 ) ) ;
#18080=CARTESIAN_POINT ( 'NONE',  ( -18.78091578003889950, -27.53959229564985378, 39.04492750791695954 ) ) ;
#18089=B_SPLINE_CURVE_WITH_KNOTS ( 'NONE', 3,
 ( #90, #4604, #2924, #3120, #7433, #10461, #9101, #17829, #16553, #17980, #14794, #4405, #15090, #13603, #1364, #5972, #10367, #16455 ),
 .UNSPECIFIED., .F., .F.,
 ( 4, 2, 2, 2, 2, 2, 2, 2, 4 ),
 ( 0.000000000000000000, 0.001329345720928956512, 0.001994018581393434877, 0.002658691441857913024, 0.003988037162786874090, 0.004652710023251353105, 0.004985046453483592613, 0.005151214668599710632, 0.005317382883715828651 ),
 .UNSPECIFIED. ) ;
#18090=CARTESIAN_POINT ( 'NONE',  ( -16.50457296725820555, -28.95583473709189448, 12.35742750791695954 ) ) ;
#18091=CARTESIAN_POINT ( 'NONE',  ( -10.75228648362910100, -26.64274437364854009, 16.51367750791695954 ) ) ;
#18093=CARTESIAN_POINT ( 'NONE',  ( -10.58745947852648328, -26.35725562635138530, 13.23632249208304046 ) ) ;
#18095=CARTESIAN_POINT ( 'NONE',  ( -15.16482700510259640, -28.99999999999998224, 1.638677507916958431 ) ) ;
#18097=CARTESIAN_POINT ( 'NONE',  ( -16.17491895705301275, -18.95583473709189448, 25.04492750791695599 ) ) ;
#18110=CARTESIAN_POINT ( 'NONE',  ( -21.99999999999999289, -24.16482700510262305, 15.42382249208304046 ) ) ;
#18113=CARTESIAN_POINT ( 'NONE',  ( -15.16482700510263371, -18.99999999999997868, 6.236322492083041347 ) ) ;
#18116=CARTESIAN_POINT ( 'NONE',  ( -12.48433729119798130, -25.64274437364855075, 11.26367750791696132 ) ) ;
#18118=CARTESIAN_POINT ( 'NONE',  ( -12.95952864787948755, -30.95583473709188382, 8.642572492083038682 ) ) ;
#18136=CARTESIAN_POINT ( 'NONE',  ( -11.35725562635144925, -18.02023567606020293, 9.951177507916955989 ) ) ;
#18141=CARTESIAN_POINT ( 'NONE',  ( -11.99999999999999289, -23.83517299489735564, 18.04882249208304046 ) ) ;
#18142=CARTESIAN_POINT ( 'NONE',  ( -9.020235676060220698, -27.64274437364852588, 6.013677507916956877 ) ) ;
#18149=CARTESIAN_POINT ( 'NONE',  ( -11.99999999999999289, -24.16482700510258752, 21.32617750791695954 ) ) ;
#18163=CARTESIAN_POINT ( 'NONE',  ( -9.955834737091912245, -22.82508104294696594, 36.85742750791696665 ) ) ;
#18166=CARTESIAN_POINT ( 'NONE',  ( -12.64274437364855252, -28.41254052147347053, 11.70117750791695777 ) ) ;
#18171=CARTESIAN_POINT ( 'NONE',  ( -12.35725562635140307, -28.24771351637085459, 18.92382249208304401 ) ) ;
#18174=CARTESIAN_POINT ( 'NONE',  ( -15.96867458239599635, -21.04416526290806999, 16.51757249208304046 ) ) ;
#18194=CARTESIAN_POINT ( 'NONE',  ( -18.78091578003889950, -27.53959229564985378, 23.29492750791695954 ) ) ;
#18196=CARTESIAN_POINT ( 'NONE',  ( -19.95583473709190514, -25.50457296725822687, 25.70507249208304756 ) ) ;
#18200=CARTESIAN_POINT ( 'NONE',  ( -13.49542703274178379, -19.04416526290806289, 20.23242750791696309 ) ) ;
#18202=CARTESIAN_POINT ( 'NONE',  ( -12.64274437364855252, -28.41254052147347053, 11.70117750791695777 ) ) ;
#18216=CARTESIAN_POINT ( 'NONE',  ( -8.855408670957602979, -27.35725562635137820, 13.23632249208303868 ) ) ;
#18217=CARTESIAN_POINT ( 'NONE',  ( -9.999999999999994671, -23.83517299489734143, 12.79882249208304046 ) ) ;
#18219=CARTESIAN_POINT ( 'NONE',  ( -11.99999999999999289, -24.16482700510258752, 10.82617750791695954 ) ) ;
#18221=CARTESIAN_POINT ( 'NONE',  ( -9.020235676060250896, -20.35725562635137820, 17.61132249208303335 ) ) ;
#18239=CARTESIAN_POINT ( 'NONE',  ( -22.04416526290807710, -25.71081734191525925, 18.48242750791695954 ) ) ;
#18244=CARTESIAN_POINT ( 'NONE',  ( -17.31681416490117087, -21.92450931948788551, 10.83007249208304223 ) ) ;
#18247=CARTESIAN_POINT ( 'NONE',  ( -7.999999999999996447, -24.16482700510256976, 16.07617750791695599 ) ) ;
#18252=CARTESIAN_POINT ( 'NONE',  ( -14.83517299489738761, -20.99999999999997513, 14.76367750791695954 ) ) ;
#18265=CARTESIAN_POINT ( 'NONE',  ( -12.64274437364855252, -28.41254052147347053, 37.95117750791695954 ) ) ;
#18270=CARTESIAN_POINT ( 'NONE',  ( -11.21908421996108629, -20.46040770435011069, 15.41992750791695954 ) ) ;
#18274=CARTESIAN_POINT ( 'NONE',  ( -15.16482700510263371, -18.99999999999997868, 16.73632249208304401 ) ) ;
#18275=CARTESIAN_POINT ( 'NONE',  ( -13.35725562635141195, -26.51566270880198672, 13.67382249208304401 ) ) ;
#18281=( BOUNDED_CURVE ( )  B_SPLINE_CURVE ( 2, ( #13195, #12019, #4492, #2715, #16537, #8687, #3006, #14671, #3105, #9086, #19189, #5756, #17714, #4292, #10249, #10743, #6447, #6250, #16740, #3308, #13687, #18314, #8110, #7724, #18113, #6355, #367, #9472, #14080, #7819, #15558, #264, #12318, #4882, #9184, #8018, #17035, #12216, #15458, #461, #13787, #12416, #10843, #3592, #9279, #15171, #13885, #6156, #16838, #3401, #9370, #4685, #15365, #2126, #18217, #3503, #4979, #18511, #1938, #10937, #1835, #10643, #18412, #7922, #16940, #12118, #2027, #13985, #555, #6542, #4794, #12509, #15266, #5078, #11036, #9563, #16646, #3211, #1739, #11022, #8099, #18401, #6810, #12775, #11117, #2208, #12685, #18771, #5344, #3866, #6530, #9648, #3581, #15739, #6434, #11306, #8377, #3775, #17304, #14068, #640, #9832, #13971, #15635, #9462, #8200, #736, #9747, #6631, #15545, #12598, #14167, #18589, #4966, #5156, #15825, #17024, #12401, #6715, #17114, #10924, #544, #9553, #2115, #8004, #17209, #3678, #2015, #12495, #18688, #16925, #5253, #18497, #15448, #2301, #5066, #11205, #8285, #14255, #827, #2392, #449, #3487, #8659, #7291, #1207, #7188, #8563, #5628, #10115, #11590, #10216, #5532, #2676, #7094, #1022, #4056, #5729, #13162, #17680, #19159, #14741, #18874, #3963, #16112, #16310, #17588, #11687, #14640, #2583, #8472, #4257, #2483, #4164, #16208, #17479, #14347, #2878, #13058, #10022, #2775, #1319, #8752, #18962, #14541, #1114, #4358, #14447, #13257, #16024, #19256, #9923, #19055 ),
 .UNSPECIFIED., .F., .F. ) 
 B_SPLINE_CURVE_WITH_KNOTS ( ( 3, 2, 2, 2, 2, 2, 2, 2, 2, 2, 2, 2, 2, 2, 2, 2, 2, 2, 2, 2, 2, 2, 2, 2, 2, 2, 2, 2, 2, 2, 2, 2, 2, 2, 2, 2, 2, 2, 2, 2, 2, 2, 2, 2, 2, 2, 2, 2, 2, 2, 2, 2, 2, 2, 2, 2, 2, 2, 2, 2, 2, 2, 2, 2, 2, 2, 2, 2, 2, 2, 2, 2, 2, 2, 2, 2, 2, 2, 2, 2, 2, 2, 2, 2, 2, 2, 2, 2, 2, 2, 2, 2, 2, 2, 2, 2, 3 ),
 ( 0.000000000000000000, 0.01041666666666666609, 0.02083333333333333218, 0.03125000000000000000, 0.04166666666666666435, 0.05208333333333333565, 0.06250000000000000000, 0.07291666666666667129, 0.08333333333333332871, 0.09375000000000000000, 0.1041666666666666713, 0.1145833333333333287, 0.1250000000000000000, 0.1354166666666666574, 0.1458333333333333426, 0.1562500000000000000, 0.1666666666666666574, 0.1770833333333333426, 0.1875000000000000000, 0.1979166666666666574, 0.2083333333333333426, 0.2187500000000000000, 0.2291666666666666574, 0.2395833333333333426, 0.2500000000000000000, 0.2604166666666666852, 0.2708333333333333148, 0.2812500000000000000, 0.2916666666666666852, 0.3020833333333333148, 0.3125000000000000000, 0.3229166666666666852, 0.3333333333333333148, 0.3437500000000000000, 0.3541666666666666852, 0.3645833333333333148, 0.3750000000000000000, 0.3854166666666666852, 0.3958333333333333148, 0.4062500000000000000, 0.4166666666666666852, 0.4270833333333333148, 0.4375000000000000000, 0.4479166666666666852, 0.4583333333333333148, 0.4687500000000000000, 0.4791666666666666852, 0.4895833333333333148, 0.5000000000000000000, 0.5104166666666666297, 0.5208333333333333703, 0.5312500000000000000, 0.5416666666666666297, 0.5520833333333333703, 0.5625000000000000000, 0.5729166666666666297, 0.5833333333333333703, 0.5937500000000000000, 0.6041666666666666297, 0.6145833333333333703, 0.6250000000000000000, 0.6354166666666666297, 0.6458333333333333703, 0.6562500000000000000, 0.6666666666666666297, 0.6770833333333333703, 0.6875000000000000000, 0.6979166666666666297, 0.7083333333333333703, 0.7187500000000000000, 0.7291666666666666297, 0.7395833333333333703, 0.7500000000000000000, 0.7604166666666666297, 0.7708333333333333703, 0.7812500000000000000, 0.7916666666666666297, 0.8020833333333333703, 0.8125000000000000000, 0.8229166666666666297, 0.8333333333333333703, 0.8437500000000000000, 0.8541666666666666297, 0.8645833333333333703, 0.8750000000000000000, 0.8854166666666666297, 0.8958333333333333703, 0.9062500000000000000, 0.9166666666666666297, 0.9270833333333333703, 0.9375000000000000000, 0.9479166666666666297, 0.9583333333333333703, 0.9687500000000000000, 0.9791666666666666297, 0.9895833333333333703, 1.000000000000000000 ),
 .UNSPECIFIED. ) 
 CURVE ( )  GEOMETRIC_REPRESENTATION_ITEM ( )  RATIONAL_B_SPLINE_CURVE ( ( 1.000000000000000000, 0.9659258262890683122, 1.000000000000000000, 0.9659258262890683122, 1.000000000000000000, 0.9659258262890683122, 1.000000000000000000, 0.9659258262890683122, 1.000000000000000000, 0.9659258262890683122, 1.000000000000000000, 0.9659258262890683122, 1.000000000000000000, 0.9659258262890683122, 1.000000000000000000, 0.9659258262890683122, 1.000000000000000000, 0.9659258262890683122, 1.000000000000000000, 0.9659258262890683122, 1.000000000000000000, 0.9659258262890683122, 1.000000000000000000, 0.9659258262890683122, 1.000000000000000000, 0.9659258262890683122, 1.000000000000000000, 0.9659258262890683122, 1.000000000000000000, 0.9659258262890683122, 1.000000000000000000, 0.9659258262890683122, 1.000000000000000000, 0.9659258262890683122, 1.000000000000000000, 0.9659258262890683122, 1.000000000000000000, 0.9659258262890683122, 1.000000000000000000, 0.9659258262890683122, 1.000000000000000000, 0.9659258262890683122, 1.000000000000000000, 0.9659258262890683122, 1.000000000000000000, 0.9659258262890683122, 1.000000000000000000, 0.9659258262890683122, 1.000000000000000000, 0.9659258262890683122, 1.000000000000000000, 0.9659258262890683122, 1.000000000000000000, 0.9659258262890683122, 1.000000000000000000, 0.9659258262890683122, 1.000000000000000000, 0.9659258262890683122, 1.000000000000000000, 0.9659258262890683122, 1.000000000000000000, 0.9659258262890683122, 1.000000000000000000, 0.9659258262890683122, 1.000000000000000000, 0.9659258262890683122, 1.000000000000000000, 0.9659258262890683122, 1.000000000000000000, 0.9659258262890683122, 1.000000000000000000, 0.9659258262890683122, 1.000000000000000000, 0.9659258262890683122, 1.000000000000000000, 0.9659258262890683122, 1.000000000000000000, 0.9659258262890683122, 1.000000000000000000, 0.9659258262890683122, 1.000000000000000000, 0.9659258262890683122, 1.000000000000000000, 0.9659258262890683122, 1.000000000000000000, 0.9659258262890683122, 1.000000000000000000, 0.9659258262890683122, 1.000000000000000000, 0.9659258262890683122, 1.000000000000000000, 0.9659258262890683122, 1.000000000000000000, 0.9659258262890683122, 1.000000000000000000, 0.9659258262890683122, 1.000000000000000000, 0.9659258262890683122, 1.000000000000000000, 0.9659258262890683122, 1.000000000000000000, 0.9659258262890683122, 1.000000000000000000, 0.9659258262890683122, 1.000000000000000000, 0.9659258262890683122, 1.000000000000000000, 0.9659258262890683122, 1.000000000000000000, 0.9659258262890683122, 1.000000000000000000, 0.9659258262890683122, 1.000000000000000000, 0.9659258262890683122, 1.000000000000000000, 0.9659258262890683122, 1.000000000000000000, 0.9659258262890683122, 1.000000000000000000, 0.9659258262890683122, 1.000000000000000000, 0.9659258262890683122, 1.000000000000000000, 0.9659258262890683122, 1.000000000000000000, 0.9659258262890683122, 1.000000000000000000, 0.9659258262890683122, 1.000000000000000000, 0.9659258262890683122, 1.000000000000000000, 0.9659258262890683122, 1.000000000000000000, 0.9659258262890683122, 1.000000000000000000, 0.9659258262890683122, 1.000000000000000000, 0.9659258262890683122, 1.000000000000000000, 0.9659258262890683122, 1.000000000000000000, 0.9659258262890683122, 1.000000000000000000, 0.9659258262890683122, 1.000000000000000000, 0.9659258262890683122, 1.000000000000000000, 0.9659258262890683122, 1.000000000000000000, 0.9659258262890683122, 1.000000000000000000, 0.9659258262890683122, 1.000000000000000000, 0.9659258262890683122, 1.000000000000000000, 0.9659258262890683122, 1.000000000000000000, 0.9659258262890683122, 1.000000000000000000, 0.9659258262890683122, 1.000000000000000000, 0.9659258262890683122, 1.000000000000000000, 0.9659258262890683122, 1.000000000000000000, 0.9659258262890683122, 1.000000000000000000, 0.9659258262890683122, 1.000000000000000000, 0.9659258262890683122, 1.000000000000000000, 0.9659258262890683122, 1.000000000000000000, 0.9659258262890683122, 1.000000000000000000, 0.9659258262890683122, 1.000000000000000000, 0.9659258262890683122, 1.000000000000000000, 0.9659258262890683122, 1.000000000000000000, 0.9659258262890683122, 1.000000000000000000, 0.9659258262890683122, 1.000000000000000000, 0.9659258262890683122, 1.000000000000000000, 0.9659258262890683122, 1.000000000000000000, 0.9659258262890683122, 1.000000000000000000, 0.9659258262890683122, 1.000000000000000000 ) ) 
 REPRESENTATION_ITEM ( '' )  );
#18287=B_SPLINE_CURVE_WITH_KNOTS ( 'NONE', 3,
 ( #11980, #13251, #16401, #8746, #7285, #13647, #16504, #11882, #10307, #19250, #13550, #5818, #10407, #129, #16302, #2872, #13354, #4650, #1509, #14835, #6115, #3067, #9046, #4454 ),
 .UNSPECIFIED., .F., .F.,
 ( 4, 2, 2, 2, 2, 2, 2, 2, 2, 2, 2, 4 ),
 ( 0.005317382883715828651, 0.005430869497434138646, 0.005544356111152449508, 0.005771329338589079039, 0.006225275793462339835, 0.007133168703208861428, 0.008041061612955383020, 0.008948954522701904613, 0.009856847432448426205, 0.01076474034219494780, 0.01167263325194146766, 0.01258052616168798925 ),
 .UNSPECIFIED. ) ;
#18293=CARTESIAN_POINT ( 'NONE',  ( -17.64274437364855430, -28.24771351637087236, 12.57617750791695777 ) ) ;
#18295=CARTESIAN_POINT ( 'NONE',  ( -17.64274437364858983, -19.75228648362910633, 16.29882249208304046 ) ) ;
#18297=CARTESIAN_POINT ( 'NONE',  ( -16.50457296725820555, -28.95583473709189448, 12.35742750791695954 ) ) ;
#18299=CARTESIAN_POINT ( 'NONE',  ( -10.04416526290807710, -25.50457296725819489, 16.29492750791695954 ) ) ;
#18309=MECHANICAL_DESIGN_GEOMETRIC_PRESENTATION_REPRESENTATION('',(#4520),#16092);
#18312=CARTESIAN_POINT ( 'NONE',  ( -9.996306089212408708, -18.75498260482328661, 27.89257249208303691 ) ) ;
#18314=CARTESIAN_POINT ( 'NONE',  ( -18.78091578003892792, -20.46040770435013556, 5.580072492083041347 ) ) ;
#18316=CARTESIAN_POINT ( 'NONE',  ( -12.48433729119798130, -25.64274437364855075, 27.01367750791695954 ) ) ;
#18318=CARTESIAN_POINT ( 'NONE',  ( -20.97976432393974022, -27.64274437364858628, 20.23632249208303691 ) ) ;
#18336=CARTESIAN_POINT ( 'NONE',  ( -11.64274437364854187, -30.14459132904234195, 32.70117750791695244 ) ) ;
#18341=CARTESIAN_POINT ( 'NONE',  ( -14.83517299489736985, -26.99999999999998579, 19.36132249208304046 ) ) ;
#18342=CARTESIAN_POINT ( 'NONE',  ( -11.35725562635144925, -18.02023567606020293, 15.20117750791695599 ) ) ;
#18346=CARTESIAN_POINT ( 'NONE',  ( -17.51566270880201159, -22.35725562635141728, 13.88867750791695954 ) ) ;
#18366=CARTESIAN_POINT ( 'NONE',  ( -11.46040770435012668, -27.78091578003887463, 32.48242750791695954 ) ) ;
#18370=CARTESIAN_POINT ( 'NONE',  ( -13.49542703274174116, -28.95583473709188738, 13.89257249208303691 ) ) ;
#18374=CARTESIAN_POINT ( 'NONE',  ( -17.51566270880199738, -25.64274437364856496, 20.23632249208304401 ) ) ;
#18389=CARTESIAN_POINT ( 'NONE',  ( -19.95583473709191580, -22.49542703274176603, 13.66992750791695599 ) ) ;
#18391=CARTESIAN_POINT ( 'NONE',  ( -19.24771351637086880, -26.64274437364857206, 14.98632249208304046 ) ) ;
#18396=CARTESIAN_POINT ( 'NONE',  ( -10.04416526290807710, -25.50457296725819489, 16.29492750791695954 ) ) ;
#18399=CARTESIAN_POINT ( 'NONE',  ( -16.50457296725820555, -28.95583473709189803, 12.35742750791695777 ) ) ;
#18401=CARTESIAN_POINT ( 'NONE',  ( -11.21908421996106142, -27.53959229564982181, 18.70507249208304401 ) ) ;
#18410=CARTESIAN_POINT ( 'NONE',  ( -7.955834737091903364, -25.71081734191518464, 34.01757249208303335 ) ) ;
#18412=CARTESIAN_POINT ( 'NONE',  ( -17.35725562635140307, -28.41254052147349185, 14.54882249208304046 ) ) ;
#18415=CARTESIAN_POINT ( 'NONE',  ( -17.99999999999999645, -23.83517299489736985, 34.45117750791695954 ) ) ;
#18418=CARTESIAN_POINT ( 'NONE',  ( -21.99999999999999289, -24.16482700510262305, 25.92382249208304046 ) ) ;
#18433=CARTESIAN_POINT ( 'NONE',  ( -14.83517299489740715, -16.99999999999997868, 35.76367750791694533 ) ) ;
#18437=CARTESIAN_POINT ( 'NONE',  ( -12.68318583509882380, -26.07549068051207541, 29.20507249208304756 ) ) ;
#18438=CARTESIAN_POINT ( 'NONE',  ( -8.855408670957631401, -20.64274437364852943, 20.88867750791695954 ) ) ;
#18443=CARTESIAN_POINT ( 'NONE',  ( -11.95583473709191047, -23.36097942780921954, 36.85742750791697375 ) ) ;
#18459=CARTESIAN_POINT ( 'NONE',  ( -9.955834737091912245, -22.82508104294696594, 31.60742750791695954 ) ) ;
#18464=CARTESIAN_POINT ( 'NONE',  ( -20.04416526290809131, -22.82508104294699791, 36.64257249208304046 ) ) ;
#18466=CARTESIAN_POINT ( 'NONE',  ( -12.48433729119799196, -22.35725562635139596, 12.36132249208304401 ) ) ;
#18485=CARTESIAN_POINT ( 'NONE',  ( -12.64274437364855252, -28.41254052147347053, 22.20117750791695599 ) ) ;
#18489=CARTESIAN_POINT ( 'NONE',  ( -14.83517299489735741, -28.99999999999998224, 14.11132249208304046 ) ) ;
#18492=CARTESIAN_POINT ( 'NONE',  ( -12.35725562635143682, -19.75228648362908501, 20.45117750791695954 ) ) ;
#18494=CARTESIAN_POINT ( 'NONE',  ( -13.49542703274178201, -19.04416526290806289, 30.73242750791695954 ) ) ;
#18497=CARTESIAN_POINT ( 'NONE',  ( -14.83517299489735741, -28.99999999999998224, 29.86132249208304401 ) ) ;
#18509=CARTESIAN_POINT ( 'NONE',  ( -11.35725562635139418, -29.97976432393972601, 34.67382249208304046 ) ) ;
#18511=CARTESIAN_POINT ( 'NONE',  ( -11.21908421996106142, -27.53959229564982181, 13.45507249208304223 ) ) ;
#18513=CARTESIAN_POINT ( 'NONE',  ( -12.31951028609537602, -22.64274437364854364, 31.38867750791696309 ) ) ;
#18515=CARTESIAN_POINT ( 'NONE',  ( -9.754982604823302594, -29.00369391078756465, 18.70507249208304046 ) ) ;
#18534=CARTESIAN_POINT ( 'NONE',  ( -21.95583473709191580, -21.95952864787954084, 29.41992750791695954 ) ) ;
#18538=CARTESIAN_POINT ( 'NONE',  ( -17.31681416490117087, -21.92450931948788551, 31.83007249208304046 ) ) ;
#18540=CARTESIAN_POINT ( 'NONE',  ( -21.99999999999999289, -23.83517299489739116, 23.95117750791696309 ) ) ;
#18546=CARTESIAN_POINT ( 'NONE',  ( -17.07549068051210739, -21.68318583509881847, 24.60742750791696309 ) ) ;
#18550=VERTEX_POINT ( 'NONE', #8643 ) ;
#18563=CARTESIAN_POINT ( 'NONE',  ( -19.24771351637089367, -21.35725562635142438, 34.88867750791696665 ) ) ;
#18566=CARTESIAN_POINT ( 'NONE',  ( -17.35725562635140307, -28.41254052147349185, 25.04882249208304401 ) ) ;
#18568=CARTESIAN_POINT ( 'NONE',  ( -13.64274437364857739, -21.31951028609534760, 32.92382249208304046 ) ) ;
#18581=CARTESIAN_POINT ( 'NONE',  ( -17.35725562635144215, -19.58745947852648683, 24.82617750791695954 ) ) ;
#18583=CARTESIAN_POINT ( 'NONE',  ( -10.75228648362912232, -21.35725562635138530, 28.11132249208304046 ) ) ;
#18585=CARTESIAN_POINT ( 'NONE',  ( -17.64274437364855430, -28.24771351637087236, 17.82617750791695599 ) ) ;
#18587=CARTESIAN_POINT ( 'NONE',  ( -13.82508104294698015, -29.04416526290806289, 32.91992750791695954 ) ) ;
#18589=CARTESIAN_POINT ( 'NONE',  ( -19.24771351637086880, -26.64274437364857206, 25.48632249208304401 ) ) ;
#18599=CARTESIAN_POINT ( 'NONE',  ( -22.04416526290809486, -22.28918265808477628, 31.39257249208304401 ) ) ;
#18603=CARTESIAN_POINT ( 'NONE',  ( -13.35725562635142794, -21.48433729119796709, 25.70117750791695954 ) ) ;
#18606=CARTESIAN_POINT ( 'NONE',  ( -21.95583473709189803, -26.04047135212049469, 20.45507249208304046 ) ) ;
#18622=CARTESIAN_POINT ( 'NONE',  ( -20.97976432393977575, -20.35725562635143504, 34.88867750791695954 ) ) ;
#18627=CARTESIAN_POINT ( 'NONE',  ( -17.51566270880199738, -25.64274437364856496, 30.73632249208304401 ) ) ;
#18628=CARTESIAN_POINT ( 'NONE',  ( -21.14459132904236327, -27.35725562635143149, 13.01367750791695777 ) ) ;
#18634=CARTESIAN_POINT ( 'NONE',  ( -11.95583473709191047, -23.36097942780921954, 26.35742750791696309 ) ) ;
#18655=CARTESIAN_POINT ( 'NONE',  ( -19.95583473709191580, -22.49542703274176603, 24.16992750791694888 ) ) ;
#18658=CARTESIAN_POINT ( 'NONE',  ( -13.82508104294702100, -18.95583473709188382, 27.45507249208304046 ) ) ;
#18661=CARTESIAN_POINT ( 'NONE',  ( -12.92450931948790149, -21.68318583509881137, 27.89257249208304401 ) ) ;
#18678=CARTESIAN_POINT ( 'NONE',  ( -20.04416526290808065, -25.17491895705300209, 34.23242750791695954 ) ) ;
#18681=CARTESIAN_POINT ( 'NONE',  ( -17.35725562635140307, -28.41254052147349185, 30.29882249208304401 ) ) ;
#18683=CARTESIAN_POINT ( 'NONE',  ( -10.04416526290807710, -25.50457296725819489, 32.04492750791695954 ) ) ;
#18686=CARTESIAN_POINT ( 'NONE',  ( -12.35725562635143682, -19.75228648362908501, 36.20117750791695954 ) ) ;
#18688=CARTESIAN_POINT ( 'NONE',  ( -11.21908421996106142, -27.53959229564982181, 29.20507249208304046 ) ) ;
#18699=CARTESIAN_POINT ( 'NONE',  ( -16.64274437364856496, -26.51566270880199738, 28.32617750791696665 ) ) ;
#18701=CARTESIAN_POINT ( 'NONE',  ( -20.97976432393974022, -27.64274437364858628, 30.73632249208304046 ) ) ;
#18713=CARTESIAN_POINT ( 'NONE',  ( -17.04047135212043784, -30.95583473709190159, 33.35742750791695244 ) ) ;
#18717=CARTESIAN_POINT ( 'NONE',  ( -12.92450931948790149, -21.68318583509881137, 33.14257249208304756 ) ) ;
#18718=CARTESIAN_POINT ( 'NONE',  ( -21.95583473709191580, -21.95952864787954084, 34.66992750791696665 ) ) ;
#18723=CARTESIAN_POINT ( 'NONE',  ( -17.51566270880201159, -22.35725562635141728, 24.38867750791696665 ) ) ;
#18740=CARTESIAN_POINT ( 'NONE',  ( -9.955834737091912245, -22.82508104294696594, 36.85742750791696665 ) ) ;
#18745=CARTESIAN_POINT ( 'NONE',  ( -9.955834737091903364, -25.17491895705294880, 34.01757249208303335 ) ) ;
#18748=CARTESIAN_POINT ( 'NONE',  ( -14.36097942780925685, -20.95583473709189093, 37.95507249208304046 ) ) ;
#18762=CARTESIAN_POINT ( 'NONE',  ( -9.999999999999994671, -24.16482700510257686, 26.57617750791695954 ) ) ;
#18764=CARTESIAN_POINT ( 'NONE',  ( -10.04416526290808953, -22.49542703274172695, 38.83007249208302625 ) ) ;
#18766=CARTESIAN_POINT ( 'NONE',  ( -20.04416526290808065, -25.17491895705300209, 28.98242750791695244 ) ) ;
#18769=CARTESIAN_POINT ( 'NONE',  ( -20.04416526290808065, -25.17491895705300209, 39.48242750791695244 ) ) ;
#18771=CARTESIAN_POINT ( 'NONE',  ( -18.53959229564983247, -27.78091578003891016, 20.01757249208304046 ) ) ;
#18783=CARTESIAN_POINT ( 'NONE',  ( -13.49542703274178379, -19.04416526290806289, -0.7675724920830416798 ) ) ;
#18786=CARTESIAN_POINT ( 'NONE',  ( -12.95952864787948755, -30.95583473709188382, 40.14257249208304756 ) ) ;
#18803=CARTESIAN_POINT ( 'NONE',  ( -9.996306089212408708, -18.75498260482328661, 6.892572492083038682 ) ) ;
#18808=PRODUCT ( 'spring', 'spring', '', ( #5899 ) ) ;
#18809=CARTESIAN_POINT ( 'NONE',  ( -18.04416526290808775, -23.36097942780924441, 26.14257249208303691 ) ) ;
#18810=CARTESIAN_POINT ( 'NONE',  ( -9.754982604823348780, -18.99630608921234654, 31.16992750791695954 ) ) ;
#18833=CARTESIAN_POINT ( 'NONE',  ( -7.999999999999996447, -24.16482700510256976, 5.576177507916956877 ) ) ;
#18838=CARTESIAN_POINT ( 'NONE',  ( -12.35725562635140307, -28.24771351637085459, 34.67382249208304046 ) ) ;
#18843=CARTESIAN_POINT ( 'NONE',  ( -11.95583473709190514, -24.63902057219072361, 34.01757249208304046 ) ) ;
#18856=CARTESIAN_POINT ( 'NONE',  ( -10.04416526290807710, -25.50457296725819489, 32.04492750791695954 ) ) ;
#18865=CARTESIAN_POINT ( 'NONE',  ( -16.17491895705301275, -18.95583473709189803, 35.54492750791695954 ) ) ;
#18867=CARTESIAN_POINT ( 'NONE',  ( -10.58745947852648328, -26.35725562635138530, 34.23632249208304046 ) ) ;
#18870=CARTESIAN_POINT ( 'NONE',  ( -19.41254052147348830, -26.35725562635142083, 34.01367750791696665 ) ) ;
#18872=CARTESIAN_POINT ( 'NONE',  ( -16.17491895705301275, -18.95583473709189448, 30.29492750791695954 ) ) ;
#18873=DIRECTION ( 'NONE',  ( 0.9863224920830413467, 5.275954983314436132E-15, 0.1648270051026190230 ) ) ;
#18874=CARTESIAN_POINT ( 'NONE',  ( -19.99999999999999645, -24.16482700510261949, 36.42382249208304046 ) ) ;
#18884=ORIENTED_EDGE ( 'NONE', *, *, #16077, .F. ) ;
#18886=CARTESIAN_POINT ( 'NONE',  ( -10.75228648362910100, -26.64274437364854009, 0.7636775079169582092 ) ) ;
#18888=CARTESIAN_POINT ( 'NONE',  ( -12.95952864787948755, -30.95583473709188382, 34.89257249208303335 ) ) ;
#18900=CARTESIAN_POINT ( 'NONE',  ( -11.64274437364854187, -30.14459132904234195, 37.95117750791695244 ) ) ;
#18903=ORIENTED_EDGE ( 'NONE', *, *, #2641, .F. ) ;
#18904=CARTESIAN_POINT ( 'NONE',  ( -11.95583473709191047, -23.36097942780921954, 5.357427507916959541 ) ) ;
#18905=CARTESIAN_POINT ( 'NONE',  ( -13.28918265808472299, -31.04416526290805933, 32.91992750791695244 ) ) ;
#18923=CARTESIAN_POINT ( 'NONE',  ( -17.35725562635144215, -19.58745947852648683, 40.57617750791696665 ) ) ;
#18927=CARTESIAN_POINT ( 'NONE',  ( -13.35725562635141195, -26.51566270880198672, 8.423822492083042235 ) ) ;
#18930=CARTESIAN_POINT ( 'NONE',  ( -17.07549068051208963, -26.31681416490115311, 35.76757249208304756 ) ) ;
#18942=CARTESIAN_POINT ( 'NONE',  ( -10.04416526290807710, -25.50457296725819489, 21.54492750791695599 ) ) ;
#18945=CARTESIAN_POINT ( 'NONE',  ( -11.46040770435012668, -27.78091578003887463, 0.9824275079169582092 ) ) ;
#18949=CARTESIAN_POINT ( 'NONE',  ( -19.95583473709190514, -25.50457296725822687, 4.705072492083039570 ) ) ;
#18951=CARTESIAN_POINT ( 'NONE',  ( -10.04416526290807710, -25.50457296725819489, 37.29492750791697375 ) ) ;
#18953=CARTESIAN_POINT ( 'NONE',  ( -13.82508104294702100, -18.95583473709188382, 32.70507249208304046 ) ) ;
#18957=CARTESIAN_POINT ( 'NONE',  ( -16.50457296725820555, -28.95583473709189448, 28.10742750791695954 ) ) ;
#18960=CARTESIAN_POINT ( 'NONE',  ( -18.53959229564986799, -20.21908421996107563, 40.35742750791695954 ) ) ;
#18962=CARTESIAN_POINT ( 'NONE',  ( -18.53959229564983247, -27.78091578003891016, 41.01757249208303335 ) ) ;
#18975=CARTESIAN_POINT ( 'NONE',  ( -12.64274437364855252, -28.41254052147347053, 6.451177507916959541 ) ) ;
#18978=CARTESIAN_POINT ( 'NONE',  ( -13.28918265808478694, -16.95583473709189093, 37.95507249208304046 ) ) ;
#18995=CARTESIAN_POINT ( 'NONE',  ( -20.00369391078762860, -18.75498260482333279, 40.35742750791695954 ) ) ;
#19000=CARTESIAN_POINT ( 'NONE',  ( -14.83517299489736985, -26.99999999999998579, 40.36132249208304756 ) ) ;
#19001=CARTESIAN_POINT ( 'NONE',  ( -7.955834737091916686, -22.28918265808470522, 31.60742750791695244 ) ) ;
#19022=CARTESIAN_POINT ( 'NONE',  ( -15.16482700510259640, -28.99999999999998224, 38.38867750791695954 ) ) ;
#19025=CARTESIAN_POINT ( 'NONE',  ( -18.04416526290808775, -23.36097942780924441, 10.39257249208304223 ) ) ;
#19028=CARTESIAN_POINT ( 'NONE',  ( -13.35725562635142794, -21.48433729119796709, 4.701177507916959541 ) ) ;
#19037=CARTESIAN_POINT ( 'NONE',  ( -19.99999999999999645, -23.83517299489738051, 29.20117750791695599 ) ) ;
#19043=CARTESIAN_POINT ( 'NONE',  ( -18.53959229564982536, -27.78091578003890660, 9.517572492083042235 ) ) ;
#19044=CARTESIAN_POINT ( 'NONE',  ( -15.16482700510258574, -30.99999999999998224, 1.638677507916956433 ) ) ;
#19046=CARTESIAN_POINT ( 'NONE',  ( -16.35725562635141372, -26.68048971390461332, 9.298822492083044011 ) ) ;
#19051=CARTESIAN_POINT ( 'NONE',  ( -11.21908421996108629, -20.46040770435011069, 36.41992750791695954 ) ) ;
#19055=CARTESIAN_POINT ( 'NONE',  ( -15.16482700510263371, -18.99999999999997868, 42.98632249208304046 ) ) ;
#19062=AXIS2_PLACEMENT_3D ( 'NONE', #8471, #18873, #5627 ) ;
#19066=CARTESIAN_POINT ( 'NONE',  ( -10.58745947852649927, -21.64274437364853654, 5.138677507916957765 ) ) ;
#19067=CARTESIAN_POINT ( 'NONE',  ( -18.78091578003889950, -27.53959229564985378, 7.544927507916956877 ) ) ;
#19069=CARTESIAN_POINT ( 'NONE',  ( -20.00369391078757886, -29.24501739517668142, 35.76757249208303335 ) ) ;
#19072=CARTESIAN_POINT ( 'NONE',  ( -18.04416526290808420, -24.63902057219074493, 28.98242750791696309 ) ) ;
#19089=CARTESIAN_POINT ( 'NONE',  ( -21.14459132904239169, -20.64274437364858628, 10.61132249208303868 ) ) ;
#19094=CARTESIAN_POINT ( 'NONE',  ( -16.35725562635141372, -26.68048971390461332, 40.79882249208304756 ) ) ;
#19095=CARTESIAN_POINT ( 'NONE',  ( -9.754982604823348780, -18.99630608921234654, 36.41992750791695954 ) ) ;
#19118=CARTESIAN_POINT ( 'NONE',  ( -21.14459132904236327, -27.35725562635143149, 2.513677507916956433 ) ) ;
#19122=CARTESIAN_POINT ( 'NONE',  ( -12.68318583509882380, -26.07549068051207541, 8.205072492083042235 ) ) ;
#19126=CARTESIAN_POINT ( 'NONE',  ( -14.03132541760401786, -21.04416526290806289, 4.482427507916961318 ) ) ;
#19139=CARTESIAN_POINT ( 'NONE',  ( -13.82508104294698192, -29.04416526290806644, 22.41992750791695244 ) ) ;
#19141=CARTESIAN_POINT ( 'NONE',  ( -15.16482700510263371, -18.99999999999997868, 0.9863224920830410136 ) ) ;
#19145=CARTESIAN_POINT ( 'NONE',  ( -10.58745947852648328, -26.35725562635138530, 2.736322492083041347 ) ) ;
#19148=CARTESIAN_POINT ( 'NONE',  ( -8.855408670957631401, -20.64274437364852943, -0.1113224920830435533 ) ) ;
#19150=CARTESIAN_POINT ( 'NONE',  ( -15.96867458239599635, -21.04416526290806999, 6.017572492083043123 ) ) ;
#19159=CARTESIAN_POINT ( 'NONE',  ( -19.24771351637086880, -26.64274437364857206, 35.98632249208304046 ) ) ;
#19167=CARTESIAN_POINT ( 'NONE',  ( -18.78091578003889950, -27.53959229564985378, 7.544927507916956877 ) ) ;
#19168=CARTESIAN_POINT ( 'NONE',  ( -18.78091578003889950, -27.53959229564985378, 2.294927507916958209 ) ) ;
#19170=CARTESIAN_POINT ( 'NONE',  ( -16.50457296725825174, -19.04416526290807354, 11.26757249208304046 ) ) ;
#19172=CARTESIAN_POINT ( 'NONE',  ( -19.99999999999999645, -23.83517299489738051, 2.951177507916958209 ) ) ;
#19173=CARTESIAN_POINT ( 'NONE',  ( -17.64274437364855430, -28.24771351637087236, 7.326177507916957765 ) ) ;
#19187=CARTESIAN_POINT ( 'NONE',  ( -20.24501739517669563, -18.99630608921239627, 10.83007249208304046 ) ) ;
#19189=CARTESIAN_POINT ( 'NONE',  ( -12.35725562635140307, -28.24771351637085459, 3.173822492083041347 ) ) ;
#19192=CARTESIAN_POINT ( 'NONE',  ( -12.92450931948788906, -26.31681416490114245, 0.9824275079169599856 ) ) ;
#19193=CARTESIAN_POINT ( 'NONE',  ( -8.044165262908093084, -21.95952864787946979, 7.330072492083040459 ) ) ;
#19213=CARTESIAN_POINT ( 'NONE',  ( -20.00369391078762860, -18.75498260482333279, 3.607427507916956433 ) ) ;
#19217=CARTESIAN_POINT ( 'NONE',  ( -17.68048971390462754, -22.64274437364856496, 5.361322492083044011 ) ) ;
#19219=ADVANCED_FACE ( 'NONE', ( #2936 ), #1571, .T. ) ;
#19223=CARTESIAN_POINT ( 'NONE',  ( -17.07549068051210739, -21.68318583509881847, 3.607427507916959097 ) ) ;
#19234=CARTESIAN_POINT ( 'NONE',  ( -18.53959229564986799, -20.21908421996107563, 24.60742750791695954 ) ) ;
#19237=CARTESIAN_POINT ( 'NONE',  ( -17.35725562635144215, -19.58745947852648683, 3.826177507916958209 ) ) ;
#19241=CARTESIAN_POINT ( 'NONE',  ( -9.999999999999994671, -23.83517299489734143, 2.298822492083040903 ) ) ;
#19243=CARTESIAN_POINT ( 'NONE',  ( -20.24501739517664234, -29.00369391078761439, 7.544927507916956877 ) ) ;
#19245=CARTESIAN_POINT ( 'NONE',  ( -17.31681416490117087, -21.92450931948788551, 5.580072492083043123 ) ) ;
#19250=CARTESIAN_POINT ( 'NONE',  ( -10.26208722734517842, -21.10617379198820487, 6.318196777486344053E-14 ) ) ;
#19256=CARTESIAN_POINT ( 'NONE',  ( -17.64274437364858983, -19.75228648362910633, 42.54882249208304046 ) ) ;
#19266=CARTESIAN_POINT ( 'NONE',  ( -18.53959229564986799, -20.21908421996107563, 3.607427507916956877 ) ) ;
#19267=CARTESIAN_POINT ( 'NONE',  ( -19.41254052147348830, -26.35725562635142083, 13.01367750791695777 ) ) ;
#19269=CARTESIAN_POINT ( 'NONE',  ( -21.14459132904239169, -20.64274437364858628, 42.11132249208304046 ) ) ;
#19271=CARTESIAN_POINT ( 'NONE',  ( -14.83517299489738761, -20.99999999999997513, 41.01367750791695954 ) ) ;
#19284=CARTESIAN_POINT ( 'NONE',  ( -15.16482700510264436, -16.99999999999997868, 16.73632249208304046 ) ) ;
#19291=CARTESIAN_POINT ( 'NONE',  ( -12.92450931948788906, -26.31681416490114245, 16.73242750791696309 ) ) ;
#19293=CARTESIAN_POINT ( 'NONE',  ( -15.16482700510264436, -16.99999999999997868, 11.48632249208304046 ) ) ;
#19313=CARTESIAN_POINT ( 'NONE',  ( -13.28918265808472299, -31.04416526290805933, 17.16992750791696309 ) ) ;
#19317=CARTESIAN_POINT ( 'NONE',  ( -15.16482700510262482, -20.99999999999997513, 0.9863224920830429010 ) ) ;
#19323=CARTESIAN_POINT ( 'NONE',  ( -15.16482700510260706, -26.99999999999998579, 6.888677507916960430 ) ) ;
#19338=CARTESIAN_POINT ( 'NONE',  ( -10.75228648362910100, -26.64274437364854009, 6.013677507916958653 ) ) ;
#19341=CARTESIAN_POINT ( 'NONE',  ( -17.64274437364858983, -19.75228648362910633, 5.798822492083041347 ) ) ;
#19342=CARTESIAN_POINT ( 'NONE',  ( -14.83517299489740715, -16.99999999999997868, 4.263677507916957765 ) ) ;
#19344=CARTESIAN_POINT ( 'NONE',  ( -15.16482700510262482, -20.99999999999997513, 6.236322492083043123 ) ) ;
#19349=CARTESIAN_POINT ( 'NONE',  ( -18.53959229564986799, -20.21908421996107563, 40.35742750791696665 ) ) ;
#19361=CARTESIAN_POINT ( 'NONE',  ( -17.64274437364855430, -28.24771351637087236, 2.076177507916958209 ) ) ;
#19362=CARTESIAN_POINT ( 'NONE',  ( -20.04416526290808065, -25.17491895705300209, 18.48242750791695954 ) ) ;
#19364=CARTESIAN_POINT ( 'NONE',  ( -14.83517299489734853, -30.99999999999998224, 40.36132249208304046 ) ) ;
#19366=CARTESIAN_POINT ( 'NONE',  ( -18.78091578003889950, -27.53959229564985378, 7.544927507916956877 ) ) ;
#19368=CARTESIAN_POINT ( 'NONE',  ( -20.04416526290808065, -25.17491895705300209, 7.982427507916958653 ) ) ;
#19381=CARTESIAN_POINT ( 'NONE',  ( -20.24501739517669563, -18.99630608921239627, 16.08007249208304046 ) ) ;
#19385=ORIENTED_EDGE ( 'NONE', *, *, #5333, .T. ) ;
#19386=CARTESIAN_POINT ( 'NONE',  ( -12.04416526290807887, -24.96867458239596260, 21.54492750791695954 ) ) ;
#19388=CARTESIAN_POINT ( 'NONE',  ( -20.97976432393974022, -27.64274437364858628, 9.736322492083036906 ) ) ;
ENDSEC;
END-ISO-10303-21;
